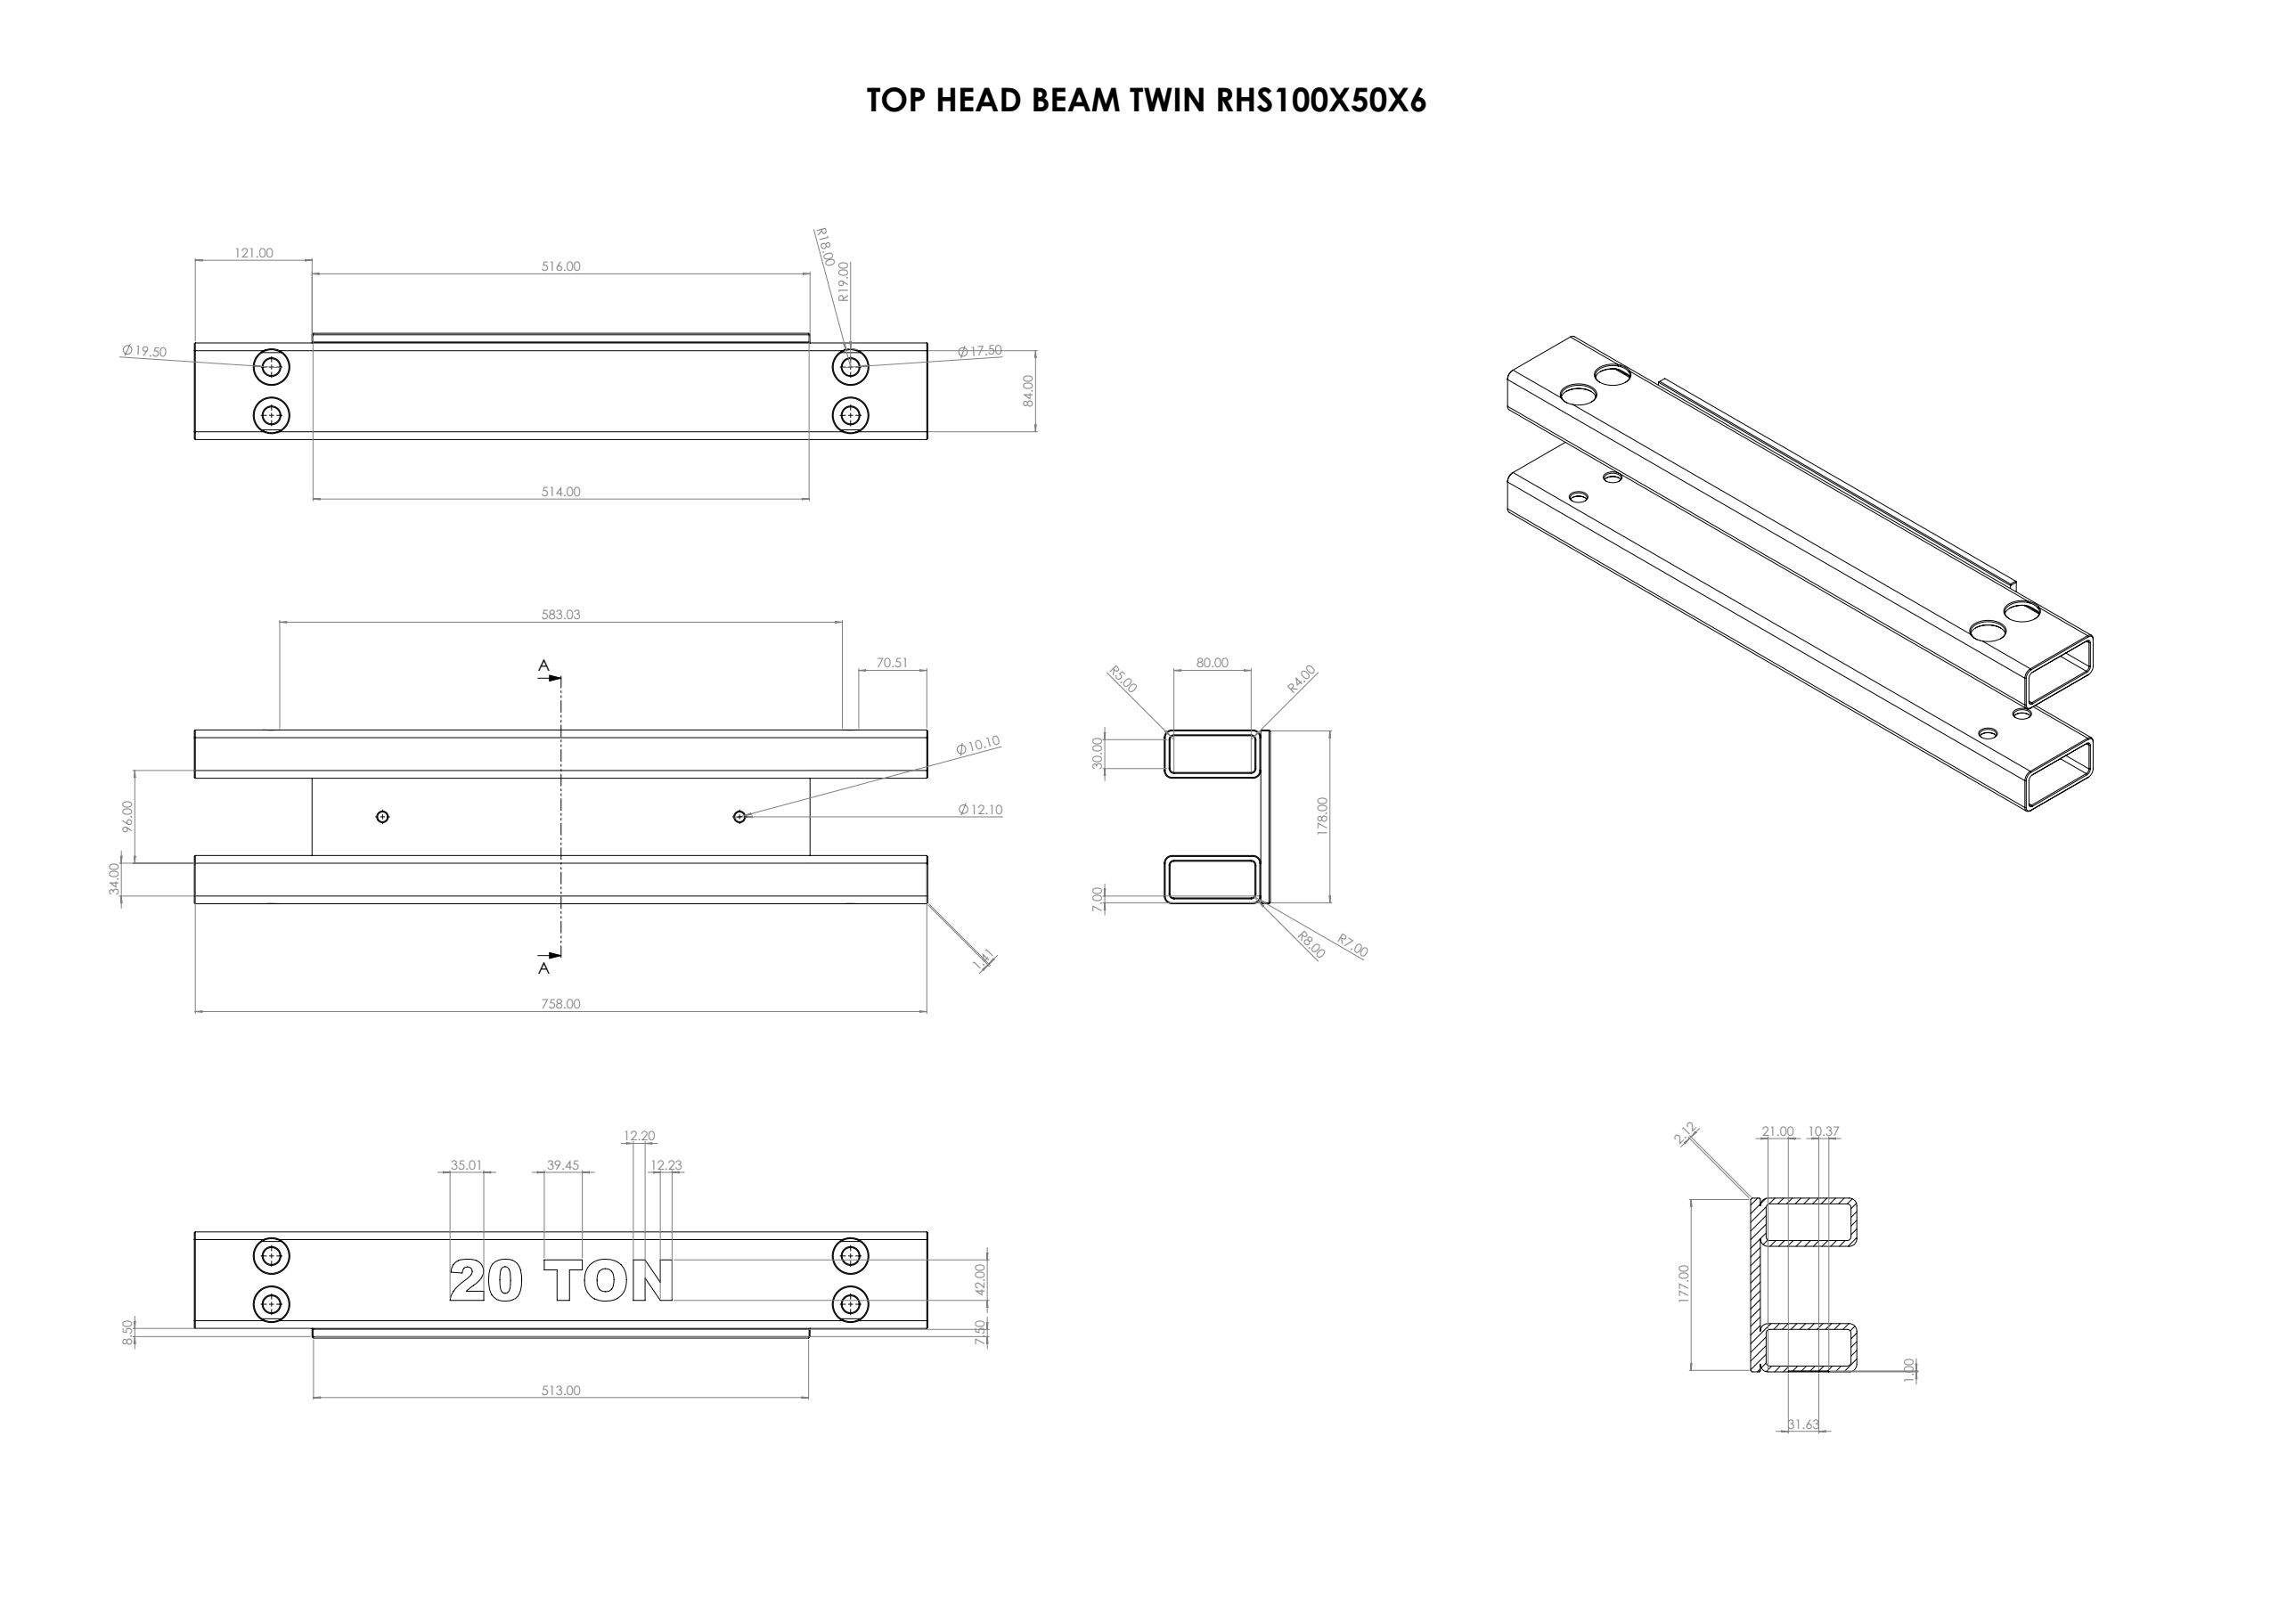
ISO-10303-21;
HEADER;
/* Generated by software containing ST-Developer
 * from STEP Tools, Inc. (www.steptools.com) 
 */

FILE_DESCRIPTION(
/* description */ (''),
/* implementation_level */ '2;1');

FILE_NAME(
/* name */ '02_Top_Head_Beam_Twin_RHS100x50x6.step',
/* time_stamp */ '2026-10-20T10:03:03-07:00',
/* author */ (''),
/* organization */ (''),
/* preprocessor_version */ 'ST-DEVELOPER v20.2',
/* originating_system */ 'Autodesk Translation Framework v15.15.0.0',
/* authorisation */ '');

FILE_SCHEMA (('AUTOMOTIVE_DESIGN { 1 0 10303 214 3 1 1 }'));
ENDSEC;

DATA;
#10=MECHANICAL_DESIGN_GEOMETRIC_PRESENTATION_REPRESENTATION('',(#439,#440,#441,#442,#443,#444,#445,#446,#447,#448,#449,#450,#451,#452,#453,#454,#455,#456,#457,#458,#459,#460,#461,#462,#463,#464,#465,#466,#467,#468,#469,#470,#471,#472,#473,#474,#475,#476,#477,#478,#479,#480,#481,#482,#483,#484,#485,#486,#487,#488,#489,#490,#491,#492,#493,#494,#495,#496,#497,#498,#499,#500,#501,#502,#503,#504,#505,#506,#507,#508,#509,#510,#511,#512,#513,#514,#515,#516,#517,#518,#519,#520,#521,#522,#523,#524),#71492);
#382=SHAPE_REPRESENTATION_RELATIONSHIP('SRR','None',#71603,#401);
#401=ADVANCED_BREP_SHAPE_REPRESENTATION('',(#420),#71473);
#420=MANIFOLD_SOLID_BREP('Top beam',#28459);
#439=STYLED_ITEM('',(#71873),#27095);
#440=STYLED_ITEM('',(#71873),#27096);
#441=STYLED_ITEM('',(#71873),#27097);
#442=STYLED_ITEM('',(#71873),#27098);
#443=STYLED_ITEM('',(#71873),#27099);
#444=STYLED_ITEM('',(#71873),#27100);
#445=STYLED_ITEM('',(#71873),#27101);
#446=STYLED_ITEM('',(#71873),#27102);
#447=STYLED_ITEM('',(#71873),#27103);
#448=STYLED_ITEM('',(#71873),#27104);
#449=STYLED_ITEM('',(#71873),#27105);
#450=STYLED_ITEM('',(#71873),#27106);
#451=STYLED_ITEM('',(#71873),#27107);
#452=STYLED_ITEM('',(#71873),#27108);
#453=STYLED_ITEM('',(#71873),#27109);
#454=STYLED_ITEM('',(#71873),#27110);
#455=STYLED_ITEM('',(#71873),#27111);
#456=STYLED_ITEM('',(#71873),#27112);
#457=STYLED_ITEM('',(#71873),#27113);
#458=STYLED_ITEM('',(#71873),#27114);
#459=STYLED_ITEM('',(#71873),#27115);
#460=STYLED_ITEM('',(#71873),#27116);
#461=STYLED_ITEM('',(#71873),#27117);
#462=STYLED_ITEM('',(#71873),#27118);
#463=STYLED_ITEM('',(#71873),#27119);
#464=STYLED_ITEM('',(#71873),#27120);
#465=STYLED_ITEM('',(#71873),#27121);
#466=STYLED_ITEM('',(#71873),#27122);
#467=STYLED_ITEM('',(#71873),#27123);
#468=STYLED_ITEM('',(#71873),#27124);
#469=STYLED_ITEM('',(#71873),#27125);
#470=STYLED_ITEM('',(#71873),#27126);
#471=STYLED_ITEM('',(#71873),#27127);
#472=STYLED_ITEM('',(#71873),#27128);
#473=STYLED_ITEM('',(#71873),#27129);
#474=STYLED_ITEM('',(#71873),#27130);
#475=STYLED_ITEM('',(#71873),#27131);
#476=STYLED_ITEM('',(#71873),#27132);
#477=STYLED_ITEM('',(#71873),#27133);
#478=STYLED_ITEM('',(#71873),#27134);
#479=STYLED_ITEM('',(#71873),#27135);
#480=STYLED_ITEM('',(#71873),#27136);
#481=STYLED_ITEM('',(#71873),#27137);
#482=STYLED_ITEM('',(#71873),#27138);
#483=STYLED_ITEM('',(#71873),#27139);
#484=STYLED_ITEM('',(#71873),#27140);
#485=STYLED_ITEM('',(#71873),#27141);
#486=STYLED_ITEM('',(#71873),#27142);
#487=STYLED_ITEM('',(#71873),#27143);
#488=STYLED_ITEM('',(#71873),#27144);
#489=STYLED_ITEM('',(#71873),#27145);
#490=STYLED_ITEM('',(#71873),#27146);
#491=STYLED_ITEM('',(#71873),#27147);
#492=STYLED_ITEM('',(#71873),#27148);
#493=STYLED_ITEM('',(#71873),#27149);
#494=STYLED_ITEM('',(#71873),#27150);
#495=STYLED_ITEM('',(#71873),#27151);
#496=STYLED_ITEM('',(#71873),#27152);
#497=STYLED_ITEM('',(#71873),#27153);
#498=STYLED_ITEM('',(#71873),#27154);
#499=STYLED_ITEM('',(#71873),#27155);
#500=STYLED_ITEM('',(#71873),#27156);
#501=STYLED_ITEM('',(#71873),#27157);
#502=STYLED_ITEM('',(#71873),#27158);
#503=STYLED_ITEM('',(#71873),#27159);
#504=STYLED_ITEM('',(#71873),#27160);
#505=STYLED_ITEM('',(#71873),#27161);
#506=STYLED_ITEM('',(#71873),#27162);
#507=STYLED_ITEM('',(#71873),#27163);
#508=STYLED_ITEM('',(#71873),#27164);
#509=STYLED_ITEM('',(#71873),#27165);
#510=STYLED_ITEM('',(#71873),#27166);
#511=STYLED_ITEM('',(#71873),#27167);
#512=STYLED_ITEM('',(#71873),#27168);
#513=STYLED_ITEM('',(#71873),#27169);
#514=STYLED_ITEM('',(#71873),#27170);
#515=STYLED_ITEM('',(#71873),#27171);
#516=STYLED_ITEM('',(#71873),#27172);
#517=STYLED_ITEM('',(#71873),#27173);
#518=STYLED_ITEM('',(#71873),#27174);
#519=STYLED_ITEM('',(#71873),#27175);
#520=STYLED_ITEM('',(#71873),#27176);
#521=STYLED_ITEM('',(#71873),#27177);
#522=STYLED_ITEM('',(#71873),#27178);
#523=STYLED_ITEM('',(#71873),#27179);
#524=STYLED_ITEM('',(#71873),#420);
#551=B_SPLINE_CURVE_WITH_KNOTS('',3,(#37939,#37940,#37941,#37942,#37943,
#37944,#37945,#37946,#37947),.UNSPECIFIED.,.F.,.F.,(4,2,1,1,1,4),(-2.76222327472562,
-2.70245118401238,-2.26839934091757,-2.05137341937016,-1.83434749782276,
-1.61732157627536),.UNSPECIFIED.);
#552=B_SPLINE_CURVE_WITH_KNOTS('',3,(#37950,#37951,#37952,#37953,#37954,
#37955,#37956,#37957,#37958),.UNSPECIFIED.,.F.,.F.,(4,1,1,1,2,4),(1.61732157627536,
1.83434749782276,2.05137341937016,2.26839934091757,2.70245118401238,2.76222327472562),
 .UNSPECIFIED.);
#553=B_SPLINE_CURVE_WITH_KNOTS('',3,(#37975,#37976,#37977,#37978),
 .UNSPECIFIED.,.F.,.F.,(4,4),(1.90569248523429,2.03375105473527),
 .UNSPECIFIED.);
#554=B_SPLINE_CURVE_WITH_KNOTS('',3,(#37979,#37980,#37981,#37982),
 .UNSPECIFIED.,.F.,.F.,(4,4),(-2.03375105473527,-1.90569248523429),
 .UNSPECIFIED.);
#555=B_SPLINE_CURVE_WITH_KNOTS('',3,(#37999,#38000,#38001,#38002),
 .UNSPECIFIED.,.F.,.F.,(4,4),(1.10784159885376,1.2359001683555),
 .UNSPECIFIED.);
#556=B_SPLINE_CURVE_WITH_KNOTS('',3,(#38003,#38004,#38005,#38006),
 .UNSPECIFIED.,.F.,.F.,(4,4),(-1.2359001683555,-1.10784159885376),
 .UNSPECIFIED.);
#557=B_SPLINE_CURVE_WITH_KNOTS('',3,(#38019,#38020,#38021,#38022),
 .UNSPECIFIED.,.F.,.F.,(4,4),(1.90569248523429,2.03375105473527),
 .UNSPECIFIED.);
#558=B_SPLINE_CURVE_WITH_KNOTS('',3,(#38024,#38025,#38026,#38027,#38028,
#38029,#38030,#38031,#38032,#38033),.UNSPECIFIED.,.F.,.F.,(4,2,1,1,1,1,
4),(-2.76222327472564,-2.70245118401238,-2.48542526246498,-2.26839934091757,
-2.05137341937017,-1.83434749782276,-1.61732157627536),.UNSPECIFIED.);
#559=B_SPLINE_CURVE_WITH_KNOTS('',3,(#38035,#38036,#38037,#38038),
 .UNSPECIFIED.,.F.,.F.,(4,4),(1.10784159885378,1.2359001683555),
 .UNSPECIFIED.);
#560=B_SPLINE_CURVE_WITH_KNOTS('',3,(#38046,#38047,#38048,#38049),
 .UNSPECIFIED.,.F.,.F.,(4,4),(2.15648187025205,2.23164162261786),
 .UNSPECIFIED.);
#561=B_SPLINE_CURVE_WITH_KNOTS('',3,(#38051,#38052,#38053,#38054,#38055,
#38056,#38057,#38058,#38059,#38060,#38061,#38062,#38063,#38064,#38065,#38066,
#38067,#38068,#38069,#38070,#38071,#38072,#38073,#38074,#38075,#38076,#38077,
#38078,#38079,#38080,#38081,#38082,#38083,#38084,#38085,#38086,#38087),
 .UNSPECIFIED.,.F.,.F.,(4,3,3,3,3,3,3,3,3,3,3,3,4),(0.754355313185428,0.781440569694549,
0.818270933113804,1.2600819055102,1.70189287790659,1.71022064144053,1.73520393204235,
1.80478675064372,1.8743695692451,1.92549026456033,1.97661095987556,2.5752615771494,
2.77481178290734),.UNSPECIFIED.);
#562=B_SPLINE_CURVE_WITH_KNOTS('',3,(#38089,#38090,#38091,#38092),
 .UNSPECIFIED.,.F.,.F.,(4,4),(0.90995103097194,0.98511078333776),
 .UNSPECIFIED.);
#563=B_SPLINE_CURVE_WITH_KNOTS('',3,(#38174,#38175,#38176,#38177),
 .UNSPECIFIED.,.F.,.F.,(4,4),(-1.2359001683555,-1.10784159885453),
 .UNSPECIFIED.);
#564=B_SPLINE_CURVE_WITH_KNOTS('',3,(#38179,#38180,#38181,#38182,#38183,
#38184,#38185,#38186,#38187,#38188),.UNSPECIFIED.,.F.,.F.,(4,2,1,1,2,4),
(-2.76222327472564,-2.70245118401238,-2.29230817720287,-2.08723667379812,
-1.67709366698862,-1.61732157627537),.UNSPECIFIED.);
#565=B_SPLINE_CURVE_WITH_KNOTS('',3,(#38190,#38191,#38192,#38193),
 .UNSPECIFIED.,.F.,.F.,(4,4),(-2.03375105473602,-1.9056924852343),
 .UNSPECIFIED.);
#566=B_SPLINE_CURVE_WITH_KNOTS('',3,(#38197,#38198,#38199,#38200),
 .UNSPECIFIED.,.F.,.F.,(4,4),(-1.2359001683555,-1.10784159885453),
 .UNSPECIFIED.);
#567=B_SPLINE_CURVE_WITH_KNOTS('',3,(#38202,#38203,#38204,#38205,#38206,
#38207,#38208,#38209,#38210,#38211,#38212),.UNSPECIFIED.,.F.,.F.,(4,2,1,
1,1,2,4),(-2.76222327472563,-2.70245118401238,-2.49737968060763,-2.39484392890525,
-2.08723667379813,-1.67709366698862,-1.61732157627537),.UNSPECIFIED.);
#568=B_SPLINE_CURVE_WITH_KNOTS('',3,(#38214,#38215,#38216,#38217),
 .UNSPECIFIED.,.F.,.F.,(4,4),(-2.03375105473601,-1.9056924852343),
 .UNSPECIFIED.);
#569=B_SPLINE_CURVE_WITH_KNOTS('',2,(#38285,#38286,#38287),
 .UNSPECIFIED.,.F.,.F.,(3,3),(0.,1.),.UNSPECIFIED.);
#570=B_SPLINE_CURVE_WITH_KNOTS('',2,(#38289,#38290,#38291),
 .UNSPECIFIED.,.F.,.F.,(3,3),(0.,1.),.UNSPECIFIED.);
#571=B_SPLINE_CURVE_WITH_KNOTS('',2,(#38293,#38294,#38295),
 .UNSPECIFIED.,.F.,.F.,(3,3),(0.,1.),.UNSPECIFIED.);
#572=B_SPLINE_CURVE_WITH_KNOTS('',2,(#38297,#38298,#38299),
 .UNSPECIFIED.,.F.,.F.,(3,3),(0.,1.),.UNSPECIFIED.);
#573=B_SPLINE_CURVE_WITH_KNOTS('',2,(#38301,#38302,#38303),
 .UNSPECIFIED.,.F.,.F.,(3,3),(0.,1.),.UNSPECIFIED.);
#574=B_SPLINE_CURVE_WITH_KNOTS('',2,(#38305,#38306,#38307),
 .UNSPECIFIED.,.F.,.F.,(3,3),(0.,1.),.UNSPECIFIED.);
#575=B_SPLINE_CURVE_WITH_KNOTS('',2,(#38309,#38310,#38311),
 .UNSPECIFIED.,.F.,.F.,(3,3),(0.,1.),.UNSPECIFIED.);
#576=B_SPLINE_CURVE_WITH_KNOTS('',2,(#38313,#38314,#38315),
 .UNSPECIFIED.,.F.,.F.,(3,3),(0.,1.),.UNSPECIFIED.);
#577=B_SPLINE_CURVE_WITH_KNOTS('',2,(#38317,#38318,#38319),
 .UNSPECIFIED.,.F.,.F.,(3,3),(0.,1.),.UNSPECIFIED.);
#578=B_SPLINE_CURVE_WITH_KNOTS('',2,(#38320,#38321,#38322),
 .UNSPECIFIED.,.F.,.F.,(3,3),(0.,1.),.UNSPECIFIED.);
#579=B_SPLINE_CURVE_WITH_KNOTS('',2,(#38341,#38342,#38343),
 .UNSPECIFIED.,.F.,.F.,(3,3),(0.,1.),.UNSPECIFIED.);
#580=B_SPLINE_CURVE_WITH_KNOTS('',2,(#38345,#38346,#38347),
 .UNSPECIFIED.,.F.,.F.,(3,3),(0.,1.),.UNSPECIFIED.);
#581=B_SPLINE_CURVE_WITH_KNOTS('',2,(#38349,#38350,#38351),
 .UNSPECIFIED.,.F.,.F.,(3,3),(0.,1.),.UNSPECIFIED.);
#582=B_SPLINE_CURVE_WITH_KNOTS('',2,(#38353,#38354,#38355),
 .UNSPECIFIED.,.F.,.F.,(3,3),(0.,1.),.UNSPECIFIED.);
#583=B_SPLINE_CURVE_WITH_KNOTS('',2,(#38357,#38358,#38359),
 .UNSPECIFIED.,.F.,.F.,(3,3),(0.,1.),.UNSPECIFIED.);
#584=B_SPLINE_CURVE_WITH_KNOTS('',2,(#38361,#38362,#38363),
 .UNSPECIFIED.,.F.,.F.,(3,3),(0.,1.),.UNSPECIFIED.);
#585=B_SPLINE_CURVE_WITH_KNOTS('',2,(#38365,#38366,#38367),
 .UNSPECIFIED.,.F.,.F.,(3,3),(0.,1.),.UNSPECIFIED.);
#586=B_SPLINE_CURVE_WITH_KNOTS('',2,(#38369,#38370,#38371),
 .UNSPECIFIED.,.F.,.F.,(3,3),(0.,1.),.UNSPECIFIED.);
#587=B_SPLINE_CURVE_WITH_KNOTS('',2,(#38373,#38374,#38375),
 .UNSPECIFIED.,.F.,.F.,(3,3),(0.,1.),.UNSPECIFIED.);
#588=B_SPLINE_CURVE_WITH_KNOTS('',2,(#38377,#38378,#38379),
 .UNSPECIFIED.,.F.,.F.,(3,3),(0.,1.),.UNSPECIFIED.);
#589=B_SPLINE_CURVE_WITH_KNOTS('',2,(#38381,#38382,#38383),
 .UNSPECIFIED.,.F.,.F.,(3,3),(0.,1.),.UNSPECIFIED.);
#590=B_SPLINE_CURVE_WITH_KNOTS('',2,(#38385,#38386,#38387),
 .UNSPECIFIED.,.F.,.F.,(3,3),(0.,1.),.UNSPECIFIED.);
#591=B_SPLINE_CURVE_WITH_KNOTS('',2,(#38388,#38389,#38390),
 .UNSPECIFIED.,.F.,.F.,(3,3),(0.,1.),.UNSPECIFIED.);
#592=B_SPLINE_CURVE_WITH_KNOTS('',2,(#38399,#38400,#38401),
 .UNSPECIFIED.,.F.,.F.,(3,3),(0.,1.),.UNSPECIFIED.);
#593=B_SPLINE_CURVE_WITH_KNOTS('',2,(#38403,#38404,#38405),
 .UNSPECIFIED.,.F.,.F.,(3,3),(0.,1.),.UNSPECIFIED.);
#594=B_SPLINE_CURVE_WITH_KNOTS('',2,(#38407,#38408,#38409),
 .UNSPECIFIED.,.F.,.F.,(3,3),(0.,1.),.UNSPECIFIED.);
#595=B_SPLINE_CURVE_WITH_KNOTS('',2,(#38411,#38412,#38413),
 .UNSPECIFIED.,.F.,.F.,(3,3),(0.,1.),.UNSPECIFIED.);
#596=B_SPLINE_CURVE_WITH_KNOTS('',2,(#38415,#38416,#38417),
 .UNSPECIFIED.,.F.,.F.,(3,3),(0.,1.),.UNSPECIFIED.);
#597=B_SPLINE_CURVE_WITH_KNOTS('',2,(#38419,#38420,#38421),
 .UNSPECIFIED.,.F.,.F.,(3,3),(0.,1.),.UNSPECIFIED.);
#598=B_SPLINE_CURVE_WITH_KNOTS('',2,(#38423,#38424,#38425),
 .UNSPECIFIED.,.F.,.F.,(3,3),(0.,1.),.UNSPECIFIED.);
#599=B_SPLINE_CURVE_WITH_KNOTS('',2,(#38427,#38428,#38429),
 .UNSPECIFIED.,.F.,.F.,(3,3),(0.,1.),.UNSPECIFIED.);
#600=B_SPLINE_CURVE_WITH_KNOTS('',2,(#38433,#38434,#38435),
 .UNSPECIFIED.,.F.,.F.,(3,3),(0.,1.),.UNSPECIFIED.);
#601=B_SPLINE_CURVE_WITH_KNOTS('',2,(#38437,#38438,#38439),
 .UNSPECIFIED.,.F.,.F.,(3,3),(0.,1.),.UNSPECIFIED.);
#602=B_SPLINE_CURVE_WITH_KNOTS('',2,(#38441,#38442,#38443),
 .UNSPECIFIED.,.F.,.F.,(3,3),(0.,1.),.UNSPECIFIED.);
#603=B_SPLINE_CURVE_WITH_KNOTS('',2,(#38445,#38446,#38447),
 .UNSPECIFIED.,.F.,.F.,(3,3),(0.,1.),.UNSPECIFIED.);
#604=B_SPLINE_CURVE_WITH_KNOTS('',2,(#38449,#38450,#38451),
 .UNSPECIFIED.,.F.,.F.,(3,3),(0.,1.),.UNSPECIFIED.);
#605=B_SPLINE_CURVE_WITH_KNOTS('',2,(#38453,#38454,#38455),
 .UNSPECIFIED.,.F.,.F.,(3,3),(0.,1.),.UNSPECIFIED.);
#606=B_SPLINE_CURVE_WITH_KNOTS('',2,(#38457,#38458,#38459),
 .UNSPECIFIED.,.F.,.F.,(3,3),(0.,1.),.UNSPECIFIED.);
#607=B_SPLINE_CURVE_WITH_KNOTS('',2,(#38461,#38462,#38463),
 .UNSPECIFIED.,.F.,.F.,(3,3),(0.,1.),.UNSPECIFIED.);
#608=B_SPLINE_CURVE_WITH_KNOTS('',2,(#38465,#38466,#38467),
 .UNSPECIFIED.,.F.,.F.,(3,3),(0.,1.),.UNSPECIFIED.);
#609=B_SPLINE_CURVE_WITH_KNOTS('',2,(#38468,#38469,#38470),
 .UNSPECIFIED.,.F.,.F.,(3,3),(0.,1.),.UNSPECIFIED.);
#610=B_SPLINE_CURVE_WITH_KNOTS('',3,(#38564,#38565,#38566,#38567,#38568,
#38569,#38570,#38571,#38572,#38573,#38574),.UNSPECIFIED.,.F.,.F.,(4,2,1,
1,1,2,4),(1.61732157627537,1.67709366698862,2.08723667379813,2.39484392890525,
2.49737968060763,2.70245118401238,2.76222327472563),.UNSPECIFIED.);
#611=B_SPLINE_CURVE_WITH_KNOTS('',3,(#38591,#38592,#38593,#38594),
 .UNSPECIFIED.,.F.,.F.,(4,4),(1.10784159885453,1.2359001683555),
 .UNSPECIFIED.);
#612=B_SPLINE_CURVE_WITH_KNOTS('',3,(#38611,#38612,#38613,#38614),
 .UNSPECIFIED.,.F.,.F.,(4,4),(1.9056924852343,2.03375105473601),
 .UNSPECIFIED.);
#613=B_SPLINE_CURVE_WITH_KNOTS('',3,(#38621,#38622,#38623,#38624),
 .UNSPECIFIED.,.F.,.F.,(4,4),(-0.985110783337743,-0.909951030971934),
 .UNSPECIFIED.);
#614=B_SPLINE_CURVE_WITH_KNOTS('',3,(#38626,#38627,#38628,#38629,#38630,
#38631,#38632,#38633,#38634,#38635,#38636,#38637,#38638,#38639,#38640,#38641,
#38642,#38643,#38644,#38645,#38646,#38647,#38648,#38649,#38650,#38651,#38652,
#38653,#38654,#38655,#38656),.UNSPECIFIED.,.F.,.F.,(4,3,3,3,3,3,3,3,3,3,
4),(0.754355313185451,0.781440569694569,0.818270933113807,1.42914691644436,
1.63277224422121,1.70189287790658,1.73520393204232,1.87436956924877,1.97661095987549,
2.57526157714938,2.77481178290734),.UNSPECIFIED.);
#615=B_SPLINE_CURVE_WITH_KNOTS('',3,(#38658,#38659,#38660,#38661),
 .UNSPECIFIED.,.F.,.F.,(4,4),(-2.23164162261785,-2.15648187025204),
 .UNSPECIFIED.);
#616=B_SPLINE_CURVE_WITH_KNOTS('',3,(#38715,#38716,#38717,#38718,#38719,
#38720,#38721,#38722,#38723,#38724),.UNSPECIFIED.,.F.,.F.,(4,1,1,1,1,2,
4),(1.61732157627536,1.83434749782276,2.05137341937017,2.26839934091757,
2.48542526246498,2.70245118401238,2.76222327472564),.UNSPECIFIED.);
#617=B_SPLINE_CURVE_WITH_KNOTS('',3,(#38741,#38742,#38743,#38744),
 .UNSPECIFIED.,.F.,.F.,(4,4),(-2.03375105473527,-1.90569248523429),
 .UNSPECIFIED.);
#618=B_SPLINE_CURVE_WITH_KNOTS('',3,(#38761,#38762,#38763,#38764),
 .UNSPECIFIED.,.F.,.F.,(4,4),(-1.2359001683555,-1.10784159885378),
 .UNSPECIFIED.);
#619=B_SPLINE_CURVE_WITH_KNOTS('',3,(#38771,#38772,#38773,#38774),
 .UNSPECIFIED.,.F.,.F.,(4,4),(2.15648187025205,2.23164162261786),
 .UNSPECIFIED.);
#620=B_SPLINE_CURVE_WITH_KNOTS('',3,(#38776,#38777,#38778,#38779,#38780,
#38781,#38782,#38783,#38784,#38785,#38786,#38787,#38788,#38789,#38790,#38791,
#38792,#38793,#38794,#38795,#38796,#38797,#38798,#38799,#38800,#38801,#38802,
#38803,#38804,#38805,#38806,#38807,#38808,#38809,#38810,#38811,#38812),
 .UNSPECIFIED.,.F.,.F.,(4,3,3,3,3,3,3,3,3,3,3,3,4),(0.75435531318544,0.781440569694525,
0.818270933113715,1.47797557423085,1.63277224422101,1.70189287790658,1.73520393204241,
1.87436956924587,1.97661095987572,2.10085602838433,2.43783390564597,2.60632284427679,
2.77481178290761),.UNSPECIFIED.);
#621=B_SPLINE_CURVE_WITH_KNOTS('',3,(#38814,#38815,#38816,#38817),
 .UNSPECIFIED.,.F.,.F.,(4,4),(0.90995103097194,0.985110783337756),
 .UNSPECIFIED.);
#622=B_SPLINE_CURVE_WITH_KNOTS('',3,(#38860,#38861,#38862,#38863),
 .UNSPECIFIED.,.F.,.F.,(4,4),(2.15648187025204,2.23164162261785),
 .UNSPECIFIED.);
#623=B_SPLINE_CURVE_WITH_KNOTS('',3,(#38865,#38866,#38867,#38868,#38869,
#38870,#38871,#38872,#38873,#38874),.UNSPECIFIED.,.F.,.F.,(4,3,3,4),(-1.16153810946438,
-0.819783369909235,-0.782081488746963,-0.754355313185429),.UNSPECIFIED.);
#624=B_SPLINE_CURVE_WITH_KNOTS('',3,(#38876,#38877,#38878,#38879,#38880,
#38881,#38882,#38883,#38884,#38885,#38886,#38887,#38888,#38889,#38890),
 .UNSPECIFIED.,.F.,.F.,(4,2,2,2,2,2,1,4),(-2.39250890756734,-2.0015894299973,
-1.89936032175267,-1.76021140268278,-1.72690435024433,-1.6577920201044,
-1.45419115408482,-1.17754443036118),.UNSPECIFIED.);
#625=B_SPLINE_CURVE_WITH_KNOTS('',3,(#38892,#38893,#38894,#38895,#38896),
 .UNSPECIFIED.,.F.,.F.,(4,1,4),(-2.79969436419745,-2.60016813064741,-2.39250890756734),
 .UNSPECIFIED.);
#626=B_SPLINE_CURVE_WITH_KNOTS('',3,(#38898,#38899,#38900,#38901),
 .UNSPECIFIED.,.F.,.F.,(4,4),(0.969091106047996,0.985110783337743),
 .UNSPECIFIED.);
#627=B_SPLINE_CURVE_WITH_KNOTS('',3,(#38903,#38904,#38905,#38906),
 .UNSPECIFIED.,.F.,.F.,(4,4),(0.909951030971922,0.969091106047996),
 .UNSPECIFIED.);
#628=B_SPLINE_CURVE_WITH_KNOTS('',3,(#38910,#38911,#38912,#38913),
 .UNSPECIFIED.,.F.,.F.,(4,4),(2.15648187025204,2.23164162261785),
 .UNSPECIFIED.);
#629=B_SPLINE_CURVE_WITH_KNOTS('',3,(#38915,#38916,#38917,#38918,#38919,
#38920,#38921,#38922,#38923,#38924),.UNSPECIFIED.,.F.,.F.,(4,3,3,4),(-1.16153810946442,
-0.8197833699093,-0.782081488746932,-0.754355313185416),.UNSPECIFIED.);
#630=B_SPLINE_CURVE_WITH_KNOTS('',3,(#38926,#38927,#38928,#38929,#38930,
#38931,#38932,#38933,#38934,#38935,#38936,#38937),.UNSPECIFIED.,.F.,.F.,
(4,2,2,2,1,1,4),(-2.39249743427155,-1.89936032175298,-1.76021140268327,
-1.72690435024575,-1.50602540169085,-1.28514645313595,-1.17750891267616),
 .UNSPECIFIED.);
#631=B_SPLINE_CURVE_WITH_KNOTS('',3,(#38939,#38940,#38941,#38942,#38943,
#38944),.UNSPECIFIED.,.F.,.F.,(4,1,1,4),(-2.79969436419745,-2.68715260889189,
-2.57461085358633,-2.39249743427155),.UNSPECIFIED.);
#632=B_SPLINE_CURVE_WITH_KNOTS('',3,(#38946,#38947,#38948,#38949),
 .UNSPECIFIED.,.F.,.F.,(4,4),(0.969091106053859,0.985110783337744),
 .UNSPECIFIED.);
#633=B_SPLINE_CURVE_WITH_KNOTS('',3,(#38951,#38952,#38953,#38954),
 .UNSPECIFIED.,.F.,.F.,(4,4),(0.909951030971929,0.969091106053859),
 .UNSPECIFIED.);
#634=B_SPLINE_CURVE_WITH_KNOTS('',3,(#39116,#39117,#39118,#39119),
 .UNSPECIFIED.,.F.,.F.,(4,4),(-0.98511078333776,-0.90995103097194),
 .UNSPECIFIED.);
#635=B_SPLINE_CURVE_WITH_KNOTS('',3,(#39121,#39122,#39123,#39124,#39125,
#39126,#39127,#39128,#39129,#39130),.UNSPECIFIED.,.F.,.F.,(4,3,3,4),(-1.16153810946441,
-0.819783369909218,-0.782081488746928,-0.754355313185416),.UNSPECIFIED.);
#636=B_SPLINE_CURVE_WITH_KNOTS('',3,(#39132,#39133,#39134,#39135,#39136,
#39137,#39138,#39139,#39140,#39141,#39142,#39143,#39144,#39145,#39146,#39147),
 .UNSPECIFIED.,.F.,.F.,(4,2,1,2,1,2,1,2,1,4),(-2.39254555505919,-2.00158942999727,
-1.95047487587308,-1.89936032174889,-1.82978586221579,-1.76021140268269,
-1.73523111335382,-1.7269043502442,-1.28514645313502,-1.17757064087985),
 .UNSPECIFIED.);
#637=B_SPLINE_CURVE_WITH_KNOTS('',3,(#39149,#39150,#39151,#39152,#39153),
 .UNSPECIFIED.,.F.,.F.,(4,1,4),(-2.79969436419745,-2.60016813064741,-2.39254555505919),
 .UNSPECIFIED.);
#638=B_SPLINE_CURVE_WITH_KNOTS('',3,(#39155,#39156,#39157,#39158),
 .UNSPECIFIED.,.F.,.F.,(4,4),(-2.17250154754389,-2.15648187025205),
 .UNSPECIFIED.);
#639=B_SPLINE_CURVE_WITH_KNOTS('',3,(#39159,#39160,#39161,#39162),
 .UNSPECIFIED.,.F.,.F.,(4,4),(-2.23164162261787,-2.17250154754389),
 .UNSPECIFIED.);
#640=B_SPLINE_CURVE_WITH_KNOTS('',3,(#39164,#39165,#39166,#39167),
 .UNSPECIFIED.,.F.,.F.,(4,4),(-0.985110783337756,-0.90995103097194),
 .UNSPECIFIED.);
#641=B_SPLINE_CURVE_WITH_KNOTS('',3,(#39169,#39170,#39171,#39172,#39173,
#39174,#39175,#39176,#39177,#39178),.UNSPECIFIED.,.F.,.F.,(4,3,3,4),(-1.16153810946433,
-0.819783369909133,-0.782081488746918,-0.754355313185436),.UNSPECIFIED.);
#642=B_SPLINE_CURVE_WITH_KNOTS('',3,(#39180,#39181,#39182,#39183,#39184,
#39185,#39186,#39187,#39188,#39189,#39190,#39191,#39192,#39193,#39194,#39195,
#39196,#39197),.UNSPECIFIED.,.F.,.F.,(4,2,2,2,2,2,2,2,4),(-2.39280165059179,
-2.12581957279538,-2.00158942999736,-1.89936032174962,-1.76021140268274,
-1.72690435024419,-1.65779202010408,-1.50301394602541,-1.17741711999687),
 .UNSPECIFIED.);
#643=B_SPLINE_CURVE_WITH_KNOTS('',3,(#39199,#39200,#39201,#39202,#39203,
#39204),.UNSPECIFIED.,.F.,.F.,(4,1,1,4),(-2.79969436419745,-2.63122566634693,
-2.46275696849641,-2.39280165059179),.UNSPECIFIED.);
#644=B_SPLINE_CURVE_WITH_KNOTS('',3,(#39206,#39207,#39208,#39209),
 .UNSPECIFIED.,.F.,.F.,(4,4),(-2.17250154754018,-2.15648187025205),
 .UNSPECIFIED.);
#645=B_SPLINE_CURVE_WITH_KNOTS('',3,(#39210,#39211,#39212,#39213),
 .UNSPECIFIED.,.F.,.F.,(4,4),(-2.23164162261787,-2.17250154754018),
 .UNSPECIFIED.);
#646=B_SPLINE_CURVE_WITH_KNOTS('',3,(#39520,#39521,#39522,#39523,#39524,
#39525,#39526,#39527,#39528,#39529),.UNSPECIFIED.,.F.,.F.,(4,2,1,1,2,4),
(1.61732157627537,1.67709366698862,2.08723667379812,2.29230817720287,2.70245118401238,
2.76222327472564),.UNSPECIFIED.);
#647=B_SPLINE_CURVE_WITH_KNOTS('',3,(#39546,#39547,#39548,#39549),
 .UNSPECIFIED.,.F.,.F.,(4,4),(1.10784159885453,1.2359001683555),
 .UNSPECIFIED.);
#648=B_SPLINE_CURVE_WITH_KNOTS('',3,(#39566,#39567,#39568,#39569),
 .UNSPECIFIED.,.F.,.F.,(4,4),(1.9056924852343,2.03375105473602),
 .UNSPECIFIED.);
#649=B_SPLINE_CURVE_WITH_KNOTS('',3,(#39576,#39577,#39578,#39579),
 .UNSPECIFIED.,.F.,.F.,(4,4),(-0.985110783337744,-0.909951030971936),
 .UNSPECIFIED.);
#650=B_SPLINE_CURVE_WITH_KNOTS('',3,(#39581,#39582,#39583,#39584,#39585,
#39586,#39587,#39588,#39589,#39590,#39591,#39592,#39593,#39594,#39595,#39596,
#39597,#39598,#39599,#39600,#39601,#39602,#39603,#39604,#39605,#39606,#39607,
#39608,#39609,#39610,#39611),.UNSPECIFIED.,.F.,.F.,(4,3,3,3,3,3,3,3,3,3,
4),(0.754355313185423,0.781440569694544,0.818270933113877,1.26008190551097,
1.48098739170952,1.70189287790806,1.73520393204287,1.87436956924915,2.5497012294929,
2.66225650620019,2.77481178290748),.UNSPECIFIED.);
#651=B_SPLINE_CURVE_WITH_KNOTS('',3,(#39613,#39614,#39615,#39616),
 .UNSPECIFIED.,.F.,.F.,(4,4),(-2.23164162261785,-2.15648187025204),
 .UNSPECIFIED.);
#652=B_SPLINE_CURVE_WITH_KNOTS('',3,(#39787,#39788,#39789,#39790),
 .UNSPECIFIED.,.F.,.F.,(4,4),(1.90569248523429,2.03375105473527),
 .UNSPECIFIED.);
#653=B_SPLINE_CURVE_WITH_KNOTS('',3,(#39792,#39793,#39794,#39795,#39796,
#39797,#39798,#39799,#39800,#39801),.UNSPECIFIED.,.F.,.F.,(4,2,1,1,2,4),
(-2.76222327472563,-2.70245118401238,-2.29230817720288,-2.08723667379812,
-1.67709366698862,-1.61732157627537),.UNSPECIFIED.);
#654=B_SPLINE_CURVE_WITH_KNOTS('',3,(#39803,#39804,#39805,#39806),
 .UNSPECIFIED.,.F.,.F.,(4,4),(1.10784159885378,1.2359001683555),
 .UNSPECIFIED.);
#655=B_SPLINE_CURVE_WITH_KNOTS('',3,(#39810,#39811,#39812,#39813),
 .UNSPECIFIED.,.F.,.F.,(4,4),(1.90569248523429,2.03375105473527),
 .UNSPECIFIED.);
#656=B_SPLINE_CURVE_WITH_KNOTS('',3,(#39815,#39816,#39817,#39818,#39819,
#39820,#39821,#39822,#39823,#39824),.UNSPECIFIED.,.F.,.F.,(4,2,1,1,2,4),
(-2.76222327472562,-2.70245118401238,-2.29230817720287,-2.08723667379812,
-1.67709366698862,-1.61732157627537),.UNSPECIFIED.);
#657=B_SPLINE_CURVE_WITH_KNOTS('',3,(#39826,#39827,#39828,#39829),
 .UNSPECIFIED.,.F.,.F.,(4,4),(1.10784159885377,1.23590016835549),
 .UNSPECIFIED.);
#658=B_SPLINE_CURVE_WITH_KNOTS('',3,(#39900,#39901,#39902,#39903),
 .UNSPECIFIED.,.F.,.F.,(4,4),(-1.23590016835551,-1.10784159885453),
 .UNSPECIFIED.);
#659=B_SPLINE_CURVE_WITH_KNOTS('',3,(#39905,#39906,#39907,#39908,#39909,
#39910,#39911,#39912,#39913,#39914),.UNSPECIFIED.,.F.,.F.,(4,2,1,1,2,4),
(-2.76222327472564,-2.70245118401238,-2.29230817720287,-2.08723667379812,
-1.67709366698862,-1.61732157627537),.UNSPECIFIED.);
#660=B_SPLINE_CURVE_WITH_KNOTS('',3,(#39916,#39917,#39918,#39919),
 .UNSPECIFIED.,.F.,.F.,(4,4),(-2.03375105473599,-1.9056924852343),
 .UNSPECIFIED.);
#661=B_SPLINE_CURVE_WITH_KNOTS('',3,(#39923,#39924,#39925,#39926),
 .UNSPECIFIED.,.F.,.F.,(4,4),(-1.2359001683555,-1.10784159885453),
 .UNSPECIFIED.);
#662=B_SPLINE_CURVE_WITH_KNOTS('',3,(#39928,#39929,#39930,#39931,#39932,
#39933,#39934,#39935,#39936,#39937,#39938),.UNSPECIFIED.,.F.,.F.,(4,2,1,
1,1,2,4),(-2.76222327472563,-2.70245118401238,-2.49737968060763,-2.39484392890525,
-2.08723667379813,-1.67709366698862,-1.61732157627537),.UNSPECIFIED.);
#663=B_SPLINE_CURVE_WITH_KNOTS('',3,(#39940,#39941,#39942,#39943),
 .UNSPECIFIED.,.F.,.F.,(4,4),(-2.03375105473601,-1.9056924852343),
 .UNSPECIFIED.);
#664=B_SPLINE_CURVE_WITH_KNOTS('',3,(#40011,#40012,#40013,#40014,#40015,
#40016,#40017,#40018,#40019,#40020),.UNSPECIFIED.,.F.,.F.,(4,2,1,1,2,4),
(1.61732157627537,1.67709366698862,2.08723667379812,2.29230817720287,2.70245118401238,
2.76222327472564),.UNSPECIFIED.);
#665=B_SPLINE_CURVE_WITH_KNOTS('',3,(#40045,#40046,#40047,#40048),
 .UNSPECIFIED.,.F.,.F.,(4,4),(1.9056924852343,2.03375105473599),
 .UNSPECIFIED.);
#666=B_SPLINE_CURVE_WITH_KNOTS('',3,(#40065,#40066,#40067,#40068),
 .UNSPECIFIED.,.F.,.F.,(4,4),(1.10784159885453,1.23590016835551),
 .UNSPECIFIED.);
#667=B_SPLINE_CURVE_WITH_KNOTS('',3,(#40075,#40076,#40077,#40078),
 .UNSPECIFIED.,.F.,.F.,(4,4),(-0.985110783337744,-0.909951030971936),
 .UNSPECIFIED.);
#668=B_SPLINE_CURVE_WITH_KNOTS('',3,(#40080,#40081,#40082,#40083,#40084,
#40085,#40086,#40087,#40088,#40089,#40090,#40091,#40092,#40093,#40094,#40095,
#40096,#40097,#40098,#40099,#40100,#40101,#40102,#40103,#40104,#40105,#40106,
#40107,#40108,#40109,#40110,#40111,#40112,#40113),.UNSPECIFIED.,.F.,.F.,
(4,3,3,3,3,3,3,3,3,3,3,4),(0.754355313185457,0.781440569694525,0.818270933113784,
1.26008190551044,1.48098739170876,1.70189287790709,1.73520393204254,1.80044174678674,
1.87436956924505,2.54970122949192,2.66225650619973,2.77481178290754),
 .UNSPECIFIED.);
#669=B_SPLINE_CURVE_WITH_KNOTS('',3,(#40115,#40116,#40117,#40118),
 .UNSPECIFIED.,.F.,.F.,(4,4),(-2.23164162261785,-2.15648187025204),
 .UNSPECIFIED.);
#670=B_SPLINE_CURVE_WITH_KNOTS('',3,(#40161,#40162,#40163,#40164),
 .UNSPECIFIED.,.F.,.F.,(4,4),(-0.985110783337753,-0.90995103097194),
 .UNSPECIFIED.);
#671=B_SPLINE_CURVE_WITH_KNOTS('',3,(#40166,#40167,#40168,#40169,#40170,
#40171,#40172,#40173,#40174,#40175),.UNSPECIFIED.,.F.,.F.,(4,3,3,4),(-1.16153810946444,
-0.819783369909333,-0.782081488746978,-0.754355313185483),.UNSPECIFIED.);
#672=B_SPLINE_CURVE_WITH_KNOTS('',3,(#40177,#40178,#40179,#40180,#40181,
#40182,#40183,#40184,#40185,#40186,#40187,#40188,#40189,#40190),
 .UNSPECIFIED.,.F.,.F.,(4,2,2,2,2,2,4),(-2.39249786125564,-1.89936032174935,
-1.8254413803293,-1.76021140268281,-1.72690435024458,-1.65779202010542,
-1.17747397511189),.UNSPECIFIED.);
#673=B_SPLINE_CURVE_WITH_KNOTS('',3,(#40192,#40193,#40194,#40195,#40196,
#40197),.UNSPECIFIED.,.F.,.F.,(4,1,1,4),(-2.79969436419745,-2.68715260889144,
-2.57461085358543,-2.39249786125564),.UNSPECIFIED.);
#674=B_SPLINE_CURVE_WITH_KNOTS('',3,(#40199,#40200,#40201,#40202),
 .UNSPECIFIED.,.F.,.F.,(4,4),(-2.23164162261786,-2.15648187025205),
 .UNSPECIFIED.);
#675=B_SPLINE_CURVE_WITH_KNOTS('',3,(#40206,#40207,#40208,#40209),
 .UNSPECIFIED.,.F.,.F.,(4,4),(-0.985110783337756,-0.90995103097194),
 .UNSPECIFIED.);
#676=B_SPLINE_CURVE_WITH_KNOTS('',3,(#40211,#40212,#40213,#40214,#40215,
#40216,#40217,#40218,#40219,#40220),.UNSPECIFIED.,.F.,.F.,(4,3,3,4),(-1.16153810946435,
-0.819783369909053,-0.782081488746808,-0.754355313185456),.UNSPECIFIED.);
#677=B_SPLINE_CURVE_WITH_KNOTS('',3,(#40222,#40223,#40224,#40225,#40226,
#40227,#40228,#40229,#40230,#40231,#40232,#40233,#40234,#40235,#40236),
 .UNSPECIFIED.,.F.,.F.,(4,2,2,2,2,2,1,4),(-2.39250890756776,-2.00158942999731,
-1.89936032174878,-1.76021140268269,-1.72690435024413,-1.65779202010392,
-1.45419115408438,-1.17754443036329),.UNSPECIFIED.);
#678=B_SPLINE_CURVE_WITH_KNOTS('',3,(#40238,#40239,#40240,#40241,#40242),
 .UNSPECIFIED.,.F.,.F.,(4,1,4),(-2.79969436419747,-2.60016813064743,-2.39250890756776),
 .UNSPECIFIED.);
#679=B_SPLINE_CURVE_WITH_KNOTS('',3,(#40244,#40245,#40246,#40247),
 .UNSPECIFIED.,.F.,.F.,(4,4),(-2.17250154753575,-2.15648187025205),
 .UNSPECIFIED.);
#680=B_SPLINE_CURVE_WITH_KNOTS('',3,(#40249,#40250,#40251,#40252),
 .UNSPECIFIED.,.F.,.F.,(4,4),(-2.23164162261787,-2.17250154753575),
 .UNSPECIFIED.);
#681=B_SPLINE_CURVE_WITH_KNOTS('',3,(#40297,#40298,#40299,#40300),
 .UNSPECIFIED.,.F.,.F.,(4,4),(2.15648187025204,2.23164162261785),
 .UNSPECIFIED.);
#682=B_SPLINE_CURVE_WITH_KNOTS('',3,(#40302,#40303,#40304,#40305,#40306,
#40307,#40308,#40309,#40310,#40311),.UNSPECIFIED.,.F.,.F.,(4,3,3,4),(-1.1615381094643,
-0.819783369909086,-0.782081488746884,-0.754355313185452),.UNSPECIFIED.);
#683=B_SPLINE_CURVE_WITH_KNOTS('',3,(#40313,#40314,#40315,#40316,#40317,
#40318,#40319,#40320,#40321,#40322,#40323,#40324,#40325,#40326,#40327,#40328),
 .UNSPECIFIED.,.F.,.F.,(4,2,2,2,2,2,2,4),(-2.39249643071187,-2.00158942999732,
-1.89936032174887,-1.82544138032896,-1.76021140268264,-1.72690435024399,
-1.65779202010374,-1.1774981323703),.UNSPECIFIED.);
#684=B_SPLINE_CURVE_WITH_KNOTS('',3,(#40330,#40331,#40332,#40333,#40334),
 .UNSPECIFIED.,.F.,.F.,(4,1,4),(-2.79969436419746,-2.60016813064742,-2.39249643071187),
 .UNSPECIFIED.);
#685=B_SPLINE_CURVE_WITH_KNOTS('',3,(#40335,#40336,#40337,#40338),
 .UNSPECIFIED.,.F.,.F.,(4,4),(0.90995103097193,0.985110783337743),
 .UNSPECIFIED.);
#686=B_SPLINE_CURVE_WITH_KNOTS('',3,(#40340,#40341,#40342,#40343),
 .UNSPECIFIED.,.F.,.F.,(4,4),(2.15648187025204,2.23164162261785),
 .UNSPECIFIED.);
#687=B_SPLINE_CURVE_WITH_KNOTS('',3,(#40345,#40346,#40347,#40348,#40349,
#40350,#40351,#40352,#40353,#40354),.UNSPECIFIED.,.F.,.F.,(4,3,3,4),(-1.16153810946437,
-0.819783369909201,-0.782081488746912,-0.754355313185438),.UNSPECIFIED.);
#688=B_SPLINE_CURVE_WITH_KNOTS('',3,(#40356,#40357,#40358,#40359,#40360,
#40361,#40362,#40363,#40364,#40365,#40366,#40367,#40368,#40369),
 .UNSPECIFIED.,.F.,.F.,(4,2,2,2,2,1,1,4),(-2.39247844687041,-1.89936032174889,
-1.82544138032945,-1.76021140268296,-1.7269043502448,-1.50602540169013,
-1.28514645313547,-1.17750545093659),.UNSPECIFIED.);
#689=B_SPLINE_CURVE_WITH_KNOTS('',3,(#40371,#40372,#40373,#40374,#40375,
#40376),.UNSPECIFIED.,.F.,.F.,(4,1,1,4),(-2.79969436419745,-2.68715260889138,
-2.57461085358531,-2.39247844687041),.UNSPECIFIED.);
#690=B_SPLINE_CURVE_WITH_KNOTS('',3,(#40378,#40379,#40380,#40381),
 .UNSPECIFIED.,.F.,.F.,(4,4),(0.969091106047469,0.985110783337744),
 .UNSPECIFIED.);
#691=B_SPLINE_CURVE_WITH_KNOTS('',3,(#40382,#40383,#40384,#40385),
 .UNSPECIFIED.,.F.,.F.,(4,4),(0.909951030971929,0.969091106047469),
 .UNSPECIFIED.);
#692=B_SPLINE_CURVE_WITH_KNOTS('',3,(#40555,#40556,#40557,#40558,#40559,
#40560,#40561,#40562,#40563,#40564),.UNSPECIFIED.,.F.,.F.,(4,2,1,1,2,4),
(1.61732157627537,1.67709366698862,2.08723667379812,2.29230817720288,2.70245118401238,
2.76222327472563),.UNSPECIFIED.);
#693=B_SPLINE_CURVE_WITH_KNOTS('',3,(#40581,#40582,#40583,#40584),
 .UNSPECIFIED.,.F.,.F.,(4,4),(-2.03375105473527,-1.90569248523429),
 .UNSPECIFIED.);
#694=B_SPLINE_CURVE_WITH_KNOTS('',3,(#40601,#40602,#40603,#40604),
 .UNSPECIFIED.,.F.,.F.,(4,4),(-1.2359001683555,-1.10784159885378),
 .UNSPECIFIED.);
#695=B_SPLINE_CURVE_WITH_KNOTS('',3,(#40611,#40612,#40613,#40614),
 .UNSPECIFIED.,.F.,.F.,(4,4),(2.15648187025205,2.23164162261786),
 .UNSPECIFIED.);
#696=B_SPLINE_CURVE_WITH_KNOTS('',3,(#40616,#40617,#40618,#40619,#40620,
#40621,#40622,#40623,#40624,#40625,#40626,#40627,#40628,#40629,#40630,#40631,
#40632,#40633,#40634,#40635,#40636,#40637,#40638,#40639,#40640,#40641,#40642,
#40643,#40644,#40645,#40646),.UNSPECIFIED.,.F.,.F.,(4,3,3,3,3,3,3,3,3,3,
4),(0.754355313185418,0.781440569694357,0.818270933113567,1.4291469164439,
1.63277224422068,1.70189287790631,1.73520393204215,1.87436956924478,1.97661095987539,
2.57526157714918,2.77481178290704),.UNSPECIFIED.);
#697=B_SPLINE_CURVE_WITH_KNOTS('',3,(#40648,#40649,#40650,#40651),
 .UNSPECIFIED.,.F.,.F.,(4,4),(0.90995103097194,0.985110783337756),
 .UNSPECIFIED.);
#698=B_SPLINE_CURVE_WITH_KNOTS('',3,(#40818,#40819,#40820,#40821,#40822,
#40823,#40824,#40825,#40826,#40827,#40828),.UNSPECIFIED.,.F.,.F.,(4,2,1,
1,1,2,4),(1.61732157627537,1.67709366698862,2.08723667379813,2.39484392890525,
2.49737968060763,2.70245118401238,2.76222327472563),.UNSPECIFIED.);
#699=B_SPLINE_CURVE_WITH_KNOTS('',3,(#40853,#40854,#40855,#40856),
 .UNSPECIFIED.,.F.,.F.,(4,4),(1.9056924852343,2.03375105473601),
 .UNSPECIFIED.);
#700=B_SPLINE_CURVE_WITH_KNOTS('',3,(#40873,#40874,#40875,#40876),
 .UNSPECIFIED.,.F.,.F.,(4,4),(1.10784159885453,1.2359001683555),
 .UNSPECIFIED.);
#701=B_SPLINE_CURVE_WITH_KNOTS('',3,(#40883,#40884,#40885,#40886),
 .UNSPECIFIED.,.F.,.F.,(4,4),(-0.985110783337743,-0.909951030971934),
 .UNSPECIFIED.);
#702=B_SPLINE_CURVE_WITH_KNOTS('',3,(#40888,#40889,#40890,#40891,#40892,
#40893,#40894,#40895,#40896,#40897,#40898,#40899,#40900,#40901,#40902,#40903,
#40904,#40905,#40906,#40907,#40908,#40909,#40910,#40911,#40912,#40913,#40914,
#40915,#40916,#40917,#40918),.UNSPECIFIED.,.F.,.F.,(4,3,3,3,3,3,3,3,3,3,
4),(0.754355313185433,0.781440569694449,0.818270933113629,1.63277224422067,
1.70189287790637,1.7352039320423,1.80044174678633,1.87436956924509,1.97661095987564,
2.57526157714951,2.77481178290747),.UNSPECIFIED.);
#703=B_SPLINE_CURVE_WITH_KNOTS('',3,(#40920,#40921,#40922,#40923),
 .UNSPECIFIED.,.F.,.F.,(4,4),(-2.23164162261785,-2.15648187025204),
 .UNSPECIFIED.);
#704=B_SPLINE_CURVE_WITH_KNOTS('',3,(#41098,#41099,#41100,#41101,#41102,
#41103,#41104,#41105,#41106,#41107),.UNSPECIFIED.,.F.,.F.,(4,2,1,1,2,4),
(1.61732157627537,1.67709366698862,2.08723667379812,2.29230817720287,2.70245118401238,
2.76222327472562),.UNSPECIFIED.);
#705=B_SPLINE_CURVE_WITH_KNOTS('',3,(#41124,#41125,#41126,#41127),
 .UNSPECIFIED.,.F.,.F.,(4,4),(-2.03375105473527,-1.90569248523429),
 .UNSPECIFIED.);
#706=B_SPLINE_CURVE_WITH_KNOTS('',3,(#41144,#41145,#41146,#41147),
 .UNSPECIFIED.,.F.,.F.,(4,4),(-1.23590016835549,-1.10784159885377),
 .UNSPECIFIED.);
#707=B_SPLINE_CURVE_WITH_KNOTS('',3,(#41154,#41155,#41156,#41157),
 .UNSPECIFIED.,.F.,.F.,(4,4),(2.15648187025205,2.23164162261786),
 .UNSPECIFIED.);
#708=B_SPLINE_CURVE_WITH_KNOTS('',3,(#41159,#41160,#41161,#41162,#41163,
#41164,#41165,#41166,#41167,#41168,#41169,#41170,#41171,#41172,#41173,#41174,
#41175,#41176,#41177,#41178,#41179,#41180,#41181,#41182,#41183,#41184,#41185,
#41186,#41187,#41188,#41189),.UNSPECIFIED.,.F.,.F.,(4,3,3,3,3,3,3,3,3,3,
4),(0.754355313185446,0.781440569694518,0.818270933113847,1.6327722442224,
1.701892877907,1.73520393204251,1.8004417467867,1.87436956924561,2.54970122949198,
2.6622565061997,2.77481178290743),.UNSPECIFIED.);
#709=B_SPLINE_CURVE_WITH_KNOTS('',3,(#41191,#41192,#41193,#41194),
 .UNSPECIFIED.,.F.,.F.,(4,4),(0.90995103097194,0.985110783337753),
 .UNSPECIFIED.);
#710=B_SPLINE_CURVE_WITH_KNOTS('',2,(#41352,#41353,#41354),
 .UNSPECIFIED.,.F.,.F.,(3,3),(0.,1.),.UNSPECIFIED.);
#711=B_SPLINE_CURVE_WITH_KNOTS('',2,(#41358,#41359,#41360),
 .UNSPECIFIED.,.F.,.F.,(3,3),(0.,1.),.UNSPECIFIED.);
#712=B_SPLINE_CURVE_WITH_KNOTS('',2,(#41369,#41370,#41371),
 .UNSPECIFIED.,.F.,.F.,(3,3),(0.,1.),.UNSPECIFIED.);
#713=B_SPLINE_CURVE_WITH_KNOTS('',2,(#41374,#41375,#41376),
 .UNSPECIFIED.,.F.,.F.,(3,3),(0.,1.),.UNSPECIFIED.);
#714=B_SPLINE_CURVE_WITH_KNOTS('',2,(#41384,#41385,#41386),
 .UNSPECIFIED.,.F.,.F.,(3,3),(0.,1.),.UNSPECIFIED.);
#715=B_SPLINE_CURVE_WITH_KNOTS('',2,(#41389,#41390,#41391),
 .UNSPECIFIED.,.F.,.F.,(3,3),(0.,1.),.UNSPECIFIED.);
#716=B_SPLINE_CURVE_WITH_KNOTS('',2,(#41399,#41400,#41401),
 .UNSPECIFIED.,.F.,.F.,(3,3),(0.,1.),.UNSPECIFIED.);
#717=B_SPLINE_CURVE_WITH_KNOTS('',2,(#41404,#41405,#41406),
 .UNSPECIFIED.,.F.,.F.,(3,3),(0.,1.),.UNSPECIFIED.);
#718=B_SPLINE_CURVE_WITH_KNOTS('',2,(#41414,#41415,#41416),
 .UNSPECIFIED.,.F.,.F.,(3,3),(0.,1.),.UNSPECIFIED.);
#719=B_SPLINE_CURVE_WITH_KNOTS('',2,(#41419,#41420,#41421),
 .UNSPECIFIED.,.F.,.F.,(3,3),(0.,1.),.UNSPECIFIED.);
#720=B_SPLINE_CURVE_WITH_KNOTS('',2,(#41429,#41430,#41431),
 .UNSPECIFIED.,.F.,.F.,(3,3),(0.,1.),.UNSPECIFIED.);
#721=B_SPLINE_CURVE_WITH_KNOTS('',2,(#41434,#41435,#41436),
 .UNSPECIFIED.,.F.,.F.,(3,3),(0.,1.),.UNSPECIFIED.);
#722=B_SPLINE_CURVE_WITH_KNOTS('',2,(#41444,#41445,#41446),
 .UNSPECIFIED.,.F.,.F.,(3,3),(0.,1.),.UNSPECIFIED.);
#723=B_SPLINE_CURVE_WITH_KNOTS('',2,(#41449,#41450,#41451),
 .UNSPECIFIED.,.F.,.F.,(3,3),(0.,1.),.UNSPECIFIED.);
#724=B_SPLINE_CURVE_WITH_KNOTS('',2,(#41458,#41459,#41460),
 .UNSPECIFIED.,.F.,.F.,(3,3),(0.,1.),.UNSPECIFIED.);
#725=B_SPLINE_CURVE_WITH_KNOTS('',2,(#41461,#41462,#41463),
 .UNSPECIFIED.,.F.,.F.,(3,3),(0.,1.),.UNSPECIFIED.);
#726=B_SPLINE_CURVE_WITH_KNOTS('',2,(#41473,#41474,#41475),
 .UNSPECIFIED.,.F.,.F.,(3,3),(0.,1.),.UNSPECIFIED.);
#727=B_SPLINE_CURVE_WITH_KNOTS('',2,(#41485,#41486,#41487),
 .UNSPECIFIED.,.F.,.F.,(3,3),(0.,1.),.UNSPECIFIED.);
#728=B_SPLINE_CURVE_WITH_KNOTS('',2,(#41496,#41497,#41498),
 .UNSPECIFIED.,.F.,.F.,(3,3),(0.,1.),.UNSPECIFIED.);
#729=B_SPLINE_CURVE_WITH_KNOTS('',2,(#41507,#41508,#41509),
 .UNSPECIFIED.,.F.,.F.,(3,3),(0.,1.),.UNSPECIFIED.);
#730=B_SPLINE_CURVE_WITH_KNOTS('',2,(#41518,#41519,#41520),
 .UNSPECIFIED.,.F.,.F.,(3,3),(0.,1.),.UNSPECIFIED.);
#731=B_SPLINE_CURVE_WITH_KNOTS('',2,(#41529,#41530,#41531),
 .UNSPECIFIED.,.F.,.F.,(3,3),(0.,1.),.UNSPECIFIED.);
#732=B_SPLINE_CURVE_WITH_KNOTS('',2,(#41540,#41541,#41542),
 .UNSPECIFIED.,.F.,.F.,(3,3),(0.,1.),.UNSPECIFIED.);
#733=B_SPLINE_CURVE_WITH_KNOTS('',2,(#41551,#41552,#41553),
 .UNSPECIFIED.,.F.,.F.,(3,3),(0.,1.),.UNSPECIFIED.);
#734=B_SPLINE_CURVE_WITH_KNOTS('',2,(#41562,#41563,#41564),
 .UNSPECIFIED.,.F.,.F.,(3,3),(0.,1.),.UNSPECIFIED.);
#735=B_SPLINE_CURVE_WITH_KNOTS('',2,(#41571,#41572,#41573),
 .UNSPECIFIED.,.F.,.F.,(3,3),(0.,1.),.UNSPECIFIED.);
#736=B_SPLINE_CURVE_WITH_KNOTS('',2,(#41616,#41617,#41618),
 .UNSPECIFIED.,.F.,.F.,(3,3),(0.,1.),.UNSPECIFIED.);
#737=B_SPLINE_CURVE_WITH_KNOTS('',2,(#41622,#41623,#41624),
 .UNSPECIFIED.,.F.,.F.,(3,3),(0.,1.),.UNSPECIFIED.);
#738=B_SPLINE_CURVE_WITH_KNOTS('',2,(#41633,#41634,#41635),
 .UNSPECIFIED.,.F.,.F.,(3,3),(0.,1.),.UNSPECIFIED.);
#739=B_SPLINE_CURVE_WITH_KNOTS('',2,(#41638,#41639,#41640),
 .UNSPECIFIED.,.F.,.F.,(3,3),(0.,1.),.UNSPECIFIED.);
#740=B_SPLINE_CURVE_WITH_KNOTS('',2,(#41648,#41649,#41650),
 .UNSPECIFIED.,.F.,.F.,(3,3),(0.,1.),.UNSPECIFIED.);
#741=B_SPLINE_CURVE_WITH_KNOTS('',2,(#41653,#41654,#41655),
 .UNSPECIFIED.,.F.,.F.,(3,3),(0.,1.),.UNSPECIFIED.);
#742=B_SPLINE_CURVE_WITH_KNOTS('',2,(#41663,#41664,#41665),
 .UNSPECIFIED.,.F.,.F.,(3,3),(0.,1.),.UNSPECIFIED.);
#743=B_SPLINE_CURVE_WITH_KNOTS('',2,(#41668,#41669,#41670),
 .UNSPECIFIED.,.F.,.F.,(3,3),(0.,1.),.UNSPECIFIED.);
#744=B_SPLINE_CURVE_WITH_KNOTS('',2,(#41678,#41679,#41680),
 .UNSPECIFIED.,.F.,.F.,(3,3),(0.,1.),.UNSPECIFIED.);
#745=B_SPLINE_CURVE_WITH_KNOTS('',2,(#41683,#41684,#41685),
 .UNSPECIFIED.,.F.,.F.,(3,3),(0.,1.),.UNSPECIFIED.);
#746=B_SPLINE_CURVE_WITH_KNOTS('',2,(#41693,#41694,#41695),
 .UNSPECIFIED.,.F.,.F.,(3,3),(0.,1.),.UNSPECIFIED.);
#747=B_SPLINE_CURVE_WITH_KNOTS('',2,(#41698,#41699,#41700),
 .UNSPECIFIED.,.F.,.F.,(3,3),(0.,1.),.UNSPECIFIED.);
#748=B_SPLINE_CURVE_WITH_KNOTS('',2,(#41708,#41709,#41710),
 .UNSPECIFIED.,.F.,.F.,(3,3),(0.,1.),.UNSPECIFIED.);
#749=B_SPLINE_CURVE_WITH_KNOTS('',2,(#41713,#41714,#41715),
 .UNSPECIFIED.,.F.,.F.,(3,3),(0.,1.),.UNSPECIFIED.);
#750=B_SPLINE_CURVE_WITH_KNOTS('',2,(#41723,#41724,#41725),
 .UNSPECIFIED.,.F.,.F.,(3,3),(0.,1.),.UNSPECIFIED.);
#751=B_SPLINE_CURVE_WITH_KNOTS('',2,(#41728,#41729,#41730),
 .UNSPECIFIED.,.F.,.F.,(3,3),(0.,1.),.UNSPECIFIED.);
#752=B_SPLINE_CURVE_WITH_KNOTS('',2,(#41737,#41738,#41739),
 .UNSPECIFIED.,.F.,.F.,(3,3),(0.,1.),.UNSPECIFIED.);
#753=B_SPLINE_CURVE_WITH_KNOTS('',2,(#41740,#41741,#41742),
 .UNSPECIFIED.,.F.,.F.,(3,3),(0.,1.),.UNSPECIFIED.);
#754=B_SPLINE_CURVE_WITH_KNOTS('',2,(#41752,#41753,#41754),
 .UNSPECIFIED.,.F.,.F.,(3,3),(0.,1.),.UNSPECIFIED.);
#755=B_SPLINE_CURVE_WITH_KNOTS('',2,(#41764,#41765,#41766),
 .UNSPECIFIED.,.F.,.F.,(3,3),(0.,1.),.UNSPECIFIED.);
#756=B_SPLINE_CURVE_WITH_KNOTS('',2,(#41775,#41776,#41777),
 .UNSPECIFIED.,.F.,.F.,(3,3),(0.,1.),.UNSPECIFIED.);
#757=B_SPLINE_CURVE_WITH_KNOTS('',2,(#41786,#41787,#41788),
 .UNSPECIFIED.,.F.,.F.,(3,3),(0.,1.),.UNSPECIFIED.);
#758=B_SPLINE_CURVE_WITH_KNOTS('',2,(#41797,#41798,#41799),
 .UNSPECIFIED.,.F.,.F.,(3,3),(0.,1.),.UNSPECIFIED.);
#759=B_SPLINE_CURVE_WITH_KNOTS('',2,(#41808,#41809,#41810),
 .UNSPECIFIED.,.F.,.F.,(3,3),(0.,1.),.UNSPECIFIED.);
#760=B_SPLINE_CURVE_WITH_KNOTS('',2,(#41819,#41820,#41821),
 .UNSPECIFIED.,.F.,.F.,(3,3),(0.,1.),.UNSPECIFIED.);
#761=B_SPLINE_CURVE_WITH_KNOTS('',2,(#41830,#41831,#41832),
 .UNSPECIFIED.,.F.,.F.,(3,3),(0.,1.),.UNSPECIFIED.);
#762=B_SPLINE_CURVE_WITH_KNOTS('',2,(#41841,#41842,#41843),
 .UNSPECIFIED.,.F.,.F.,(3,3),(0.,1.),.UNSPECIFIED.);
#763=B_SPLINE_CURVE_WITH_KNOTS('',2,(#41852,#41853,#41854),
 .UNSPECIFIED.,.F.,.F.,(3,3),(0.,1.),.UNSPECIFIED.);
#764=B_SPLINE_CURVE_WITH_KNOTS('',2,(#41863,#41864,#41865),
 .UNSPECIFIED.,.F.,.F.,(3,3),(0.,1.),.UNSPECIFIED.);
#765=B_SPLINE_CURVE_WITH_KNOTS('',2,(#41874,#41875,#41876),
 .UNSPECIFIED.,.F.,.F.,(3,3),(0.,1.),.UNSPECIFIED.);
#766=B_SPLINE_CURVE_WITH_KNOTS('',2,(#41883,#41884,#41885),
 .UNSPECIFIED.,.F.,.F.,(3,3),(0.,1.),.UNSPECIFIED.);
#767=B_SPLINE_CURVE_WITH_KNOTS('',2,(#41901,#41902,#41903),
 .UNSPECIFIED.,.F.,.F.,(3,3),(0.,1.),.UNSPECIFIED.);
#768=B_SPLINE_CURVE_WITH_KNOTS('',2,(#41912,#41913,#41914),
 .UNSPECIFIED.,.F.,.F.,(3,3),(0.,1.),.UNSPECIFIED.);
#769=B_SPLINE_CURVE_WITH_KNOTS('',2,(#41923,#41924,#41925),
 .UNSPECIFIED.,.F.,.F.,(3,3),(0.,1.),.UNSPECIFIED.);
#770=B_SPLINE_CURVE_WITH_KNOTS('',2,(#41934,#41935,#41936),
 .UNSPECIFIED.,.F.,.F.,(3,3),(0.,1.),.UNSPECIFIED.);
#771=B_SPLINE_CURVE_WITH_KNOTS('',2,(#41945,#41946,#41947),
 .UNSPECIFIED.,.F.,.F.,(3,3),(0.,1.),.UNSPECIFIED.);
#772=B_SPLINE_CURVE_WITH_KNOTS('',2,(#41956,#41957,#41958),
 .UNSPECIFIED.,.F.,.F.,(3,3),(0.,1.),.UNSPECIFIED.);
#773=B_SPLINE_CURVE_WITH_KNOTS('',2,(#41967,#41968,#41969),
 .UNSPECIFIED.,.F.,.F.,(3,3),(0.,1.),.UNSPECIFIED.);
#774=B_SPLINE_CURVE_WITH_KNOTS('',2,(#41978,#41979,#41980),
 .UNSPECIFIED.,.F.,.F.,(3,3),(0.,1.),.UNSPECIFIED.);
#775=B_SPLINE_CURVE_WITH_KNOTS('',2,(#41989,#41990,#41991),
 .UNSPECIFIED.,.F.,.F.,(3,3),(0.,1.),.UNSPECIFIED.);
#776=B_SPLINE_CURVE_WITH_KNOTS('',2,(#42000,#42001,#42002),
 .UNSPECIFIED.,.F.,.F.,(3,3),(0.,1.),.UNSPECIFIED.);
#777=B_SPLINE_CURVE_WITH_KNOTS('',2,(#42015,#42016,#42017),
 .UNSPECIFIED.,.F.,.F.,(3,3),(0.,1.),.UNSPECIFIED.);
#778=B_SPLINE_CURVE_WITH_KNOTS('',2,(#42026,#42027,#42028),
 .UNSPECIFIED.,.F.,.F.,(3,3),(0.,1.),.UNSPECIFIED.);
#779=B_SPLINE_CURVE_WITH_KNOTS('',2,(#42037,#42038,#42039),
 .UNSPECIFIED.,.F.,.F.,(3,3),(0.,1.),.UNSPECIFIED.);
#780=B_SPLINE_CURVE_WITH_KNOTS('',2,(#42048,#42049,#42050),
 .UNSPECIFIED.,.F.,.F.,(3,3),(0.,1.),.UNSPECIFIED.);
#781=B_SPLINE_CURVE_WITH_KNOTS('',2,(#42059,#42060,#42061),
 .UNSPECIFIED.,.F.,.F.,(3,3),(0.,1.),.UNSPECIFIED.);
#782=B_SPLINE_CURVE_WITH_KNOTS('',2,(#42070,#42071,#42072),
 .UNSPECIFIED.,.F.,.F.,(3,3),(0.,1.),.UNSPECIFIED.);
#783=B_SPLINE_CURVE_WITH_KNOTS('',2,(#42081,#42082,#42083),
 .UNSPECIFIED.,.F.,.F.,(3,3),(0.,1.),.UNSPECIFIED.);
#784=B_SPLINE_CURVE_WITH_KNOTS('',2,(#42092,#42093,#42094),
 .UNSPECIFIED.,.F.,.F.,(3,3),(0.,1.),.UNSPECIFIED.);
#1348=B_SPLINE_SURFACE_WITH_KNOTS('',3,3,((#37899,#37900,#37901,#37902,
#37903,#37904,#37905,#37906,#37907),(#37908,#37909,#37910,#37911,#37912,
#37913,#37914,#37915,#37916),(#37917,#37918,#37919,#37920,#37921,#37922,
#37923,#37924,#37925),(#37926,#37927,#37928,#37929,#37930,#37931,#37932,
#37933,#37934)),.UNSPECIFIED.,.F.,.F.,.F.,(4,4),(4,1,1,1,2,4),(0.,1.),(1.61732157627536,
1.83434749782276,2.05137341937016,2.26839934091757,2.70245118401238,2.76222327472562),
 .UNSPECIFIED.);
#1349=B_SPLINE_SURFACE_WITH_KNOTS('',3,3,((#37959,#37960,#37961,#37962),
(#37963,#37964,#37965,#37966),(#37967,#37968,#37969,#37970),(#37971,#37972,
#37973,#37974)),.UNSPECIFIED.,.F.,.F.,.F.,(4,4),(4,4),(0.,1.),(-2.03375105473527,
-1.90569248523429),.UNSPECIFIED.);
#1350=B_SPLINE_SURFACE_WITH_KNOTS('',3,3,((#37983,#37984,#37985,#37986),
(#37987,#37988,#37989,#37990),(#37991,#37992,#37993,#37994),(#37995,#37996,
#37997,#37998)),.UNSPECIFIED.,.F.,.F.,.F.,(4,4),(4,4),(0.,1.),(-1.2359001683555,
-1.10784159885376),.UNSPECIFIED.);
#1351=B_SPLINE_SURFACE_WITH_KNOTS('',3,3,((#38516,#38517,#38518,#38519,
#38520,#38521,#38522,#38523,#38524,#38525,#38526),(#38527,#38528,#38529,
#38530,#38531,#38532,#38533,#38534,#38535,#38536,#38537),(#38538,#38539,
#38540,#38541,#38542,#38543,#38544,#38545,#38546,#38547,#38548),(#38549,
#38550,#38551,#38552,#38553,#38554,#38555,#38556,#38557,#38558,#38559)),
 .UNSPECIFIED.,.F.,.F.,.F.,(4,4),(4,2,1,1,1,2,4),(0.,1.),(1.61732157627537,
1.67709366698862,2.08723667379813,2.39484392890525,2.49737968060763,2.70245118401238,
2.76222327472563),.UNSPECIFIED.);
#1352=B_SPLINE_SURFACE_WITH_KNOTS('',3,3,((#38575,#38576,#38577,#38578),
(#38579,#38580,#38581,#38582),(#38583,#38584,#38585,#38586),(#38587,#38588,
#38589,#38590)),.UNSPECIFIED.,.F.,.F.,.F.,(4,4),(4,4),(0.,1.),(1.10784159885453,
1.2359001683555),.UNSPECIFIED.);
#1353=B_SPLINE_SURFACE_WITH_KNOTS('',3,3,((#38595,#38596,#38597,#38598),
(#38599,#38600,#38601,#38602),(#38603,#38604,#38605,#38606),(#38607,#38608,
#38609,#38610)),.UNSPECIFIED.,.F.,.F.,.F.,(4,4),(4,4),(0.,1.),(1.9056924852343,
2.03375105473601),.UNSPECIFIED.);
#1354=B_SPLINE_SURFACE_WITH_KNOTS('',3,3,((#38671,#38672,#38673,#38674,
#38675,#38676,#38677,#38678,#38679,#38680),(#38681,#38682,#38683,#38684,
#38685,#38686,#38687,#38688,#38689,#38690),(#38691,#38692,#38693,#38694,
#38695,#38696,#38697,#38698,#38699,#38700),(#38701,#38702,#38703,#38704,
#38705,#38706,#38707,#38708,#38709,#38710)),.UNSPECIFIED.,.F.,.F.,.F.,(4,
4),(4,1,1,1,1,2,4),(0.,1.),(1.61732157627536,1.83434749782276,2.05137341937017,
2.26839934091757,2.48542526246498,2.70245118401238,2.76222327472564),
 .UNSPECIFIED.);
#1355=B_SPLINE_SURFACE_WITH_KNOTS('',3,3,((#38725,#38726,#38727,#38728),
(#38729,#38730,#38731,#38732),(#38733,#38734,#38735,#38736),(#38737,#38738,
#38739,#38740)),.UNSPECIFIED.,.F.,.F.,.F.,(4,4),(4,4),(0.,1.),(-2.03375105473527,
-1.90569248523429),.UNSPECIFIED.);
#1356=B_SPLINE_SURFACE_WITH_KNOTS('',3,3,((#38745,#38746,#38747,#38748),
(#38749,#38750,#38751,#38752),(#38753,#38754,#38755,#38756),(#38757,#38758,
#38759,#38760)),.UNSPECIFIED.,.F.,.F.,.F.,(4,4),(4,4),(0.,1.),(-1.2359001683555,
-1.10784159885378),.UNSPECIFIED.);
#1357=B_SPLINE_SURFACE_WITH_KNOTS('',3,3,((#38972,#38973,#38974,#38975,
#38976,#38977,#38978,#38979,#38980,#38981,#38982,#38983,#38984,#38985,#38986,
#38987,#38988,#38989,#38990,#38991),(#38992,#38993,#38994,#38995,#38996,
#38997,#38998,#38999,#39000,#39001,#39002,#39003,#39004,#39005,#39006,#39007,
#39008,#39009,#39010,#39011),(#39012,#39013,#39014,#39015,#39016,#39017,
#39018,#39019,#39020,#39021,#39022,#39023,#39024,#39025,#39026,#39027,#39028,
#39029,#39030,#39031),(#39032,#39033,#39034,#39035,#39036,#39037,#39038,
#39039,#39040,#39041,#39042,#39043,#39044,#39045,#39046,#39047,#39048,#39049,
#39050,#39051)),.UNSPECIFIED.,.F.,.F.,.F.,(4,4),(4,2,2,1,2,2,2,2,2,1,4),
(0.,1.),(0.779480614358526,0.806562617083009,0.843388556026078,1.45419115408482,
1.6577920201044,1.72690435024433,1.76021140268278,1.89936032175267,2.0015894299973,
2.60016813064741,2.79969436419745),.UNSPECIFIED.);
#1358=B_SPLINE_SURFACE_WITH_KNOTS('',3,3,((#39057,#39058,#39059,#39060),
(#39061,#39062,#39063,#39064),(#39065,#39066,#39067,#39068),(#39069,#39070,
#39071,#39072)),.UNSPECIFIED.,.F.,.F.,.F.,(4,4),(4,4),(0.,1.),(-0.985110783337743,
-0.90995102981447),.UNSPECIFIED.);
#1359=B_SPLINE_SURFACE_WITH_KNOTS('',3,3,((#39073,#39074,#39075,#39076),
(#39077,#39078,#39079,#39080),(#39081,#39082,#39083,#39084),(#39085,#39086,
#39087,#39088)),.UNSPECIFIED.,.F.,.F.,.F.,(4,4),(4,4),(0.,1.),(-2.23164162261785,
-2.15648187025204),.UNSPECIFIED.);
#1360=B_SPLINE_SURFACE_WITH_KNOTS('',3,3,((#39214,#39215,#39216,#39217,
#39218,#39219,#39220,#39221,#39222,#39223,#39224,#39225,#39226,#39227,#39228,
#39229,#39230,#39231,#39232,#39233,#39234),(#39235,#39236,#39237,#39238,
#39239,#39240,#39241,#39242,#39243,#39244,#39245,#39246,#39247,#39248,#39249,
#39250,#39251,#39252,#39253,#39254,#39255),(#39256,#39257,#39258,#39259,
#39260,#39261,#39262,#39263,#39264,#39265,#39266,#39267,#39268,#39269,#39270,
#39271,#39272,#39273,#39274,#39275,#39276),(#39277,#39278,#39279,#39280,
#39281,#39282,#39283,#39284,#39285,#39286,#39287,#39288,#39289,#39290,#39291,
#39292,#39293,#39294,#39295,#39296,#39297)),.UNSPECIFIED.,.F.,.F.,.F.,(4,
4),(4,2,2,1,2,1,2,1,2,1,2,1,4),(0.,1.),(0.779480614358288,0.806562617082741,
0.843388556025833,1.28514645313502,1.7269043502442,1.73523111335382,1.76021140268269,
1.82978586221579,1.89936032174889,1.95047487587308,2.00158942999727,2.60016813064741,
2.79969436419745),.UNSPECIFIED.);
#1361=B_SPLINE_SURFACE_WITH_KNOTS('',3,3,((#39303,#39304,#39305,#39306),
(#39307,#39308,#39309,#39310),(#39311,#39312,#39313,#39314),(#39315,#39316,
#39317,#39318)),.UNSPECIFIED.,.F.,.F.,.F.,(4,4),(4,4),(0.,1.),(2.15648187025205,
2.23164162377532),.UNSPECIFIED.);
#1362=B_SPLINE_SURFACE_WITH_KNOTS('',3,3,((#39319,#39320,#39321,#39322),
(#39323,#39324,#39325,#39326),(#39327,#39328,#39329,#39330),(#39331,#39332,
#39333,#39334)),.UNSPECIFIED.,.F.,.F.,.F.,(4,4),(4,4),(0.,1.),(0.90995103097194,
0.98511078333776),.UNSPECIFIED.);
#1363=B_SPLINE_SURFACE_WITH_KNOTS('',3,3,((#39335,#39336,#39337,#39338,
#39339,#39340,#39341,#39342,#39343,#39344,#39345,#39346,#39347,#39348,#39349,
#39350,#39351,#39352,#39353,#39354,#39355,#39356,#39357,#39358),(#39359,
#39360,#39361,#39362,#39363,#39364,#39365,#39366,#39367,#39368,#39369,#39370,
#39371,#39372,#39373,#39374,#39375,#39376,#39377,#39378,#39379,#39380,#39381,
#39382),(#39383,#39384,#39385,#39386,#39387,#39388,#39389,#39390,#39391,
#39392,#39393,#39394,#39395,#39396,#39397,#39398,#39399,#39400,#39401,#39402,
#39403,#39404,#39405,#39406),(#39407,#39408,#39409,#39410,#39411,#39412,
#39413,#39414,#39415,#39416,#39417,#39418,#39419,#39420,#39421,#39422,#39423,
#39424,#39425,#39426,#39427,#39428,#39429,#39430)),.UNSPECIFIED.,.F.,.F.,
 .F.,(4,4),(4,2,2,2,2,2,2,2,2,2,1,1,4),(0.,1.),(0.77948061435851,0.806562617082946,
0.843388556025962,1.50301394602541,1.65779202010408,1.72690435024419,1.76021140268274,
1.89936032174962,2.00158942999736,2.12581957279538,2.46275696849641,2.63122566634693,
2.79969436419745),.UNSPECIFIED.);
#1364=B_SPLINE_SURFACE_WITH_KNOTS('',3,3,((#39436,#39437,#39438,#39439),
(#39440,#39441,#39442,#39443),(#39444,#39445,#39446,#39447),(#39448,#39449,
#39450,#39451)),.UNSPECIFIED.,.F.,.F.,.F.,(4,4),(4,4),(0.,1.),(2.15648187025205,
2.23164162377532),.UNSPECIFIED.);
#1365=B_SPLINE_SURFACE_WITH_KNOTS('',3,3,((#39452,#39453,#39454,#39455),
(#39456,#39457,#39458,#39459),(#39460,#39461,#39462,#39463),(#39464,#39465,
#39466,#39467)),.UNSPECIFIED.,.F.,.F.,.F.,(4,4),(4,4),(0.,1.),(0.90995103097194,
0.985110783337756),.UNSPECIFIED.);
#1366=B_SPLINE_SURFACE_WITH_KNOTS('',3,3,((#39476,#39477,#39478,#39479,
#39480,#39481,#39482,#39483,#39484,#39485),(#39486,#39487,#39488,#39489,
#39490,#39491,#39492,#39493,#39494,#39495),(#39496,#39497,#39498,#39499,
#39500,#39501,#39502,#39503,#39504,#39505),(#39506,#39507,#39508,#39509,
#39510,#39511,#39512,#39513,#39514,#39515)),.UNSPECIFIED.,.F.,.F.,.F.,(4,
4),(4,2,1,1,2,4),(0.,1.),(1.61732157627537,1.67709366698862,2.08723667379812,
2.29230817720287,2.70245118401238,2.76222327472564),.UNSPECIFIED.);
#1367=B_SPLINE_SURFACE_WITH_KNOTS('',3,3,((#39530,#39531,#39532,#39533),
(#39534,#39535,#39536,#39537),(#39538,#39539,#39540,#39541),(#39542,#39543,
#39544,#39545)),.UNSPECIFIED.,.F.,.F.,.F.,(4,4),(4,4),(0.,1.),(1.10784159885453,
1.2359001683555),.UNSPECIFIED.);
#1368=B_SPLINE_SURFACE_WITH_KNOTS('',3,3,((#39550,#39551,#39552,#39553),
(#39554,#39555,#39556,#39557),(#39558,#39559,#39560,#39561),(#39562,#39563,
#39564,#39565)),.UNSPECIFIED.,.F.,.F.,.F.,(4,4),(4,4),(0.,1.),(1.9056924852343,
2.03375105473602),.UNSPECIFIED.);
#1369=B_SPLINE_SURFACE_WITH_KNOTS('',3,3,((#39618,#39619,#39620,#39621,
#39622,#39623,#39624,#39625,#39626,#39627,#39628,#39629,#39630,#39631,#39632,
#39633,#39634,#39635),(#39636,#39637,#39638,#39639,#39640,#39641,#39642,
#39643,#39644,#39645,#39646,#39647,#39648,#39649,#39650,#39651,#39652,#39653),
(#39654,#39655,#39656,#39657,#39658,#39659,#39660,#39661,#39662,#39663,
#39664,#39665,#39666,#39667,#39668,#39669,#39670,#39671),(#39672,#39673,
#39674,#39675,#39676,#39677,#39678,#39679,#39680,#39681,#39682,#39683,#39684,
#39685,#39686,#39687,#39688,#39689)),.UNSPECIFIED.,.F.,.F.,.F.,(4,4),(4,
2,2,1,1,2,2,2,1,1,4),(0.,1.),(0.779480614358544,0.806562617082991,0.843388556026153,
1.28514645313595,1.50602540169085,1.72690435024575,1.76021140268327,1.89936032175298,
2.57461085358633,2.68715260889189,2.79969436419745),.UNSPECIFIED.);
#1370=B_SPLINE_SURFACE_WITH_KNOTS('',3,3,((#39695,#39696,#39697,#39698),
(#39699,#39700,#39701,#39702),(#39703,#39704,#39705,#39706),(#39707,#39708,
#39709,#39710)),.UNSPECIFIED.,.F.,.F.,.F.,(4,4),(4,4),(0.,1.),(-0.985110783337744,
-0.909951029814477),.UNSPECIFIED.);
#1371=B_SPLINE_SURFACE_WITH_KNOTS('',3,3,((#39711,#39712,#39713,#39714),
(#39715,#39716,#39717,#39718),(#39719,#39720,#39721,#39722),(#39723,#39724,
#39725,#39726)),.UNSPECIFIED.,.F.,.F.,.F.,(4,4),(4,4),(0.,1.),(-2.23164162261785,
-2.15648187025204),.UNSPECIFIED.);
#1372=B_SPLINE_SURFACE_WITH_KNOTS('',3,3,((#39967,#39968,#39969,#39970,
#39971,#39972,#39973,#39974,#39975,#39976),(#39977,#39978,#39979,#39980,
#39981,#39982,#39983,#39984,#39985,#39986),(#39987,#39988,#39989,#39990,
#39991,#39992,#39993,#39994,#39995,#39996),(#39997,#39998,#39999,#40000,
#40001,#40002,#40003,#40004,#40005,#40006)),.UNSPECIFIED.,.F.,.F.,.F.,(4,
4),(4,2,1,1,2,4),(0.,1.),(1.61732157627537,1.67709366698862,2.08723667379812,
2.29230817720287,2.70245118401238,2.76222327472564),.UNSPECIFIED.);
#1373=B_SPLINE_SURFACE_WITH_KNOTS('',3,3,((#40029,#40030,#40031,#40032),
(#40033,#40034,#40035,#40036),(#40037,#40038,#40039,#40040),(#40041,#40042,
#40043,#40044)),.UNSPECIFIED.,.F.,.F.,.F.,(4,4),(4,4),(0.,1.),(1.9056924852343,
2.03375105473599),.UNSPECIFIED.);
#1374=B_SPLINE_SURFACE_WITH_KNOTS('',3,3,((#40049,#40050,#40051,#40052),
(#40053,#40054,#40055,#40056),(#40057,#40058,#40059,#40060),(#40061,#40062,
#40063,#40064)),.UNSPECIFIED.,.F.,.F.,.F.,(4,4),(4,4),(0.,1.),(1.10784159885453,
1.23590016835551),.UNSPECIFIED.);
#1375=B_SPLINE_SURFACE_WITH_KNOTS('',3,3,((#40386,#40387,#40388,#40389,
#40390,#40391,#40392,#40393,#40394,#40395,#40396,#40397,#40398,#40399,#40400,
#40401,#40402,#40403,#40404,#40405),(#40406,#40407,#40408,#40409,#40410,
#40411,#40412,#40413,#40414,#40415,#40416,#40417,#40418,#40419,#40420,#40421,
#40422,#40423,#40424,#40425),(#40426,#40427,#40428,#40429,#40430,#40431,
#40432,#40433,#40434,#40435,#40436,#40437,#40438,#40439,#40440,#40441,#40442,
#40443,#40444,#40445),(#40446,#40447,#40448,#40449,#40450,#40451,#40452,
#40453,#40454,#40455,#40456,#40457,#40458,#40459,#40460,#40461,#40462,#40463,
#40464,#40465)),.UNSPECIFIED.,.F.,.F.,.F.,(4,4),(4,2,2,1,1,2,2,2,2,1,1,
4),(0.,1.),(0.779480614358656,0.806562617083063,0.843388556026148,1.28514645313547,
1.50602540169013,1.7269043502448,1.76021140268296,1.82544138032945,1.89936032174889,
2.57461085358531,2.68715260889138,2.79969436419745),.UNSPECIFIED.);
#1376=B_SPLINE_SURFACE_WITH_KNOTS('',3,3,((#40471,#40472,#40473,#40474),
(#40475,#40476,#40477,#40478),(#40479,#40480,#40481,#40482),(#40483,#40484,
#40485,#40486)),.UNSPECIFIED.,.F.,.F.,.F.,(4,4),(4,4),(0.,1.),(-0.985110783337744,
-0.909951029814477),.UNSPECIFIED.);
#1377=B_SPLINE_SURFACE_WITH_KNOTS('',3,3,((#40487,#40488,#40489,#40490),
(#40491,#40492,#40493,#40494),(#40495,#40496,#40497,#40498),(#40499,#40500,
#40501,#40502)),.UNSPECIFIED.,.F.,.F.,.F.,(4,4),(4,4),(0.,1.),(-2.23164162261785,
-2.15648187025204),.UNSPECIFIED.);
#1378=B_SPLINE_SURFACE_WITH_KNOTS('',3,3,((#40511,#40512,#40513,#40514,
#40515,#40516,#40517,#40518,#40519,#40520),(#40521,#40522,#40523,#40524,
#40525,#40526,#40527,#40528,#40529,#40530),(#40531,#40532,#40533,#40534,
#40535,#40536,#40537,#40538,#40539,#40540),(#40541,#40542,#40543,#40544,
#40545,#40546,#40547,#40548,#40549,#40550)),.UNSPECIFIED.,.F.,.F.,.F.,(4,
4),(4,2,1,1,2,4),(0.,1.),(1.61732157627537,1.67709366698862,2.08723667379812,
2.29230817720288,2.70245118401238,2.76222327472563),.UNSPECIFIED.);
#1379=B_SPLINE_SURFACE_WITH_KNOTS('',3,3,((#40565,#40566,#40567,#40568),
(#40569,#40570,#40571,#40572),(#40573,#40574,#40575,#40576),(#40577,#40578,
#40579,#40580)),.UNSPECIFIED.,.F.,.F.,.F.,(4,4),(4,4),(0.,1.),(-2.03375105473527,
-1.90569248523429),.UNSPECIFIED.);
#1380=B_SPLINE_SURFACE_WITH_KNOTS('',3,3,((#40585,#40586,#40587,#40588),
(#40589,#40590,#40591,#40592),(#40593,#40594,#40595,#40596),(#40597,#40598,
#40599,#40600)),.UNSPECIFIED.,.F.,.F.,.F.,(4,4),(4,4),(0.,1.),(-1.2359001683555,
-1.10784159885378),.UNSPECIFIED.);
#1381=B_SPLINE_SURFACE_WITH_KNOTS('',3,3,((#40653,#40654,#40655,#40656,
#40657,#40658,#40659,#40660,#40661,#40662,#40663,#40664,#40665,#40666,#40667,
#40668,#40669,#40670,#40671,#40672),(#40673,#40674,#40675,#40676,#40677,
#40678,#40679,#40680,#40681,#40682,#40683,#40684,#40685,#40686,#40687,#40688,
#40689,#40690,#40691,#40692),(#40693,#40694,#40695,#40696,#40697,#40698,
#40699,#40700,#40701,#40702,#40703,#40704,#40705,#40706,#40707,#40708,#40709,
#40710,#40711,#40712),(#40713,#40714,#40715,#40716,#40717,#40718,#40719,
#40720,#40721,#40722,#40723,#40724,#40725,#40726,#40727,#40728,#40729,#40730,
#40731,#40732)),.UNSPECIFIED.,.F.,.F.,.F.,(4,4),(4,2,2,1,2,2,2,2,2,1,4),
(0.,1.),(0.77948061435839,0.806562617082694,0.843388556025742,1.45419115408438,
1.65779202010392,1.72690435024413,1.76021140268269,1.89936032174878,2.00158942999731,
2.60016813064743,2.79969436419747),.UNSPECIFIED.);
#1382=B_SPLINE_SURFACE_WITH_KNOTS('',3,3,((#40738,#40739,#40740,#40741),
(#40742,#40743,#40744,#40745),(#40746,#40747,#40748,#40749),(#40750,#40751,
#40752,#40753)),.UNSPECIFIED.,.F.,.F.,.F.,(4,4),(4,4),(0.,1.),(2.15648187025205,
2.23164162377532),.UNSPECIFIED.);
#1383=B_SPLINE_SURFACE_WITH_KNOTS('',3,3,((#40754,#40755,#40756,#40757),
(#40758,#40759,#40760,#40761),(#40762,#40763,#40764,#40765),(#40766,#40767,
#40768,#40769)),.UNSPECIFIED.,.F.,.F.,.F.,(4,4),(4,4),(0.,1.),(0.90995103097194,
0.985110783337756),.UNSPECIFIED.);
#1384=B_SPLINE_SURFACE_WITH_KNOTS('',3,3,((#40770,#40771,#40772,#40773,
#40774,#40775,#40776,#40777,#40778,#40779,#40780),(#40781,#40782,#40783,
#40784,#40785,#40786,#40787,#40788,#40789,#40790,#40791),(#40792,#40793,
#40794,#40795,#40796,#40797,#40798,#40799,#40800,#40801,#40802),(#40803,
#40804,#40805,#40806,#40807,#40808,#40809,#40810,#40811,#40812,#40813)),
 .UNSPECIFIED.,.F.,.F.,.F.,(4,4),(4,2,1,1,1,2,4),(0.,1.),(1.61732157627537,
1.67709366698862,2.08723667379813,2.39484392890525,2.49737968060763,2.70245118401238,
2.76222327472563),.UNSPECIFIED.);
#1385=B_SPLINE_SURFACE_WITH_KNOTS('',3,3,((#40837,#40838,#40839,#40840),
(#40841,#40842,#40843,#40844),(#40845,#40846,#40847,#40848),(#40849,#40850,
#40851,#40852)),.UNSPECIFIED.,.F.,.F.,.F.,(4,4),(4,4),(0.,1.),(1.9056924852343,
2.03375105473601),.UNSPECIFIED.);
#1386=B_SPLINE_SURFACE_WITH_KNOTS('',3,3,((#40857,#40858,#40859,#40860),
(#40861,#40862,#40863,#40864),(#40865,#40866,#40867,#40868),(#40869,#40870,
#40871,#40872)),.UNSPECIFIED.,.F.,.F.,.F.,(4,4),(4,4),(0.,1.),(1.10784159885453,
1.2359001683555),.UNSPECIFIED.);
#1387=B_SPLINE_SURFACE_WITH_KNOTS('',3,3,((#40925,#40926,#40927,#40928,
#40929,#40930,#40931,#40932,#40933,#40934,#40935,#40936,#40937,#40938,#40939,
#40940,#40941,#40942,#40943,#40944,#40945),(#40946,#40947,#40948,#40949,
#40950,#40951,#40952,#40953,#40954,#40955,#40956,#40957,#40958,#40959,#40960,
#40961,#40962,#40963,#40964,#40965,#40966),(#40967,#40968,#40969,#40970,
#40971,#40972,#40973,#40974,#40975,#40976,#40977,#40978,#40979,#40980,#40981,
#40982,#40983,#40984,#40985,#40986,#40987),(#40988,#40989,#40990,#40991,
#40992,#40993,#40994,#40995,#40996,#40997,#40998,#40999,#41000,#41001,#41002,
#41003,#41004,#41005,#41006,#41007,#41008)),.UNSPECIFIED.,.F.,.F.,.F.,(4,
4),(4,2,2,2,2,2,2,2,2,1,4),(0.,1.),(0.779480614358366,0.806562617082747,
0.84338855602576,1.65779202010374,1.72690435024399,1.76021140268264,1.82544138032896,
1.89936032174887,2.00158942999732,2.60016813064742,2.79969436419746),
 .UNSPECIFIED.);
#1388=B_SPLINE_SURFACE_WITH_KNOTS('',3,3,((#41014,#41015,#41016,#41017),
(#41018,#41019,#41020,#41021),(#41022,#41023,#41024,#41025),(#41026,#41027,
#41028,#41029)),.UNSPECIFIED.,.F.,.F.,.F.,(4,4),(4,4),(0.,1.),(-0.985110783337743,
-0.90995102981447),.UNSPECIFIED.);
#1389=B_SPLINE_SURFACE_WITH_KNOTS('',3,3,((#41030,#41031,#41032,#41033),
(#41034,#41035,#41036,#41037),(#41038,#41039,#41040,#41041),(#41042,#41043,
#41044,#41045)),.UNSPECIFIED.,.F.,.F.,.F.,(4,4),(4,4),(0.,1.),(-2.23164162261785,
-2.15648187025204),.UNSPECIFIED.);
#1390=B_SPLINE_SURFACE_WITH_KNOTS('',3,3,((#41054,#41055,#41056,#41057,
#41058,#41059,#41060,#41061,#41062,#41063),(#41064,#41065,#41066,#41067,
#41068,#41069,#41070,#41071,#41072,#41073),(#41074,#41075,#41076,#41077,
#41078,#41079,#41080,#41081,#41082,#41083),(#41084,#41085,#41086,#41087,
#41088,#41089,#41090,#41091,#41092,#41093)),.UNSPECIFIED.,.F.,.F.,.F.,(4,
4),(4,2,1,1,2,4),(0.,1.),(1.61732157627537,1.67709366698862,2.08723667379812,
2.29230817720287,2.70245118401238,2.76222327472562),.UNSPECIFIED.);
#1391=B_SPLINE_SURFACE_WITH_KNOTS('',3,3,((#41108,#41109,#41110,#41111),
(#41112,#41113,#41114,#41115),(#41116,#41117,#41118,#41119),(#41120,#41121,
#41122,#41123)),.UNSPECIFIED.,.F.,.F.,.F.,(4,4),(4,4),(0.,1.),(-2.03375105473527,
-1.90569248523429),.UNSPECIFIED.);
#1392=B_SPLINE_SURFACE_WITH_KNOTS('',3,3,((#41128,#41129,#41130,#41131),
(#41132,#41133,#41134,#41135),(#41136,#41137,#41138,#41139),(#41140,#41141,
#41142,#41143)),.UNSPECIFIED.,.F.,.F.,.F.,(4,4),(4,4),(0.,1.),(-1.23590016835549,
-1.10784159885377),.UNSPECIFIED.);
#1393=B_SPLINE_SURFACE_WITH_KNOTS('',3,3,((#41196,#41197,#41198,#41199,
#41200,#41201,#41202,#41203,#41204,#41205,#41206,#41207,#41208,#41209,#41210,
#41211,#41212,#41213,#41214,#41215),(#41216,#41217,#41218,#41219,#41220,
#41221,#41222,#41223,#41224,#41225,#41226,#41227,#41228,#41229,#41230,#41231,
#41232,#41233,#41234,#41235),(#41236,#41237,#41238,#41239,#41240,#41241,
#41242,#41243,#41244,#41245,#41246,#41247,#41248,#41249,#41250,#41251,#41252,
#41253,#41254,#41255),(#41256,#41257,#41258,#41259,#41260,#41261,#41262,
#41263,#41264,#41265,#41266,#41267,#41268,#41269,#41270,#41271,#41272,#41273,
#41274,#41275)),.UNSPECIFIED.,.F.,.F.,.F.,(4,4),(4,2,2,2,2,2,2,2,1,1,4),
(0.,1.),(0.779480614358288,0.806562617082717,0.843388556025879,1.65779202010542,
1.72690435024458,1.76021140268281,1.8254413803293,1.89936032174935,2.57461085358543,
2.68715260889144,2.79969436419745),.UNSPECIFIED.);
#1394=B_SPLINE_SURFACE_WITH_KNOTS('',3,3,((#41281,#41282,#41283,#41284),
(#41285,#41286,#41287,#41288),(#41289,#41290,#41291,#41292),(#41293,#41294,
#41295,#41296)),.UNSPECIFIED.,.F.,.F.,.F.,(4,4),(4,4),(0.,1.),(2.15648187025205,
2.23164162377533),.UNSPECIFIED.);
#1395=B_SPLINE_SURFACE_WITH_KNOTS('',3,3,((#41297,#41298,#41299,#41300),
(#41301,#41302,#41303,#41304),(#41305,#41306,#41307,#41308),(#41309,#41310,
#41311,#41312)),.UNSPECIFIED.,.F.,.F.,.F.,(4,4),(4,4),(0.,1.),(0.90995103097194,
0.985110783337753),.UNSPECIFIED.);
#1396=B_SPLINE_SURFACE_WITH_KNOTS('',2,1,((#41344,#41345),(#41346,#41347),
(#41348,#41349)),.UNSPECIFIED.,.F.,.F.,.F.,(3,3),(2,2),(0.,1.),(0.,0.0999999999999996),
 .UNSPECIFIED.);
#1397=B_SPLINE_SURFACE_WITH_KNOTS('',2,1,((#41362,#41363),(#41364,#41365),
(#41366,#41367)),.UNSPECIFIED.,.F.,.F.,.F.,(3,3),(2,2),(0.,1.),(0.,0.0999999999999996),
 .UNSPECIFIED.);
#1398=B_SPLINE_SURFACE_WITH_KNOTS('',2,1,((#41377,#41378),(#41379,#41380),
(#41381,#41382)),.UNSPECIFIED.,.F.,.F.,.F.,(3,3),(2,2),(0.,1.),(0.,0.0999999999999996),
 .UNSPECIFIED.);
#1399=B_SPLINE_SURFACE_WITH_KNOTS('',2,1,((#41392,#41393),(#41394,#41395),
(#41396,#41397)),.UNSPECIFIED.,.F.,.F.,.F.,(3,3),(2,2),(0.,1.),(0.,0.0999999999999996),
 .UNSPECIFIED.);
#1400=B_SPLINE_SURFACE_WITH_KNOTS('',2,1,((#41407,#41408),(#41409,#41410),
(#41411,#41412)),.UNSPECIFIED.,.F.,.F.,.F.,(3,3),(2,2),(0.,1.),(0.,0.0999999999999996),
 .UNSPECIFIED.);
#1401=B_SPLINE_SURFACE_WITH_KNOTS('',2,1,((#41422,#41423),(#41424,#41425),
(#41426,#41427)),.UNSPECIFIED.,.F.,.F.,.F.,(3,3),(2,2),(0.,1.),(0.,0.0999999999999996),
 .UNSPECIFIED.);
#1402=B_SPLINE_SURFACE_WITH_KNOTS('',2,1,((#41437,#41438),(#41439,#41440),
(#41441,#41442)),.UNSPECIFIED.,.F.,.F.,.F.,(3,3),(2,2),(0.,1.),(0.,0.0999999999999996),
 .UNSPECIFIED.);
#1403=B_SPLINE_SURFACE_WITH_KNOTS('',2,1,((#41452,#41453),(#41454,#41455),
(#41456,#41457)),.UNSPECIFIED.,.F.,.F.,.F.,(3,3),(2,2),(0.,1.),(0.,0.0999999999999996),
 .UNSPECIFIED.);
#1404=B_SPLINE_SURFACE_WITH_KNOTS('',2,1,((#41464,#41465),(#41466,#41467),
(#41468,#41469)),.UNSPECIFIED.,.F.,.F.,.F.,(3,3),(2,2),(0.,1.),(0.,0.0999999999999996),
 .UNSPECIFIED.);
#1405=B_SPLINE_SURFACE_WITH_KNOTS('',2,1,((#41477,#41478),(#41479,#41480),
(#41481,#41482)),.UNSPECIFIED.,.F.,.F.,.F.,(3,3),(2,2),(0.,1.),(0.,0.0999999999999996),
 .UNSPECIFIED.);
#1406=B_SPLINE_SURFACE_WITH_KNOTS('',2,1,((#41488,#41489),(#41490,#41491),
(#41492,#41493)),.UNSPECIFIED.,.F.,.F.,.F.,(3,3),(2,2),(0.,1.),(0.,0.0999999999999996),
 .UNSPECIFIED.);
#1407=B_SPLINE_SURFACE_WITH_KNOTS('',2,1,((#41499,#41500),(#41501,#41502),
(#41503,#41504)),.UNSPECIFIED.,.F.,.F.,.F.,(3,3),(2,2),(0.,1.),(0.,0.0999999999999996),
 .UNSPECIFIED.);
#1408=B_SPLINE_SURFACE_WITH_KNOTS('',2,1,((#41510,#41511),(#41512,#41513),
(#41514,#41515)),.UNSPECIFIED.,.F.,.F.,.F.,(3,3),(2,2),(0.,1.),(0.,0.0999999999999996),
 .UNSPECIFIED.);
#1409=B_SPLINE_SURFACE_WITH_KNOTS('',2,1,((#41521,#41522),(#41523,#41524),
(#41525,#41526)),.UNSPECIFIED.,.F.,.F.,.F.,(3,3),(2,2),(0.,1.),(0.,0.0999999999999996),
 .UNSPECIFIED.);
#1410=B_SPLINE_SURFACE_WITH_KNOTS('',2,1,((#41532,#41533),(#41534,#41535),
(#41536,#41537)),.UNSPECIFIED.,.F.,.F.,.F.,(3,3),(2,2),(0.,1.),(0.,0.0999999999999996),
 .UNSPECIFIED.);
#1411=B_SPLINE_SURFACE_WITH_KNOTS('',2,1,((#41543,#41544),(#41545,#41546),
(#41547,#41548)),.UNSPECIFIED.,.F.,.F.,.F.,(3,3),(2,2),(0.,1.),(0.,0.0999999999999996),
 .UNSPECIFIED.);
#1412=B_SPLINE_SURFACE_WITH_KNOTS('',2,1,((#41554,#41555),(#41556,#41557),
(#41558,#41559)),.UNSPECIFIED.,.F.,.F.,.F.,(3,3),(2,2),(0.,1.),(0.,0.0999999999999996),
 .UNSPECIFIED.);
#1413=B_SPLINE_SURFACE_WITH_KNOTS('',2,1,((#41565,#41566),(#41567,#41568),
(#41569,#41570)),.UNSPECIFIED.,.F.,.F.,.F.,(3,3),(2,2),(0.,1.),(0.,0.0999999999999996),
 .UNSPECIFIED.);
#1414=B_SPLINE_SURFACE_WITH_KNOTS('',2,1,((#41608,#41609),(#41610,#41611),
(#41612,#41613)),.UNSPECIFIED.,.F.,.F.,.F.,(3,3),(2,2),(0.,1.),(0.,0.0999999999999996),
 .UNSPECIFIED.);
#1415=B_SPLINE_SURFACE_WITH_KNOTS('',2,1,((#41626,#41627),(#41628,#41629),
(#41630,#41631)),.UNSPECIFIED.,.F.,.F.,.F.,(3,3),(2,2),(0.,1.),(0.,0.0999999999999996),
 .UNSPECIFIED.);
#1416=B_SPLINE_SURFACE_WITH_KNOTS('',2,1,((#41641,#41642),(#41643,#41644),
(#41645,#41646)),.UNSPECIFIED.,.F.,.F.,.F.,(3,3),(2,2),(0.,1.),(0.,0.0999999999999996),
 .UNSPECIFIED.);
#1417=B_SPLINE_SURFACE_WITH_KNOTS('',2,1,((#41656,#41657),(#41658,#41659),
(#41660,#41661)),.UNSPECIFIED.,.F.,.F.,.F.,(3,3),(2,2),(0.,1.),(0.,0.0999999999999996),
 .UNSPECIFIED.);
#1418=B_SPLINE_SURFACE_WITH_KNOTS('',2,1,((#41671,#41672),(#41673,#41674),
(#41675,#41676)),.UNSPECIFIED.,.F.,.F.,.F.,(3,3),(2,2),(0.,1.),(0.,0.0999999999999996),
 .UNSPECIFIED.);
#1419=B_SPLINE_SURFACE_WITH_KNOTS('',2,1,((#41686,#41687),(#41688,#41689),
(#41690,#41691)),.UNSPECIFIED.,.F.,.F.,.F.,(3,3),(2,2),(0.,1.),(0.,0.0999999999999996),
 .UNSPECIFIED.);
#1420=B_SPLINE_SURFACE_WITH_KNOTS('',2,1,((#41701,#41702),(#41703,#41704),
(#41705,#41706)),.UNSPECIFIED.,.F.,.F.,.F.,(3,3),(2,2),(0.,1.),(0.,0.0999999999999996),
 .UNSPECIFIED.);
#1421=B_SPLINE_SURFACE_WITH_KNOTS('',2,1,((#41716,#41717),(#41718,#41719),
(#41720,#41721)),.UNSPECIFIED.,.F.,.F.,.F.,(3,3),(2,2),(0.,1.),(0.,0.0999999999999996),
 .UNSPECIFIED.);
#1422=B_SPLINE_SURFACE_WITH_KNOTS('',2,1,((#41731,#41732),(#41733,#41734),
(#41735,#41736)),.UNSPECIFIED.,.F.,.F.,.F.,(3,3),(2,2),(0.,1.),(0.,0.0999999999999996),
 .UNSPECIFIED.);
#1423=B_SPLINE_SURFACE_WITH_KNOTS('',2,1,((#41743,#41744),(#41745,#41746),
(#41747,#41748)),.UNSPECIFIED.,.F.,.F.,.F.,(3,3),(2,2),(0.,1.),(0.,0.0999999999999996),
 .UNSPECIFIED.);
#1424=B_SPLINE_SURFACE_WITH_KNOTS('',2,1,((#41756,#41757),(#41758,#41759),
(#41760,#41761)),.UNSPECIFIED.,.F.,.F.,.F.,(3,3),(2,2),(0.,1.),(0.,0.0999999999999996),
 .UNSPECIFIED.);
#1425=B_SPLINE_SURFACE_WITH_KNOTS('',2,1,((#41767,#41768),(#41769,#41770),
(#41771,#41772)),.UNSPECIFIED.,.F.,.F.,.F.,(3,3),(2,2),(0.,1.),(0.,0.0999999999999996),
 .UNSPECIFIED.);
#1426=B_SPLINE_SURFACE_WITH_KNOTS('',2,1,((#41778,#41779),(#41780,#41781),
(#41782,#41783)),.UNSPECIFIED.,.F.,.F.,.F.,(3,3),(2,2),(0.,1.),(0.,0.0999999999999996),
 .UNSPECIFIED.);
#1427=B_SPLINE_SURFACE_WITH_KNOTS('',2,1,((#41789,#41790),(#41791,#41792),
(#41793,#41794)),.UNSPECIFIED.,.F.,.F.,.F.,(3,3),(2,2),(0.,1.),(0.,0.0999999999999996),
 .UNSPECIFIED.);
#1428=B_SPLINE_SURFACE_WITH_KNOTS('',2,1,((#41800,#41801),(#41802,#41803),
(#41804,#41805)),.UNSPECIFIED.,.F.,.F.,.F.,(3,3),(2,2),(0.,1.),(0.,0.0999999999999996),
 .UNSPECIFIED.);
#1429=B_SPLINE_SURFACE_WITH_KNOTS('',2,1,((#41811,#41812),(#41813,#41814),
(#41815,#41816)),.UNSPECIFIED.,.F.,.F.,.F.,(3,3),(2,2),(0.,1.),(0.,0.0999999999999996),
 .UNSPECIFIED.);
#1430=B_SPLINE_SURFACE_WITH_KNOTS('',2,1,((#41822,#41823),(#41824,#41825),
(#41826,#41827)),.UNSPECIFIED.,.F.,.F.,.F.,(3,3),(2,2),(0.,1.),(0.,0.0999999999999996),
 .UNSPECIFIED.);
#1431=B_SPLINE_SURFACE_WITH_KNOTS('',2,1,((#41833,#41834),(#41835,#41836),
(#41837,#41838)),.UNSPECIFIED.,.F.,.F.,.F.,(3,3),(2,2),(0.,1.),(0.,0.0999999999999996),
 .UNSPECIFIED.);
#1432=B_SPLINE_SURFACE_WITH_KNOTS('',2,1,((#41844,#41845),(#41846,#41847),
(#41848,#41849)),.UNSPECIFIED.,.F.,.F.,.F.,(3,3),(2,2),(0.,1.),(0.,0.0999999999999996),
 .UNSPECIFIED.);
#1433=B_SPLINE_SURFACE_WITH_KNOTS('',2,1,((#41855,#41856),(#41857,#41858),
(#41859,#41860)),.UNSPECIFIED.,.F.,.F.,.F.,(3,3),(2,2),(0.,1.),(0.,0.0999999999999996),
 .UNSPECIFIED.);
#1434=B_SPLINE_SURFACE_WITH_KNOTS('',2,1,((#41866,#41867),(#41868,#41869),
(#41870,#41871)),.UNSPECIFIED.,.F.,.F.,.F.,(3,3),(2,2),(0.,1.),(0.,0.0999999999999996),
 .UNSPECIFIED.);
#1435=B_SPLINE_SURFACE_WITH_KNOTS('',2,1,((#41877,#41878),(#41879,#41880),
(#41881,#41882)),.UNSPECIFIED.,.F.,.F.,.F.,(3,3),(2,2),(0.,1.),(0.,0.0999999999999996),
 .UNSPECIFIED.);
#1436=B_SPLINE_SURFACE_WITH_KNOTS('',2,1,((#41893,#41894),(#41895,#41896),
(#41897,#41898)),.UNSPECIFIED.,.F.,.F.,.F.,(3,3),(2,2),(0.,1.),(0.,0.0999999999999996),
 .UNSPECIFIED.);
#1437=B_SPLINE_SURFACE_WITH_KNOTS('',2,1,((#41904,#41905),(#41906,#41907),
(#41908,#41909)),.UNSPECIFIED.,.F.,.F.,.F.,(3,3),(2,2),(0.,1.),(0.,0.0999999999999996),
 .UNSPECIFIED.);
#1438=B_SPLINE_SURFACE_WITH_KNOTS('',2,1,((#41915,#41916),(#41917,#41918),
(#41919,#41920)),.UNSPECIFIED.,.F.,.F.,.F.,(3,3),(2,2),(0.,1.),(0.,0.0999999999999996),
 .UNSPECIFIED.);
#1439=B_SPLINE_SURFACE_WITH_KNOTS('',2,1,((#41926,#41927),(#41928,#41929),
(#41930,#41931)),.UNSPECIFIED.,.F.,.F.,.F.,(3,3),(2,2),(0.,1.),(0.,0.0999999999999996),
 .UNSPECIFIED.);
#1440=B_SPLINE_SURFACE_WITH_KNOTS('',2,1,((#41937,#41938),(#41939,#41940),
(#41941,#41942)),.UNSPECIFIED.,.F.,.F.,.F.,(3,3),(2,2),(0.,1.),(0.,0.0999999999999996),
 .UNSPECIFIED.);
#1441=B_SPLINE_SURFACE_WITH_KNOTS('',2,1,((#41948,#41949),(#41950,#41951),
(#41952,#41953)),.UNSPECIFIED.,.F.,.F.,.F.,(3,3),(2,2),(0.,1.),(0.,0.0999999999999996),
 .UNSPECIFIED.);
#1442=B_SPLINE_SURFACE_WITH_KNOTS('',2,1,((#41959,#41960),(#41961,#41962),
(#41963,#41964)),.UNSPECIFIED.,.F.,.F.,.F.,(3,3),(2,2),(0.,1.),(0.,0.0999999999999996),
 .UNSPECIFIED.);
#1443=B_SPLINE_SURFACE_WITH_KNOTS('',2,1,((#41970,#41971),(#41972,#41973),
(#41974,#41975)),.UNSPECIFIED.,.F.,.F.,.F.,(3,3),(2,2),(0.,1.),(0.,0.0999999999999996),
 .UNSPECIFIED.);
#1444=B_SPLINE_SURFACE_WITH_KNOTS('',2,1,((#41981,#41982),(#41983,#41984),
(#41985,#41986)),.UNSPECIFIED.,.F.,.F.,.F.,(3,3),(2,2),(0.,1.),(0.,0.0999999999999996),
 .UNSPECIFIED.);
#1445=B_SPLINE_SURFACE_WITH_KNOTS('',2,1,((#41992,#41993),(#41994,#41995),
(#41996,#41997)),.UNSPECIFIED.,.F.,.F.,.F.,(3,3),(2,2),(0.,1.),(0.,0.0999999999999996),
 .UNSPECIFIED.);
#1446=B_SPLINE_SURFACE_WITH_KNOTS('',2,1,((#42007,#42008),(#42009,#42010),
(#42011,#42012)),.UNSPECIFIED.,.F.,.F.,.F.,(3,3),(2,2),(0.,1.),(0.,0.0999999999999996),
 .UNSPECIFIED.);
#1447=B_SPLINE_SURFACE_WITH_KNOTS('',2,1,((#42018,#42019),(#42020,#42021),
(#42022,#42023)),.UNSPECIFIED.,.F.,.F.,.F.,(3,3),(2,2),(0.,1.),(0.,0.0999999999999996),
 .UNSPECIFIED.);
#1448=B_SPLINE_SURFACE_WITH_KNOTS('',2,1,((#42029,#42030),(#42031,#42032),
(#42033,#42034)),.UNSPECIFIED.,.F.,.F.,.F.,(3,3),(2,2),(0.,1.),(0.,0.0999999999999996),
 .UNSPECIFIED.);
#1449=B_SPLINE_SURFACE_WITH_KNOTS('',2,1,((#42040,#42041),(#42042,#42043),
(#42044,#42045)),.UNSPECIFIED.,.F.,.F.,.F.,(3,3),(2,2),(0.,1.),(0.,0.0999999999999996),
 .UNSPECIFIED.);
#1450=B_SPLINE_SURFACE_WITH_KNOTS('',2,1,((#42051,#42052),(#42053,#42054),
(#42055,#42056)),.UNSPECIFIED.,.F.,.F.,.F.,(3,3),(2,2),(0.,1.),(0.,0.0999999999999996),
 .UNSPECIFIED.);
#1451=B_SPLINE_SURFACE_WITH_KNOTS('',2,1,((#42062,#42063),(#42064,#42065),
(#42066,#42067)),.UNSPECIFIED.,.F.,.F.,.F.,(3,3),(2,2),(0.,1.),(0.,0.0999999999999996),
 .UNSPECIFIED.);
#1452=B_SPLINE_SURFACE_WITH_KNOTS('',2,1,((#42073,#42074),(#42075,#42076),
(#42077,#42078)),.UNSPECIFIED.,.F.,.F.,.F.,(3,3),(2,2),(0.,1.),(0.,0.0999999999999996),
 .UNSPECIFIED.);
#1453=B_SPLINE_SURFACE_WITH_KNOTS('',2,1,((#42084,#42085),(#42086,#42087),
(#42088,#42089)),.UNSPECIFIED.,.F.,.F.,.F.,(3,3),(2,2),(0.,1.),(0.,0.0999999999999996),
 .UNSPECIFIED.);
#1532=CYLINDRICAL_SURFACE('',#28711,0.875);
#1533=CYLINDRICAL_SURFACE('',#28715,0.875);
#1534=CYLINDRICAL_SURFACE('',#28719,0.875);
#1535=CYLINDRICAL_SURFACE('',#28723,0.875);
#1536=CYLINDRICAL_SURFACE('',#28741,0.875);
#1537=CYLINDRICAL_SURFACE('',#28745,0.875);
#1538=CYLINDRICAL_SURFACE('',#28749,0.875);
#1539=CYLINDRICAL_SURFACE('',#28753,0.875);
#1540=CYLINDRICAL_SURFACE('',#28759,0.8);
#1541=CYLINDRICAL_SURFACE('',#28762,1.8);
#1542=CYLINDRICAL_SURFACE('',#28789,0.8);
#1543=CYLINDRICAL_SURFACE('',#28792,0.8);
#1544=CYLINDRICAL_SURFACE('',#28825,1.8);
#1545=CYLINDRICAL_SURFACE('',#28831,1.8);
#1546=CYLINDRICAL_SURFACE('',#28846,0.4);
#1547=CYLINDRICAL_SURFACE('',#28849,0.4);
#1548=CYLINDRICAL_SURFACE('',#28867,0.4);
#1549=CYLINDRICAL_SURFACE('',#28869,0.4);
#1550=CYLINDRICAL_SURFACE('',#28875,1.8);
#1551=CYLINDRICAL_SURFACE('',#28895,0.8);
#1552=CYLINDRICAL_SURFACE('',#28898,0.8);
#1553=CYLINDRICAL_SURFACE('',#28920,0.8);
#1554=CYLINDRICAL_SURFACE('',#28934,1.8);
#1555=CYLINDRICAL_SURFACE('',#28949,0.4);
#1556=CYLINDRICAL_SURFACE('',#28952,0.4);
#1557=CYLINDRICAL_SURFACE('',#28969,0.4);
#1558=CYLINDRICAL_SURFACE('',#28971,0.4);
#1559=CYLINDRICAL_SURFACE('',#28976,1.8);
#1560=CYLINDRICAL_SURFACE('',#28983,1.8);
#1561=CYLINDRICAL_SURFACE('',#28990,1.8);
#1562=CYLINDRICAL_SURFACE('',#28997,0.504999999999999);
#1563=CYLINDRICAL_SURFACE('',#29007,0.504999999999999);
#1564=CYLINDRICAL_SURFACE('',#29042,0.8);
#1565=CYLINDRICAL_SURFACE('',#29044,0.8);
#1874=FACE_BOUND('',#4567,.T.);
#1875=FACE_BOUND('',#4568,.T.);
#1876=FACE_BOUND('',#4569,.T.);
#1877=FACE_BOUND('',#4570,.T.);
#1878=FACE_BOUND('',#4580,.T.);
#1879=FACE_BOUND('',#4581,.T.);
#1880=FACE_BOUND('',#4582,.T.);
#1881=FACE_BOUND('',#4583,.T.);
#1882=FACE_BOUND('',#4589,.T.);
#1883=FACE_BOUND('',#4590,.T.);
#1884=FACE_BOUND('',#4591,.T.);
#1885=FACE_BOUND('',#4592,.T.);
#1886=FACE_BOUND('',#4608,.T.);
#1887=FACE_BOUND('',#4609,.T.);
#1888=FACE_BOUND('',#4610,.T.);
#1889=FACE_BOUND('',#4611,.T.);
#1890=FACE_BOUND('',#4627,.T.);
#1891=FACE_BOUND('',#4638,.T.);
#1892=FACE_BOUND('',#4639,.T.);
#1893=FACE_BOUND('',#4640,.T.);
#1894=FACE_BOUND('',#4641,.T.);
#1895=FACE_BOUND('',#4642,.T.);
#1896=FACE_BOUND('',#4644,.T.);
#1897=FACE_BOUND('',#4711,.T.);
#1898=FACE_BOUND('',#4724,.T.);
#1899=FACE_BOUND('',#4787,.T.);
#1900=FACE_BOUND('',#4788,.T.);
#1901=FACE_BOUND('',#4791,.T.);
#1902=FACE_BOUND('',#4792,.T.);
#1903=FACE_BOUND('',#4815,.T.);
#1904=FACE_BOUND('',#4848,.T.);
#2045=CIRCLE('',#28705,0.975000000000001);
#2046=CIRCLE('',#28706,0.875);
#2047=CIRCLE('',#28708,0.975000000000001);
#2048=CIRCLE('',#28709,0.975000000000001);
#2049=CIRCLE('',#28710,0.975000000000001);
#2050=CIRCLE('',#28712,0.875);
#2051=CIRCLE('',#28714,0.875);
#2052=CIRCLE('',#28716,0.875);
#2053=CIRCLE('',#28718,0.875);
#2054=CIRCLE('',#28720,0.875);
#2055=CIRCLE('',#28722,0.875);
#2056=CIRCLE('',#28724,0.875);
#2057=CIRCLE('',#28726,0.975000000000001);
#2058=CIRCLE('',#28728,0.975000000000001);
#2059=CIRCLE('',#28729,0.975000000000001);
#2060=CIRCLE('',#28730,0.975000000000001);
#2061=CIRCLE('',#28735,0.975000000000001);
#2062=CIRCLE('',#28736,0.875);
#2063=CIRCLE('',#28738,0.975000000000001);
#2064=CIRCLE('',#28739,0.975000000000001);
#2065=CIRCLE('',#28740,0.975000000000001);
#2066=CIRCLE('',#28742,0.875);
#2067=CIRCLE('',#28744,0.875);
#2068=CIRCLE('',#28746,0.875);
#2069=CIRCLE('',#28748,0.875);
#2070=CIRCLE('',#28750,0.875);
#2071=CIRCLE('',#28752,0.875);
#2072=CIRCLE('',#28754,0.875);
#2073=CIRCLE('',#28756,1.8);
#2074=CIRCLE('',#28757,1.8);
#2075=CIRCLE('',#28758,1.9);
#2076=CIRCLE('',#28760,0.8);
#2077=CIRCLE('',#28761,0.8);
#2078=CIRCLE('',#28763,1.8);
#2079=CIRCLE('',#28764,1.8);
#2080=CIRCLE('',#28766,0.975000000000001);
#2081=CIRCLE('',#28768,0.975000000000001);
#2082=CIRCLE('',#28769,0.975000000000001);
#2083=CIRCLE('',#28770,0.975000000000001);
#2084=CIRCLE('',#28775,0.8);
#2085=CIRCLE('',#28776,0.700000000000011);
#2086=CIRCLE('',#28779,0.700000000000011);
#2087=CIRCLE('',#28782,0.8);
#2088=CIRCLE('',#28783,0.700000000000011);
#2089=CIRCLE('',#28786,0.8);
#2090=CIRCLE('',#28787,0.700000000000011);
#2091=CIRCLE('',#28790,0.8);
#2092=CIRCLE('',#28793,0.8);
#2093=CIRCLE('',#28795,0.499999999999985);
#2094=CIRCLE('',#28796,0.499999999999985);
#2095=CIRCLE('',#28797,0.499999999999985);
#2096=CIRCLE('',#28798,0.499999999999986);
#2097=CIRCLE('',#28800,0.700000000000011);
#2098=CIRCLE('',#28803,0.700000000000011);
#2099=CIRCLE('',#28806,0.8);
#2100=CIRCLE('',#28807,0.700000000000011);
#2101=CIRCLE('',#28810,0.700000000000011);
#2102=CIRCLE('',#28814,1.9);
#2103=CIRCLE('',#28815,1.9);
#2104=CIRCLE('',#28816,1.9);
#2105=CIRCLE('',#28818,0.499999999999986);
#2106=CIRCLE('',#28819,0.499999999999985);
#2107=CIRCLE('',#28820,0.499999999999985);
#2108=CIRCLE('',#28821,0.499999999999985);
#2109=CIRCLE('',#28823,1.8);
#2110=CIRCLE('',#28824,1.8);
#2111=CIRCLE('',#28826,1.8);
#2112=CIRCLE('',#28827,1.8);
#2113=CIRCLE('',#28829,1.8);
#2114=CIRCLE('',#28830,1.8);
#2115=CIRCLE('',#28832,1.8);
#2116=CIRCLE('',#28833,1.8);
#2117=CIRCLE('',#28836,0.4);
#2118=CIRCLE('',#28839,0.4);
#2119=CIRCLE('',#28842,0.4);
#2120=CIRCLE('',#28845,0.4);
#2121=CIRCLE('',#28847,0.4);
#2122=CIRCLE('',#28850,0.4);
#2123=CIRCLE('',#28852,1.9);
#2124=CIRCLE('',#28853,1.9);
#2125=CIRCLE('',#28854,1.9);
#2126=CIRCLE('',#28855,1.9);
#2127=CIRCLE('',#28859,0.4);
#2128=CIRCLE('',#28862,0.4);
#2129=CIRCLE('',#28873,1.8);
#2130=CIRCLE('',#28874,1.8);
#2131=CIRCLE('',#28876,1.8);
#2132=CIRCLE('',#28877,1.8);
#2133=CIRCLE('',#28880,0.8);
#2134=CIRCLE('',#28881,0.700000000000011);
#2135=CIRCLE('',#28884,0.8);
#2136=CIRCLE('',#28885,0.700000000000011);
#2137=CIRCLE('',#28888,0.8);
#2138=CIRCLE('',#28889,0.700000000000011);
#2139=CIRCLE('',#28892,0.8);
#2140=CIRCLE('',#28893,0.700000000000011);
#2141=CIRCLE('',#28896,0.8);
#2142=CIRCLE('',#28899,0.8);
#2143=CIRCLE('',#28901,0.499999999999986);
#2144=CIRCLE('',#28902,0.499999999999985);
#2145=CIRCLE('',#28903,0.499999999999985);
#2146=CIRCLE('',#28904,0.499999999999985);
#2147=CIRCLE('',#28906,0.700000000000011);
#2148=CIRCLE('',#28909,0.700000000000011);
#2149=CIRCLE('',#28912,0.8);
#2150=CIRCLE('',#28913,0.700000000000011);
#2151=CIRCLE('',#28916,0.8);
#2152=CIRCLE('',#28917,0.700000000000011);
#2153=CIRCLE('',#28922,1.9);
#2154=CIRCLE('',#28923,1.9);
#2155=CIRCLE('',#28924,1.9);
#2156=CIRCLE('',#28925,1.9);
#2157=CIRCLE('',#28927,0.499999999999985);
#2158=CIRCLE('',#28928,0.499999999999985);
#2159=CIRCLE('',#28929,0.499999999999985);
#2160=CIRCLE('',#28930,0.499999999999986);
#2161=CIRCLE('',#28932,1.8);
#2162=CIRCLE('',#28933,1.8);
#2163=CIRCLE('',#28935,1.8);
#2164=CIRCLE('',#28936,1.8);
#2165=CIRCLE('',#28939,0.4);
#2166=CIRCLE('',#28942,0.4);
#2167=CIRCLE('',#28945,0.4);
#2168=CIRCLE('',#28948,0.4);
#2169=CIRCLE('',#28950,0.4);
#2170=CIRCLE('',#28953,0.4);
#2171=CIRCLE('',#28955,1.9);
#2172=CIRCLE('',#28956,1.9);
#2173=CIRCLE('',#28957,1.9);
#2174=CIRCLE('',#28958,1.9);
#2175=CIRCLE('',#28965,0.4);
#2176=CIRCLE('',#28968,0.4);
#2177=CIRCLE('',#28974,1.8);
#2178=CIRCLE('',#28975,1.8);
#2179=CIRCLE('',#28977,1.8);
#2180=CIRCLE('',#28978,1.8);
#2181=CIRCLE('',#28981,1.8);
#2182=CIRCLE('',#28982,1.8);
#2183=CIRCLE('',#28984,1.8);
#2184=CIRCLE('',#28985,1.8);
#2185=CIRCLE('',#28988,1.8);
#2186=CIRCLE('',#28989,1.8);
#2187=CIRCLE('',#28991,1.8);
#2188=CIRCLE('',#28992,1.8);
#2189=CIRCLE('',#28995,0.605);
#2190=CIRCLE('',#28996,0.504999999999999);
#2191=CIRCLE('',#28998,0.504999999999999);
#2192=CIRCLE('',#29000,0.605);
#2193=CIRCLE('',#29002,0.605);
#2194=CIRCLE('',#29004,0.605);
#2195=CIRCLE('',#29006,0.504999999999999);
#2196=CIRCLE('',#29008,0.504999999999999);
#2731=CONICAL_SURFACE('',#28704,0.925000000000001,0.785398163397457);
#2732=CONICAL_SURFACE('',#28713,0.925000000000001,0.785398163397457);
#2733=CONICAL_SURFACE('',#28717,0.925000000000001,0.785398163397457);
#2734=CONICAL_SURFACE('',#28721,0.925000000000001,0.785398163397457);
#2735=CONICAL_SURFACE('',#28725,0.925000000000001,0.785398163397457);
#2736=CONICAL_SURFACE('',#28731,0.925000000000001,0.785398163397457);
#2737=CONICAL_SURFACE('',#28732,0.925000000000001,0.785398163397457);
#2738=CONICAL_SURFACE('',#28733,0.925000000000001,0.785398163397457);
#2739=CONICAL_SURFACE('',#28734,0.925000000000001,0.785398163397457);
#2740=CONICAL_SURFACE('',#28743,0.925000000000001,0.785398163397457);
#2741=CONICAL_SURFACE('',#28747,0.925000000000001,0.785398163397457);
#2742=CONICAL_SURFACE('',#28751,0.925000000000001,0.785398163397457);
#2743=CONICAL_SURFACE('',#28755,1.85,0.785398163397422);
#2744=CONICAL_SURFACE('',#28765,0.925000000000001,0.785398163397457);
#2745=CONICAL_SURFACE('',#28771,0.925000000000001,0.785398163397457);
#2746=CONICAL_SURFACE('',#28772,0.925000000000001,0.785398163397457);
#2747=CONICAL_SURFACE('',#28773,0.925000000000001,0.785398163397457);
#2748=CONICAL_SURFACE('',#28774,0.750000000000006,0.78539816339742);
#2749=CONICAL_SURFACE('',#28778,0.750000000000006,0.78539816339742);
#2750=CONICAL_SURFACE('',#28781,0.750000000000006,0.78539816339742);
#2751=CONICAL_SURFACE('',#28785,0.750000000000005,0.785398163397422);
#2752=CONICAL_SURFACE('',#28799,0.750000000000006,0.785398163397384);
#2753=CONICAL_SURFACE('',#28802,0.750000000000005,0.785398163397387);
#2754=CONICAL_SURFACE('',#28805,0.750000000000006,0.785398163397384);
#2755=CONICAL_SURFACE('',#28809,0.750000000000006,0.785398163397384);
#2756=CONICAL_SURFACE('',#28822,1.85,0.785398163397422);
#2757=CONICAL_SURFACE('',#28828,1.85,0.785398163397422);
#2758=CONICAL_SURFACE('',#28835,0.449999999999992,0.785398163397365);
#2759=CONICAL_SURFACE('',#28838,0.449999999999993,0.785398163397367);
#2760=CONICAL_SURFACE('',#28841,0.449999999999993,0.785398163397367);
#2761=CONICAL_SURFACE('',#28844,0.449999999999993,0.785398163397371);
#2762=CONICAL_SURFACE('',#28856,1.85,0.785398163397422);
#2763=CONICAL_SURFACE('',#28858,0.449999999999992,0.785398163397401);
#2764=CONICAL_SURFACE('',#28861,0.449999999999993,0.785398163397403);
#2765=CONICAL_SURFACE('',#28864,0.449999999999993,0.785398163397403);
#2766=CONICAL_SURFACE('',#28866,0.449999999999993,0.785398163397406);
#2767=CONICAL_SURFACE('',#28870,1.85,0.785398163397422);
#2768=CONICAL_SURFACE('',#28871,1.85,0.785398163397422);
#2769=CONICAL_SURFACE('',#28872,1.85,0.785398163397422);
#2770=CONICAL_SURFACE('',#28878,1.85,0.785398163397422);
#2771=CONICAL_SURFACE('',#28879,0.750000000000006,0.785398163397384);
#2772=CONICAL_SURFACE('',#28883,0.750000000000006,0.785398163397384);
#2773=CONICAL_SURFACE('',#28887,0.750000000000005,0.785398163397387);
#2774=CONICAL_SURFACE('',#28891,0.750000000000006,0.785398163397384);
#2775=CONICAL_SURFACE('',#28905,0.750000000000006,0.78539816339742);
#2776=CONICAL_SURFACE('',#28908,0.750000000000006,0.78539816339742);
#2777=CONICAL_SURFACE('',#28911,0.750000000000005,0.785398163397422);
#2778=CONICAL_SURFACE('',#28915,0.750000000000006,0.78539816339742);
#2779=CONICAL_SURFACE('',#28931,1.85,0.785398163397422);
#2780=CONICAL_SURFACE('',#28938,0.449999999999992,0.785398163397401);
#2781=CONICAL_SURFACE('',#28941,0.449999999999993,0.785398163397403);
#2782=CONICAL_SURFACE('',#28944,0.449999999999993,0.785398163397403);
#2783=CONICAL_SURFACE('',#28947,0.449999999999993,0.785398163397406);
#2784=CONICAL_SURFACE('',#28960,0.449999999999992,0.785398163397365);
#2785=CONICAL_SURFACE('',#28962,0.449999999999993,0.785398163397367);
#2786=CONICAL_SURFACE('',#28964,0.449999999999993,0.785398163397367);
#2787=CONICAL_SURFACE('',#28967,0.449999999999993,0.785398163397371);
#2788=CONICAL_SURFACE('',#28972,1.85,0.785398163397422);
#2789=CONICAL_SURFACE('',#28973,1.85,0.785398163397422);
#2790=CONICAL_SURFACE('',#28979,1.85,0.785398163397422);
#2791=CONICAL_SURFACE('',#28980,1.85,0.785398163397422);
#2792=CONICAL_SURFACE('',#28986,1.85,0.785398163397422);
#2793=CONICAL_SURFACE('',#28987,1.85,0.785398163397422);
#2794=CONICAL_SURFACE('',#28993,1.85,0.785398163397422);
#2795=CONICAL_SURFACE('',#28994,0.555,0.785398163397484);
#2796=CONICAL_SURFACE('',#29001,0.555,0.785398163397484);
#2797=CONICAL_SURFACE('',#29005,0.555,0.785398163397484);
#2798=CONICAL_SURFACE('',#29009,0.555,0.785398163397484);
#2971=FACE_OUTER_BOUND('',#4551,.T.);
#2972=FACE_OUTER_BOUND('',#4552,.T.);
#2973=FACE_OUTER_BOUND('',#4553,.T.);
#2974=FACE_OUTER_BOUND('',#4554,.T.);
#2975=FACE_OUTER_BOUND('',#4555,.T.);
#2976=FACE_OUTER_BOUND('',#4556,.T.);
#2977=FACE_OUTER_BOUND('',#4557,.T.);
#2978=FACE_OUTER_BOUND('',#4558,.T.);
#2979=FACE_OUTER_BOUND('',#4559,.T.);
#2980=FACE_OUTER_BOUND('',#4560,.T.);
#2981=FACE_OUTER_BOUND('',#4561,.T.);
#2982=FACE_OUTER_BOUND('',#4562,.T.);
#2983=FACE_OUTER_BOUND('',#4563,.T.);
#2984=FACE_OUTER_BOUND('',#4564,.T.);
#2985=FACE_OUTER_BOUND('',#4565,.T.);
#2986=FACE_OUTER_BOUND('',#4566,.T.);
#2987=FACE_OUTER_BOUND('',#4571,.T.);
#2988=FACE_OUTER_BOUND('',#4572,.T.);
#2989=FACE_OUTER_BOUND('',#4573,.T.);
#2990=FACE_OUTER_BOUND('',#4574,.T.);
#2991=FACE_OUTER_BOUND('',#4575,.T.);
#2992=FACE_OUTER_BOUND('',#4576,.T.);
#2993=FACE_OUTER_BOUND('',#4577,.T.);
#2994=FACE_OUTER_BOUND('',#4578,.T.);
#2995=FACE_OUTER_BOUND('',#4579,.T.);
#2996=FACE_OUTER_BOUND('',#4584,.T.);
#2997=FACE_OUTER_BOUND('',#4585,.T.);
#2998=FACE_OUTER_BOUND('',#4586,.T.);
#2999=FACE_OUTER_BOUND('',#4587,.T.);
#3000=FACE_OUTER_BOUND('',#4588,.T.);
#3001=FACE_OUTER_BOUND('',#4593,.T.);
#3002=FACE_OUTER_BOUND('',#4594,.T.);
#3003=FACE_OUTER_BOUND('',#4595,.T.);
#3004=FACE_OUTER_BOUND('',#4596,.T.);
#3005=FACE_OUTER_BOUND('',#4597,.T.);
#3006=FACE_OUTER_BOUND('',#4598,.T.);
#3007=FACE_OUTER_BOUND('',#4599,.T.);
#3008=FACE_OUTER_BOUND('',#4600,.T.);
#3009=FACE_OUTER_BOUND('',#4601,.T.);
#3010=FACE_OUTER_BOUND('',#4602,.T.);
#3011=FACE_OUTER_BOUND('',#4603,.T.);
#3012=FACE_OUTER_BOUND('',#4604,.T.);
#3013=FACE_OUTER_BOUND('',#4605,.T.);
#3014=FACE_OUTER_BOUND('',#4606,.T.);
#3015=FACE_OUTER_BOUND('',#4607,.T.);
#3016=FACE_OUTER_BOUND('',#4612,.T.);
#3017=FACE_OUTER_BOUND('',#4613,.T.);
#3018=FACE_OUTER_BOUND('',#4614,.T.);
#3019=FACE_OUTER_BOUND('',#4615,.T.);
#3020=FACE_OUTER_BOUND('',#4616,.T.);
#3021=FACE_OUTER_BOUND('',#4617,.T.);
#3022=FACE_OUTER_BOUND('',#4618,.T.);
#3023=FACE_OUTER_BOUND('',#4619,.T.);
#3024=FACE_OUTER_BOUND('',#4620,.T.);
#3025=FACE_OUTER_BOUND('',#4621,.T.);
#3026=FACE_OUTER_BOUND('',#4622,.T.);
#3027=FACE_OUTER_BOUND('',#4623,.T.);
#3028=FACE_OUTER_BOUND('',#4624,.T.);
#3029=FACE_OUTER_BOUND('',#4625,.T.);
#3030=FACE_OUTER_BOUND('',#4626,.T.);
#3031=FACE_OUTER_BOUND('',#4628,.T.);
#3032=FACE_OUTER_BOUND('',#4629,.T.);
#3033=FACE_OUTER_BOUND('',#4630,.T.);
#3034=FACE_OUTER_BOUND('',#4631,.T.);
#3035=FACE_OUTER_BOUND('',#4632,.T.);
#3036=FACE_OUTER_BOUND('',#4633,.T.);
#3037=FACE_OUTER_BOUND('',#4634,.T.);
#3038=FACE_OUTER_BOUND('',#4635,.T.);
#3039=FACE_OUTER_BOUND('',#4636,.T.);
#3040=FACE_OUTER_BOUND('',#4637,.T.);
#3041=FACE_OUTER_BOUND('',#4643,.T.);
#3042=FACE_OUTER_BOUND('',#4645,.T.);
#3043=FACE_OUTER_BOUND('',#4646,.T.);
#3044=FACE_OUTER_BOUND('',#4647,.T.);
#3045=FACE_OUTER_BOUND('',#4648,.T.);
#3046=FACE_OUTER_BOUND('',#4649,.T.);
#3047=FACE_OUTER_BOUND('',#4650,.T.);
#3048=FACE_OUTER_BOUND('',#4651,.T.);
#3049=FACE_OUTER_BOUND('',#4652,.T.);
#3050=FACE_OUTER_BOUND('',#4653,.T.);
#3051=FACE_OUTER_BOUND('',#4654,.T.);
#3052=FACE_OUTER_BOUND('',#4655,.T.);
#3053=FACE_OUTER_BOUND('',#4656,.T.);
#3054=FACE_OUTER_BOUND('',#4657,.T.);
#3055=FACE_OUTER_BOUND('',#4658,.T.);
#3056=FACE_OUTER_BOUND('',#4659,.T.);
#3057=FACE_OUTER_BOUND('',#4660,.T.);
#3058=FACE_OUTER_BOUND('',#4661,.T.);
#3059=FACE_OUTER_BOUND('',#4662,.T.);
#3060=FACE_OUTER_BOUND('',#4663,.T.);
#3061=FACE_OUTER_BOUND('',#4664,.T.);
#3062=FACE_OUTER_BOUND('',#4665,.T.);
#3063=FACE_OUTER_BOUND('',#4666,.T.);
#3064=FACE_OUTER_BOUND('',#4667,.T.);
#3065=FACE_OUTER_BOUND('',#4668,.T.);
#3066=FACE_OUTER_BOUND('',#4669,.T.);
#3067=FACE_OUTER_BOUND('',#4670,.T.);
#3068=FACE_OUTER_BOUND('',#4671,.T.);
#3069=FACE_OUTER_BOUND('',#4672,.T.);
#3070=FACE_OUTER_BOUND('',#4673,.T.);
#3071=FACE_OUTER_BOUND('',#4674,.T.);
#3072=FACE_OUTER_BOUND('',#4675,.T.);
#3073=FACE_OUTER_BOUND('',#4676,.T.);
#3074=FACE_OUTER_BOUND('',#4677,.T.);
#3075=FACE_OUTER_BOUND('',#4678,.T.);
#3076=FACE_OUTER_BOUND('',#4679,.T.);
#3077=FACE_OUTER_BOUND('',#4680,.T.);
#3078=FACE_OUTER_BOUND('',#4681,.T.);
#3079=FACE_OUTER_BOUND('',#4682,.T.);
#3080=FACE_OUTER_BOUND('',#4683,.T.);
#3081=FACE_OUTER_BOUND('',#4684,.T.);
#3082=FACE_OUTER_BOUND('',#4685,.T.);
#3083=FACE_OUTER_BOUND('',#4686,.T.);
#3084=FACE_OUTER_BOUND('',#4687,.T.);
#3085=FACE_OUTER_BOUND('',#4688,.T.);
#3086=FACE_OUTER_BOUND('',#4689,.T.);
#3087=FACE_OUTER_BOUND('',#4690,.T.);
#3088=FACE_OUTER_BOUND('',#4691,.T.);
#3089=FACE_OUTER_BOUND('',#4692,.T.);
#3090=FACE_OUTER_BOUND('',#4693,.T.);
#3091=FACE_OUTER_BOUND('',#4694,.T.);
#3092=FACE_OUTER_BOUND('',#4695,.T.);
#3093=FACE_OUTER_BOUND('',#4696,.T.);
#3094=FACE_OUTER_BOUND('',#4697,.T.);
#3095=FACE_OUTER_BOUND('',#4698,.T.);
#3096=FACE_OUTER_BOUND('',#4699,.T.);
#3097=FACE_OUTER_BOUND('',#4700,.T.);
#3098=FACE_OUTER_BOUND('',#4701,.T.);
#3099=FACE_OUTER_BOUND('',#4702,.T.);
#3100=FACE_OUTER_BOUND('',#4703,.T.);
#3101=FACE_OUTER_BOUND('',#4704,.T.);
#3102=FACE_OUTER_BOUND('',#4705,.T.);
#3103=FACE_OUTER_BOUND('',#4706,.T.);
#3104=FACE_OUTER_BOUND('',#4707,.T.);
#3105=FACE_OUTER_BOUND('',#4708,.T.);
#3106=FACE_OUTER_BOUND('',#4709,.T.);
#3107=FACE_OUTER_BOUND('',#4710,.T.);
#3108=FACE_OUTER_BOUND('',#4712,.T.);
#3109=FACE_OUTER_BOUND('',#4713,.T.);
#3110=FACE_OUTER_BOUND('',#4714,.T.);
#3111=FACE_OUTER_BOUND('',#4715,.T.);
#3112=FACE_OUTER_BOUND('',#4716,.T.);
#3113=FACE_OUTER_BOUND('',#4717,.T.);
#3114=FACE_OUTER_BOUND('',#4718,.T.);
#3115=FACE_OUTER_BOUND('',#4719,.T.);
#3116=FACE_OUTER_BOUND('',#4720,.T.);
#3117=FACE_OUTER_BOUND('',#4721,.T.);
#3118=FACE_OUTER_BOUND('',#4722,.T.);
#3119=FACE_OUTER_BOUND('',#4723,.T.);
#3120=FACE_OUTER_BOUND('',#4725,.T.);
#3121=FACE_OUTER_BOUND('',#4726,.T.);
#3122=FACE_OUTER_BOUND('',#4727,.T.);
#3123=FACE_OUTER_BOUND('',#4728,.T.);
#3124=FACE_OUTER_BOUND('',#4729,.T.);
#3125=FACE_OUTER_BOUND('',#4730,.T.);
#3126=FACE_OUTER_BOUND('',#4731,.T.);
#3127=FACE_OUTER_BOUND('',#4732,.T.);
#3128=FACE_OUTER_BOUND('',#4733,.T.);
#3129=FACE_OUTER_BOUND('',#4734,.T.);
#3130=FACE_OUTER_BOUND('',#4735,.T.);
#3131=FACE_OUTER_BOUND('',#4736,.T.);
#3132=FACE_OUTER_BOUND('',#4737,.T.);
#3133=FACE_OUTER_BOUND('',#4738,.T.);
#3134=FACE_OUTER_BOUND('',#4739,.T.);
#3135=FACE_OUTER_BOUND('',#4740,.T.);
#3136=FACE_OUTER_BOUND('',#4741,.T.);
#3137=FACE_OUTER_BOUND('',#4742,.T.);
#3138=FACE_OUTER_BOUND('',#4743,.T.);
#3139=FACE_OUTER_BOUND('',#4744,.T.);
#3140=FACE_OUTER_BOUND('',#4745,.T.);
#3141=FACE_OUTER_BOUND('',#4746,.T.);
#3142=FACE_OUTER_BOUND('',#4747,.T.);
#3143=FACE_OUTER_BOUND('',#4748,.T.);
#3144=FACE_OUTER_BOUND('',#4749,.T.);
#3145=FACE_OUTER_BOUND('',#4750,.T.);
#3146=FACE_OUTER_BOUND('',#4751,.T.);
#3147=FACE_OUTER_BOUND('',#4752,.T.);
#3148=FACE_OUTER_BOUND('',#4753,.T.);
#3149=FACE_OUTER_BOUND('',#4754,.T.);
#3150=FACE_OUTER_BOUND('',#4755,.T.);
#3151=FACE_OUTER_BOUND('',#4756,.T.);
#3152=FACE_OUTER_BOUND('',#4757,.T.);
#3153=FACE_OUTER_BOUND('',#4758,.T.);
#3154=FACE_OUTER_BOUND('',#4759,.T.);
#3155=FACE_OUTER_BOUND('',#4760,.T.);
#3156=FACE_OUTER_BOUND('',#4761,.T.);
#3157=FACE_OUTER_BOUND('',#4762,.T.);
#3158=FACE_OUTER_BOUND('',#4763,.T.);
#3159=FACE_OUTER_BOUND('',#4764,.T.);
#3160=FACE_OUTER_BOUND('',#4765,.T.);
#3161=FACE_OUTER_BOUND('',#4766,.T.);
#3162=FACE_OUTER_BOUND('',#4767,.T.);
#3163=FACE_OUTER_BOUND('',#4768,.T.);
#3164=FACE_OUTER_BOUND('',#4769,.T.);
#3165=FACE_OUTER_BOUND('',#4770,.T.);
#3166=FACE_OUTER_BOUND('',#4771,.T.);
#3167=FACE_OUTER_BOUND('',#4772,.T.);
#3168=FACE_OUTER_BOUND('',#4773,.T.);
#3169=FACE_OUTER_BOUND('',#4774,.T.);
#3170=FACE_OUTER_BOUND('',#4775,.T.);
#3171=FACE_OUTER_BOUND('',#4776,.T.);
#3172=FACE_OUTER_BOUND('',#4777,.T.);
#3173=FACE_OUTER_BOUND('',#4778,.T.);
#3174=FACE_OUTER_BOUND('',#4779,.T.);
#3175=FACE_OUTER_BOUND('',#4780,.T.);
#3176=FACE_OUTER_BOUND('',#4781,.T.);
#3177=FACE_OUTER_BOUND('',#4782,.T.);
#3178=FACE_OUTER_BOUND('',#4783,.T.);
#3179=FACE_OUTER_BOUND('',#4784,.T.);
#3180=FACE_OUTER_BOUND('',#4785,.T.);
#3181=FACE_OUTER_BOUND('',#4786,.T.);
#3182=FACE_OUTER_BOUND('',#4789,.T.);
#3183=FACE_OUTER_BOUND('',#4790,.T.);
#3184=FACE_OUTER_BOUND('',#4793,.T.);
#3185=FACE_OUTER_BOUND('',#4794,.T.);
#3186=FACE_OUTER_BOUND('',#4795,.T.);
#3187=FACE_OUTER_BOUND('',#4796,.T.);
#3188=FACE_OUTER_BOUND('',#4797,.T.);
#3189=FACE_OUTER_BOUND('',#4798,.T.);
#3190=FACE_OUTER_BOUND('',#4799,.T.);
#3191=FACE_OUTER_BOUND('',#4800,.T.);
#3192=FACE_OUTER_BOUND('',#4801,.T.);
#3193=FACE_OUTER_BOUND('',#4802,.T.);
#3194=FACE_OUTER_BOUND('',#4803,.T.);
#3195=FACE_OUTER_BOUND('',#4804,.T.);
#3196=FACE_OUTER_BOUND('',#4805,.T.);
#3197=FACE_OUTER_BOUND('',#4806,.T.);
#3198=FACE_OUTER_BOUND('',#4807,.T.);
#3199=FACE_OUTER_BOUND('',#4808,.T.);
#3200=FACE_OUTER_BOUND('',#4809,.T.);
#3201=FACE_OUTER_BOUND('',#4810,.T.);
#3202=FACE_OUTER_BOUND('',#4811,.T.);
#3203=FACE_OUTER_BOUND('',#4812,.T.);
#3204=FACE_OUTER_BOUND('',#4813,.T.);
#3205=FACE_OUTER_BOUND('',#4814,.T.);
#3206=FACE_OUTER_BOUND('',#4816,.T.);
#3207=FACE_OUTER_BOUND('',#4817,.T.);
#3208=FACE_OUTER_BOUND('',#4818,.T.);
#3209=FACE_OUTER_BOUND('',#4819,.T.);
#3210=FACE_OUTER_BOUND('',#4820,.T.);
#3211=FACE_OUTER_BOUND('',#4821,.T.);
#3212=FACE_OUTER_BOUND('',#4822,.T.);
#3213=FACE_OUTER_BOUND('',#4823,.T.);
#3214=FACE_OUTER_BOUND('',#4824,.T.);
#3215=FACE_OUTER_BOUND('',#4825,.T.);
#3216=FACE_OUTER_BOUND('',#4826,.T.);
#3217=FACE_OUTER_BOUND('',#4827,.T.);
#3218=FACE_OUTER_BOUND('',#4828,.T.);
#3219=FACE_OUTER_BOUND('',#4829,.T.);
#3220=FACE_OUTER_BOUND('',#4830,.T.);
#3221=FACE_OUTER_BOUND('',#4831,.T.);
#3222=FACE_OUTER_BOUND('',#4832,.T.);
#3223=FACE_OUTER_BOUND('',#4833,.T.);
#3224=FACE_OUTER_BOUND('',#4834,.T.);
#3225=FACE_OUTER_BOUND('',#4835,.T.);
#3226=FACE_OUTER_BOUND('',#4836,.T.);
#3227=FACE_OUTER_BOUND('',#4837,.T.);
#3228=FACE_OUTER_BOUND('',#4838,.T.);
#3229=FACE_OUTER_BOUND('',#4839,.T.);
#3230=FACE_OUTER_BOUND('',#4840,.T.);
#3231=FACE_OUTER_BOUND('',#4841,.T.);
#3232=FACE_OUTER_BOUND('',#4842,.T.);
#3233=FACE_OUTER_BOUND('',#4843,.T.);
#3234=FACE_OUTER_BOUND('',#4844,.T.);
#3235=FACE_OUTER_BOUND('',#4845,.T.);
#3236=FACE_OUTER_BOUND('',#4846,.T.);
#3237=FACE_OUTER_BOUND('',#4847,.T.);
#3238=FACE_OUTER_BOUND('',#4849,.T.);
#3239=FACE_OUTER_BOUND('',#4850,.T.);
#3240=FACE_OUTER_BOUND('',#4851,.T.);
#3241=FACE_OUTER_BOUND('',#4852,.T.);
#3242=FACE_OUTER_BOUND('',#4853,.T.);
#3243=FACE_OUTER_BOUND('',#4854,.T.);
#3244=FACE_OUTER_BOUND('',#4855,.T.);
#3245=FACE_OUTER_BOUND('',#4856,.T.);
#3246=FACE_OUTER_BOUND('',#4857,.T.);
#3247=FACE_OUTER_BOUND('',#4858,.T.);
#3248=FACE_OUTER_BOUND('',#4859,.T.);
#3249=FACE_OUTER_BOUND('',#4860,.T.);
#3250=FACE_OUTER_BOUND('',#4861,.T.);
#3251=FACE_OUTER_BOUND('',#4862,.T.);
#3252=FACE_OUTER_BOUND('',#4863,.T.);
#3253=FACE_OUTER_BOUND('',#4864,.T.);
#3254=FACE_OUTER_BOUND('',#4865,.T.);
#3255=FACE_OUTER_BOUND('',#4866,.T.);
#3256=FACE_OUTER_BOUND('',#4867,.T.);
#3257=FACE_OUTER_BOUND('',#4868,.T.);
#3258=FACE_OUTER_BOUND('',#4869,.T.);
#3259=FACE_OUTER_BOUND('',#4870,.T.);
#3260=FACE_OUTER_BOUND('',#4871,.T.);
#3261=FACE_OUTER_BOUND('',#4872,.T.);
#3262=FACE_OUTER_BOUND('',#4873,.T.);
#3263=FACE_OUTER_BOUND('',#4874,.T.);
#3264=FACE_OUTER_BOUND('',#4875,.T.);
#3265=FACE_OUTER_BOUND('',#4876,.T.);
#3266=FACE_OUTER_BOUND('',#4877,.T.);
#3267=FACE_OUTER_BOUND('',#4878,.T.);
#3268=FACE_OUTER_BOUND('',#4879,.T.);
#3269=FACE_OUTER_BOUND('',#4880,.T.);
#3270=FACE_OUTER_BOUND('',#4881,.T.);
#3271=FACE_OUTER_BOUND('',#4882,.T.);
#3272=FACE_OUTER_BOUND('',#4883,.T.);
#3273=FACE_OUTER_BOUND('',#4884,.T.);
#3274=FACE_OUTER_BOUND('',#4885,.T.);
#3275=FACE_OUTER_BOUND('',#4886,.T.);
#3276=FACE_OUTER_BOUND('',#4887,.T.);
#3277=FACE_OUTER_BOUND('',#4888,.T.);
#3278=FACE_OUTER_BOUND('',#4889,.T.);
#3279=FACE_OUTER_BOUND('',#4890,.T.);
#4551=EDGE_LOOP('',(#17919,#17920,#17921,#17922,#17923));
#4552=EDGE_LOOP('',(#17924,#17925,#17926,#17927,#17928,#17929));
#4553=EDGE_LOOP('',(#17930,#17931,#17932,#17933));
#4554=EDGE_LOOP('',(#17934,#17935,#17936,#17937));
#4555=EDGE_LOOP('',(#17938,#17939,#17940,#17941,#17942));
#4556=EDGE_LOOP('',(#17943,#17944,#17945,#17946,#17947,#17948));
#4557=EDGE_LOOP('',(#17949,#17950,#17951,#17952,#17953,#17954,#17955,#17956));
#4558=EDGE_LOOP('',(#17957,#17958,#17959,#17960,#17961));
#4559=EDGE_LOOP('',(#17962,#17963,#17964,#17965));
#4560=EDGE_LOOP('',(#17966,#17967,#17968,#17969,#17970,#17971));
#4561=EDGE_LOOP('',(#17972,#17973,#17974,#17975,#17976,#17977));
#4562=EDGE_LOOP('',(#17978,#17979,#17980,#17981));
#4563=EDGE_LOOP('',(#17982,#17983,#17984,#17985));
#4564=EDGE_LOOP('',(#17986,#17987,#17988,#17989,#17990));
#4565=EDGE_LOOP('',(#17991,#17992,#17993,#17994));
#4566=EDGE_LOOP('',(#17995,#17996,#17997,#17998));
#4567=EDGE_LOOP('',(#17999));
#4568=EDGE_LOOP('',(#18000));
#4569=EDGE_LOOP('',(#18001));
#4570=EDGE_LOOP('',(#18002));
#4571=EDGE_LOOP('',(#18003,#18004,#18005,#18006));
#4572=EDGE_LOOP('',(#18007,#18008,#18009,#18010));
#4573=EDGE_LOOP('',(#18011,#18012,#18013,#18014));
#4574=EDGE_LOOP('',(#18015,#18016,#18017,#18018));
#4575=EDGE_LOOP('',(#18019,#18020,#18021,#18022));
#4576=EDGE_LOOP('',(#18023,#18024,#18025,#18026));
#4577=EDGE_LOOP('',(#18027,#18028,#18029,#18030));
#4578=EDGE_LOOP('',(#18031,#18032,#18033,#18034));
#4579=EDGE_LOOP('',(#18035,#18036,#18037,#18038));
#4580=EDGE_LOOP('',(#18039));
#4581=EDGE_LOOP('',(#18040));
#4582=EDGE_LOOP('',(#18041));
#4583=EDGE_LOOP('',(#18042));
#4584=EDGE_LOOP('',(#18043,#18044,#18045,#18046));
#4585=EDGE_LOOP('',(#18047,#18048,#18049,#18050));
#4586=EDGE_LOOP('',(#18051,#18052,#18053,#18054));
#4587=EDGE_LOOP('',(#18055,#18056,#18057,#18058));
#4588=EDGE_LOOP('',(#18059,#18060,#18061,#18062));
#4589=EDGE_LOOP('',(#18063));
#4590=EDGE_LOOP('',(#18064));
#4591=EDGE_LOOP('',(#18065));
#4592=EDGE_LOOP('',(#18066));
#4593=EDGE_LOOP('',(#18067,#18068,#18069,#18070));
#4594=EDGE_LOOP('',(#18071,#18072,#18073,#18074));
#4595=EDGE_LOOP('',(#18075,#18076,#18077,#18078));
#4596=EDGE_LOOP('',(#18079,#18080,#18081,#18082));
#4597=EDGE_LOOP('',(#18083,#18084,#18085,#18086));
#4598=EDGE_LOOP('',(#18087,#18088,#18089,#18090));
#4599=EDGE_LOOP('',(#18091,#18092,#18093,#18094));
#4600=EDGE_LOOP('',(#18095,#18096,#18097,#18098,#18099));
#4601=EDGE_LOOP('',(#18100,#18101,#18102,#18103));
#4602=EDGE_LOOP('',(#18104,#18105,#18106,#18107));
#4603=EDGE_LOOP('',(#18108,#18109,#18110,#18111));
#4604=EDGE_LOOP('',(#18112,#18113,#18114,#18115,#18116,#18117,#18118,#18119,
#18120,#18121,#18122,#18123));
#4605=EDGE_LOOP('',(#18124,#18125,#18126,#18127,#18128,#18129,#18130,#18131,
#18132,#18133,#18134,#18135));
#4606=EDGE_LOOP('',(#18136,#18137,#18138,#18139));
#4607=EDGE_LOOP('',(#18140,#18141,#18142,#18143));
#4608=EDGE_LOOP('',(#18144));
#4609=EDGE_LOOP('',(#18145));
#4610=EDGE_LOOP('',(#18146));
#4611=EDGE_LOOP('',(#18147));
#4612=EDGE_LOOP('',(#18148,#18149,#18150,#18151));
#4613=EDGE_LOOP('',(#18152,#18153,#18154,#18155));
#4614=EDGE_LOOP('',(#18156,#18157,#18158,#18159));
#4615=EDGE_LOOP('',(#18160,#18161,#18162,#18163));
#4616=EDGE_LOOP('',(#18164,#18165,#18166,#18167));
#4617=EDGE_LOOP('',(#18168,#18169,#18170,#18171));
#4618=EDGE_LOOP('',(#18172,#18173,#18174,#18175));
#4619=EDGE_LOOP('',(#18176,#18177,#18178,#18179));
#4620=EDGE_LOOP('',(#18180,#18181,#18182,#18183));
#4621=EDGE_LOOP('',(#18184,#18185,#18186,#18187));
#4622=EDGE_LOOP('',(#18188,#18189,#18190,#18191));
#4623=EDGE_LOOP('',(#18192,#18193,#18194,#18195,#18196,#18197));
#4624=EDGE_LOOP('',(#18198,#18199,#18200,#18201));
#4625=EDGE_LOOP('',(#18202,#18203,#18204,#18205,#18206,#18207,#18208,#18209,
#18210,#18211,#18212,#18213,#18214,#18215));
#4626=EDGE_LOOP('',(#18216,#18217,#18218,#18219,#18220,#18221,#18222,#18223));
#4627=EDGE_LOOP('',(#18224,#18225,#18226,#18227,#18228,#18229,#18230,#18231));
#4628=EDGE_LOOP('',(#18232,#18233,#18234,#18235));
#4629=EDGE_LOOP('',(#18236,#18237,#18238,#18239));
#4630=EDGE_LOOP('',(#18240,#18241,#18242,#18243));
#4631=EDGE_LOOP('',(#18244,#18245,#18246,#18247));
#4632=EDGE_LOOP('',(#18248,#18249,#18250,#18251));
#4633=EDGE_LOOP('',(#18252,#18253,#18254,#18255));
#4634=EDGE_LOOP('',(#18256,#18257,#18258,#18259));
#4635=EDGE_LOOP('',(#18260,#18261,#18262,#18263));
#4636=EDGE_LOOP('',(#18264,#18265,#18266,#18267));
#4637=EDGE_LOOP('',(#18268,#18269,#18270,#18271,#18272,#18273,#18274,#18275,
#18276,#18277,#18278,#18279));
#4638=EDGE_LOOP('',(#18280,#18281,#18282,#18283,#18284,#18285,#18286,#18287,
#18288,#18289));
#4639=EDGE_LOOP('',(#18290,#18291,#18292,#18293,#18294,#18295,#18296,#18297));
#4640=EDGE_LOOP('',(#18298,#18299,#18300,#18301,#18302,#18303,#18304,#18305,
#18306,#18307,#18308,#18309,#18310));
#4641=EDGE_LOOP('',(#18311,#18312,#18313,#18314,#18315,#18316,#18317,#18318,
#18319,#18320,#18321,#18322,#18323,#18324,#18325,#18326,#18327,#18328,#18329,
#18330,#18331,#18332));
#4642=EDGE_LOOP('',(#18333,#18334,#18335,#18336,#18337,#18338,#18339,#18340,
#18341,#18342));
#4643=EDGE_LOOP('',(#18343,#18344,#18345,#18346,#18347,#18348,#18349,#18350));
#4644=EDGE_LOOP('',(#18351,#18352,#18353,#18354,#18355,#18356,#18357,#18358));
#4645=EDGE_LOOP('',(#18359,#18360,#18361,#18362,#18363));
#4646=EDGE_LOOP('',(#18364,#18365,#18366,#18367));
#4647=EDGE_LOOP('',(#18368,#18369,#18370,#18371));
#4648=EDGE_LOOP('',(#18372,#18373,#18374,#18375));
#4649=EDGE_LOOP('',(#18376,#18377,#18378,#18379,#18380,#18381,#18382,#18383,
#18384,#18385,#18386,#18387));
#4650=EDGE_LOOP('',(#18388,#18389,#18390,#18391,#18392));
#4651=EDGE_LOOP('',(#18393,#18394,#18395,#18396));
#4652=EDGE_LOOP('',(#18397,#18398,#18399,#18400));
#4653=EDGE_LOOP('',(#18401,#18402,#18403,#18404));
#4654=EDGE_LOOP('',(#18405,#18406,#18407,#18408,#18409,#18410,#18411,#18412,
#18413,#18414,#18415,#18416));
#4655=EDGE_LOOP('',(#18417,#18418,#18419,#18420));
#4656=EDGE_LOOP('',(#18421,#18422,#18423,#18424));
#4657=EDGE_LOOP('',(#18425,#18426,#18427,#18428));
#4658=EDGE_LOOP('',(#18429,#18430,#18431,#18432));
#4659=EDGE_LOOP('',(#18433,#18434,#18435,#18436));
#4660=EDGE_LOOP('',(#18437,#18438,#18439,#18440));
#4661=EDGE_LOOP('',(#18441,#18442,#18443,#18444));
#4662=EDGE_LOOP('',(#18445,#18446,#18447,#18448));
#4663=EDGE_LOOP('',(#18449,#18450,#18451,#18452));
#4664=EDGE_LOOP('',(#18453,#18454,#18455,#18456));
#4665=EDGE_LOOP('',(#18457,#18458,#18459,#18460,#18461,#18462,#18463,#18464,
#18465,#18466,#18467,#18468,#18469,#18470,#18471,#18472,#18473,#18474));
#4666=EDGE_LOOP('',(#18475,#18476,#18477,#18478,#18479,#18480,#18481,#18482,
#18483,#18484,#18485,#18486));
#4667=EDGE_LOOP('',(#18487,#18488,#18489,#18490,#18491,#18492));
#4668=EDGE_LOOP('',(#18493,#18494,#18495,#18496,#18497));
#4669=EDGE_LOOP('',(#18498,#18499,#18500,#18501,#18502));
#4670=EDGE_LOOP('',(#18503,#18504,#18505,#18506));
#4671=EDGE_LOOP('',(#18507,#18508,#18509,#18510));
#4672=EDGE_LOOP('',(#18511,#18512,#18513,#18514));
#4673=EDGE_LOOP('',(#18515,#18516,#18517,#18518));
#4674=EDGE_LOOP('',(#18519,#18520,#18521,#18522));
#4675=EDGE_LOOP('',(#18523,#18524,#18525,#18526));
#4676=EDGE_LOOP('',(#18527,#18528,#18529,#18530));
#4677=EDGE_LOOP('',(#18531,#18532,#18533,#18534));
#4678=EDGE_LOOP('',(#18535,#18536,#18537,#18538));
#4679=EDGE_LOOP('',(#18539,#18540,#18541,#18542));
#4680=EDGE_LOOP('',(#18543,#18544,#18545,#18546));
#4681=EDGE_LOOP('',(#18547,#18548,#18549,#18550,#18551,#18552,#18553,#18554,
#18555,#18556,#18557,#18558,#18559,#18560,#18561,#18562,#18563,#18564));
#4682=EDGE_LOOP('',(#18565,#18566,#18567,#18568,#18569,#18570));
#4683=EDGE_LOOP('',(#18571,#18572,#18573,#18574,#18575));
#4684=EDGE_LOOP('',(#18576,#18577,#18578,#18579,#18580));
#4685=EDGE_LOOP('',(#18581,#18582,#18583,#18584));
#4686=EDGE_LOOP('',(#18585,#18586,#18587,#18588,#18589,#18590));
#4687=EDGE_LOOP('',(#18591,#18592,#18593,#18594,#18595));
#4688=EDGE_LOOP('',(#18596,#18597,#18598,#18599,#18600));
#4689=EDGE_LOOP('',(#18601,#18602,#18603,#18604));
#4690=EDGE_LOOP('',(#18605,#18606,#18607,#18608,#18609));
#4691=EDGE_LOOP('',(#18610,#18611,#18612,#18613));
#4692=EDGE_LOOP('',(#18614,#18615,#18616,#18617));
#4693=EDGE_LOOP('',(#18618,#18619,#18620,#18621));
#4694=EDGE_LOOP('',(#18622,#18623,#18624,#18625,#18626,#18627,#18628,#18629,
#18630,#18631,#18632,#18633));
#4695=EDGE_LOOP('',(#18634,#18635,#18636,#18637,#18638,#18639));
#4696=EDGE_LOOP('',(#18640,#18641,#18642,#18643,#18644));
#4697=EDGE_LOOP('',(#18645,#18646,#18647,#18648,#18649));
#4698=EDGE_LOOP('',(#18650,#18651,#18652,#18653));
#4699=EDGE_LOOP('',(#18654,#18655,#18656,#18657));
#4700=EDGE_LOOP('',(#18658,#18659,#18660,#18661));
#4701=EDGE_LOOP('',(#18662,#18663,#18664,#18665));
#4702=EDGE_LOOP('',(#18666,#18667,#18668,#18669));
#4703=EDGE_LOOP('',(#18670,#18671,#18672,#18673));
#4704=EDGE_LOOP('',(#18674,#18675,#18676,#18677));
#4705=EDGE_LOOP('',(#18678,#18679,#18680,#18681));
#4706=EDGE_LOOP('',(#18682,#18683,#18684,#18685));
#4707=EDGE_LOOP('',(#18686,#18687,#18688,#18689,#18690,#18691));
#4708=EDGE_LOOP('',(#18692,#18693,#18694,#18695));
#4709=EDGE_LOOP('',(#18696,#18697,#18698,#18699,#18700,#18701,#18702,#18703,
#18704,#18705,#18706,#18707,#18708,#18709));
#4710=EDGE_LOOP('',(#18710,#18711,#18712,#18713,#18714,#18715,#18716,#18717));
#4711=EDGE_LOOP('',(#18718,#18719,#18720,#18721,#18722,#18723,#18724,#18725));
#4712=EDGE_LOOP('',(#18726,#18727,#18728,#18729));
#4713=EDGE_LOOP('',(#18730,#18731,#18732,#18733));
#4714=EDGE_LOOP('',(#18734,#18735,#18736,#18737));
#4715=EDGE_LOOP('',(#18738,#18739,#18740,#18741));
#4716=EDGE_LOOP('',(#18742,#18743,#18744,#18745));
#4717=EDGE_LOOP('',(#18746,#18747,#18748,#18749));
#4718=EDGE_LOOP('',(#18750,#18751,#18752,#18753));
#4719=EDGE_LOOP('',(#18754,#18755,#18756,#18757));
#4720=EDGE_LOOP('',(#18758,#18759,#18760,#18761));
#4721=EDGE_LOOP('',(#18762,#18763,#18764,#18765,#18766,#18767,#18768,#18769,
#18770,#18771,#18772,#18773));
#4722=EDGE_LOOP('',(#18774,#18775,#18776,#18777,#18778,#18779,#18780,#18781,
#18782,#18783,#18784,#18785));
#4723=EDGE_LOOP('',(#18786,#18787,#18788,#18789,#18790,#18791,#18792,#18793));
#4724=EDGE_LOOP('',(#18794,#18795,#18796,#18797,#18798,#18799,#18800,#18801));
#4725=EDGE_LOOP('',(#18802,#18803,#18804,#18805));
#4726=EDGE_LOOP('',(#18806,#18807,#18808,#18809,#18810));
#4727=EDGE_LOOP('',(#18811,#18812,#18813,#18814));
#4728=EDGE_LOOP('',(#18815,#18816,#18817,#18818));
#4729=EDGE_LOOP('',(#18819,#18820,#18821,#18822,#18823,#18824,#18825,#18826,
#18827,#18828,#18829,#18830));
#4730=EDGE_LOOP('',(#18831,#18832,#18833,#18834));
#4731=EDGE_LOOP('',(#18835,#18836,#18837,#18838));
#4732=EDGE_LOOP('',(#18839,#18840,#18841,#18842));
#4733=EDGE_LOOP('',(#18843,#18844,#18845,#18846));
#4734=EDGE_LOOP('',(#18847,#18848,#18849,#18850));
#4735=EDGE_LOOP('',(#18851,#18852,#18853,#18854));
#4736=EDGE_LOOP('',(#18855,#18856,#18857,#18858));
#4737=EDGE_LOOP('',(#18859,#18860,#18861,#18862));
#4738=EDGE_LOOP('',(#18863,#18864,#18865,#18866));
#4739=EDGE_LOOP('',(#18867,#18868,#18869,#18870));
#4740=EDGE_LOOP('',(#18871,#18872,#18873,#18874,#18875,#18876,#18877,#18878,
#18879,#18880,#18881,#18882,#18883,#18884,#18885,#18886,#18887));
#4741=EDGE_LOOP('',(#18888,#18889,#18890,#18891,#18892,#18893,#18894,#18895,
#18896,#18897,#18898,#18899));
#4742=EDGE_LOOP('',(#18900,#18901,#18902,#18903));
#4743=EDGE_LOOP('',(#18904,#18905,#18906,#18907));
#4744=EDGE_LOOP('',(#18908,#18909,#18910,#18911));
#4745=EDGE_LOOP('',(#18912,#18913,#18914,#18915));
#4746=EDGE_LOOP('',(#18916,#18917,#18918,#18919));
#4747=EDGE_LOOP('',(#18920,#18921,#18922,#18923));
#4748=EDGE_LOOP('',(#18924,#18925,#18926,#18927));
#4749=EDGE_LOOP('',(#18928,#18929,#18930,#18931));
#4750=EDGE_LOOP('',(#18932,#18933,#18934,#18935));
#4751=EDGE_LOOP('',(#18936,#18937,#18938,#18939));
#4752=EDGE_LOOP('',(#18940,#18941,#18942,#18943,#18944,#18945,#18946,#18947,
#18948,#18949,#18950,#18951,#18952,#18953,#18954,#18955,#18956));
#4753=EDGE_LOOP('',(#18957,#18958,#18959,#18960,#18961,#18962));
#4754=EDGE_LOOP('',(#18963,#18964,#18965,#18966,#18967));
#4755=EDGE_LOOP('',(#18968,#18969,#18970,#18971,#18972));
#4756=EDGE_LOOP('',(#18973,#18974,#18975,#18976));
#4757=EDGE_LOOP('',(#18977,#18978,#18979,#18980,#18981));
#4758=EDGE_LOOP('',(#18982,#18983,#18984,#18985));
#4759=EDGE_LOOP('',(#18986,#18987,#18988,#18989));
#4760=EDGE_LOOP('',(#18990,#18991,#18992,#18993));
#4761=EDGE_LOOP('',(#18994,#18995,#18996,#18997,#18998,#18999,#19000,#19001,
#19002,#19003,#19004,#19005));
#4762=EDGE_LOOP('',(#19006,#19007,#19008,#19009,#19010,#19011));
#4763=EDGE_LOOP('',(#19012,#19013,#19014,#19015,#19016));
#4764=EDGE_LOOP('',(#19017,#19018,#19019,#19020,#19021));
#4765=EDGE_LOOP('',(#19022,#19023,#19024,#19025));
#4766=EDGE_LOOP('',(#19026,#19027,#19028,#19029));
#4767=EDGE_LOOP('',(#19030,#19031,#19032,#19033,#19034));
#4768=EDGE_LOOP('',(#19035,#19036,#19037,#19038));
#4769=EDGE_LOOP('',(#19039,#19040,#19041,#19042));
#4770=EDGE_LOOP('',(#19043,#19044,#19045,#19046,#19047,#19048,#19049,#19050,
#19051,#19052,#19053,#19054));
#4771=EDGE_LOOP('',(#19055,#19056,#19057,#19058,#19059,#19060));
#4772=EDGE_LOOP('',(#19061,#19062,#19063,#19064,#19065));
#4773=EDGE_LOOP('',(#19066,#19067,#19068,#19069));
#4774=EDGE_LOOP('',(#19070,#19071,#19072,#19073));
#4775=EDGE_LOOP('',(#19074,#19075,#19076,#19077,#19078));
#4776=EDGE_LOOP('',(#19079,#19080,#19081,#19082));
#4777=EDGE_LOOP('',(#19083,#19084,#19085,#19086));
#4778=EDGE_LOOP('',(#19087,#19088,#19089,#19090));
#4779=EDGE_LOOP('',(#19091,#19092,#19093,#19094,#19095,#19096,#19097,#19098,
#19099,#19100,#19101,#19102));
#4780=EDGE_LOOP('',(#19103,#19104,#19105,#19106,#19107,#19108));
#4781=EDGE_LOOP('',(#19109,#19110,#19111,#19112,#19113));
#4782=EDGE_LOOP('',(#19114,#19115,#19116,#19117));
#4783=EDGE_LOOP('',(#19118,#19119,#19120,#19121));
#4784=EDGE_LOOP('',(#19122,#19123,#19124,#19125));
#4785=EDGE_LOOP('',(#19126,#19127,#19128,#19129));
#4786=EDGE_LOOP('',(#19130,#19131,#19132,#19133));
#4787=EDGE_LOOP('',(#19134));
#4788=EDGE_LOOP('',(#19135));
#4789=EDGE_LOOP('',(#19136,#19137,#19138,#19139));
#4790=EDGE_LOOP('',(#19140,#19141,#19142,#19143));
#4791=EDGE_LOOP('',(#19144));
#4792=EDGE_LOOP('',(#19145));
#4793=EDGE_LOOP('',(#19146,#19147,#19148,#19149));
#4794=EDGE_LOOP('',(#19150,#19151,#19152,#19153));
#4795=EDGE_LOOP('',(#19154,#19155,#19156,#19157));
#4796=EDGE_LOOP('',(#19158,#19159,#19160,#19161));
#4797=EDGE_LOOP('',(#19162,#19163,#19164,#19165));
#4798=EDGE_LOOP('',(#19166,#19167,#19168,#19169));
#4799=EDGE_LOOP('',(#19170,#19171,#19172,#19173));
#4800=EDGE_LOOP('',(#19174,#19175,#19176,#19177));
#4801=EDGE_LOOP('',(#19178,#19179,#19180,#19181));
#4802=EDGE_LOOP('',(#19182,#19183,#19184,#19185));
#4803=EDGE_LOOP('',(#19186,#19187,#19188,#19189));
#4804=EDGE_LOOP('',(#19190,#19191,#19192,#19193));
#4805=EDGE_LOOP('',(#19194,#19195,#19196,#19197));
#4806=EDGE_LOOP('',(#19198,#19199,#19200,#19201));
#4807=EDGE_LOOP('',(#19202,#19203,#19204,#19205));
#4808=EDGE_LOOP('',(#19206,#19207,#19208,#19209));
#4809=EDGE_LOOP('',(#19210,#19211,#19212,#19213));
#4810=EDGE_LOOP('',(#19214,#19215,#19216,#19217));
#4811=EDGE_LOOP('',(#19218,#19219,#19220,#19221));
#4812=EDGE_LOOP('',(#19222,#19223,#19224,#19225));
#4813=EDGE_LOOP('',(#19226,#19227,#19228,#19229));
#4814=EDGE_LOOP('',(#19230,#19231,#19232,#19233,#19234,#19235,#19236,#19237,
#19238,#19239));
#4815=EDGE_LOOP('',(#19240,#19241,#19242,#19243,#19244,#19245,#19246,#19247));
#4816=EDGE_LOOP('',(#19248,#19249,#19250,#19251));
#4817=EDGE_LOOP('',(#19252,#19253,#19254,#19255));
#4818=EDGE_LOOP('',(#19256,#19257,#19258,#19259));
#4819=EDGE_LOOP('',(#19260,#19261,#19262,#19263));
#4820=EDGE_LOOP('',(#19264,#19265,#19266,#19267));
#4821=EDGE_LOOP('',(#19268,#19269,#19270,#19271));
#4822=EDGE_LOOP('',(#19272,#19273,#19274,#19275));
#4823=EDGE_LOOP('',(#19276,#19277,#19278,#19279));
#4824=EDGE_LOOP('',(#19280,#19281,#19282,#19283,#19284,#19285,#19286,#19287));
#4825=EDGE_LOOP('',(#19288,#19289,#19290,#19291));
#4826=EDGE_LOOP('',(#19292,#19293,#19294,#19295));
#4827=EDGE_LOOP('',(#19296,#19297,#19298,#19299));
#4828=EDGE_LOOP('',(#19300,#19301,#19302,#19303));
#4829=EDGE_LOOP('',(#19304,#19305,#19306,#19307));
#4830=EDGE_LOOP('',(#19308,#19309,#19310,#19311));
#4831=EDGE_LOOP('',(#19312,#19313,#19314,#19315));
#4832=EDGE_LOOP('',(#19316,#19317,#19318,#19319));
#4833=EDGE_LOOP('',(#19320,#19321,#19322,#19323));
#4834=EDGE_LOOP('',(#19324,#19325,#19326,#19327));
#4835=EDGE_LOOP('',(#19328,#19329,#19330,#19331));
#4836=EDGE_LOOP('',(#19332,#19333,#19334,#19335));
#4837=EDGE_LOOP('',(#19336,#19337,#19338,#19339));
#4838=EDGE_LOOP('',(#19340,#19341,#19342,#19343));
#4839=EDGE_LOOP('',(#19344,#19345,#19346,#19347));
#4840=EDGE_LOOP('',(#19348,#19349,#19350,#19351));
#4841=EDGE_LOOP('',(#19352,#19353,#19354,#19355));
#4842=EDGE_LOOP('',(#19356,#19357,#19358,#19359));
#4843=EDGE_LOOP('',(#19360,#19361,#19362,#19363));
#4844=EDGE_LOOP('',(#19364,#19365,#19366,#19367));
#4845=EDGE_LOOP('',(#19368,#19369,#19370,#19371));
#4846=EDGE_LOOP('',(#19372,#19373,#19374,#19375));
#4847=EDGE_LOOP('',(#19376,#19377,#19378,#19379,#19380,#19381,#19382,#19383,
#19384,#19385,#19386,#19387,#19388));
#4848=EDGE_LOOP('',(#19389,#19390,#19391,#19392,#19393,#19394,#19395,#19396,
#19397));
#4849=EDGE_LOOP('',(#19398,#19399,#19400,#19401));
#4850=EDGE_LOOP('',(#19402,#19403,#19404,#19405));
#4851=EDGE_LOOP('',(#19406,#19407,#19408,#19409));
#4852=EDGE_LOOP('',(#19410,#19411,#19412,#19413));
#4853=EDGE_LOOP('',(#19414,#19415,#19416,#19417));
#4854=EDGE_LOOP('',(#19418,#19419,#19420,#19421));
#4855=EDGE_LOOP('',(#19422,#19423,#19424,#19425));
#4856=EDGE_LOOP('',(#19426,#19427,#19428,#19429));
#4857=EDGE_LOOP('',(#19430,#19431,#19432,#19433));
#4858=EDGE_LOOP('',(#19434,#19435,#19436,#19437));
#4859=EDGE_LOOP('',(#19438,#19439,#19440,#19441));
#4860=EDGE_LOOP('',(#19442,#19443,#19444,#19445));
#4861=EDGE_LOOP('',(#19446,#19447,#19448,#19449));
#4862=EDGE_LOOP('',(#19450,#19451,#19452,#19453));
#4863=EDGE_LOOP('',(#19454,#19455,#19456,#19457));
#4864=EDGE_LOOP('',(#19458,#19459,#19460,#19461));
#4865=EDGE_LOOP('',(#19462,#19463,#19464,#19465));
#4866=EDGE_LOOP('',(#19466,#19467,#19468,#19469));
#4867=EDGE_LOOP('',(#19470,#19471,#19472,#19473));
#4868=EDGE_LOOP('',(#19474,#19475,#19476,#19477));
#4869=EDGE_LOOP('',(#19478,#19479,#19480,#19481));
#4870=EDGE_LOOP('',(#19482,#19483,#19484,#19485));
#4871=EDGE_LOOP('',(#19486,#19487,#19488,#19489,#19490,#19491,#19492,#19493,
#19494,#19495,#19496,#19497,#19498,#19499,#19500,#19501,#19502,#19503,#19504,
#19505,#19506,#19507));
#4872=EDGE_LOOP('',(#19508,#19509,#19510,#19511));
#4873=EDGE_LOOP('',(#19512,#19513,#19514,#19515));
#4874=EDGE_LOOP('',(#19516,#19517,#19518,#19519));
#4875=EDGE_LOOP('',(#19520,#19521,#19522,#19523));
#4876=EDGE_LOOP('',(#19524,#19525,#19526,#19527));
#4877=EDGE_LOOP('',(#19528,#19529,#19530,#19531));
#4878=EDGE_LOOP('',(#19532,#19533,#19534,#19535));
#4879=EDGE_LOOP('',(#19536,#19537,#19538,#19539));
#4880=EDGE_LOOP('',(#19540,#19541,#19542,#19543));
#4881=EDGE_LOOP('',(#19544,#19545,#19546,#19547));
#4882=EDGE_LOOP('',(#19548,#19549,#19550,#19551,#19552,#19553,#19554,#19555,
#19556,#19557));
#4883=EDGE_LOOP('',(#19558,#19559,#19560,#19561,#19562,#19563,#19564,#19565,
#19566));
#4884=EDGE_LOOP('',(#19567,#19568,#19569,#19570,#19571,#19572,#19573,#19574));
#4885=EDGE_LOOP('',(#19575,#19576,#19577,#19578));
#4886=EDGE_LOOP('',(#19579,#19580,#19581,#19582,#19583,#19584,#19585,#19586));
#4887=EDGE_LOOP('',(#19587,#19588,#19589,#19590));
#4888=EDGE_LOOP('',(#19591,#19592,#19593,#19594));
#4889=EDGE_LOOP('',(#19595,#19596,#19597,#19598));
#4890=EDGE_LOOP('',(#19599,#19600,#19601,#19602));
#6302=LINE('',#37682,#8790);
#6303=LINE('',#37684,#8791);
#6304=LINE('',#37686,#8792);
#6305=LINE('',#37688,#8793);
#6306=LINE('',#37689,#8794);
#6307=LINE('',#37692,#8795);
#6308=LINE('',#37694,#8796);
#6309=LINE('',#37696,#8797);
#6310=LINE('',#37698,#8798);
#6311=LINE('',#37699,#8799);
#6312=LINE('',#37702,#8800);
#6313=LINE('',#37703,#8801);
#6314=LINE('',#37706,#8802);
#6315=LINE('',#37707,#8803);
#6316=LINE('',#37710,#8804);
#6317=LINE('',#37711,#8805);
#6318=LINE('',#37714,#8806);
#6319=LINE('',#37716,#8807);
#6320=LINE('',#37718,#8808);
#6321=LINE('',#37719,#8809);
#6322=LINE('',#37722,#8810);
#6323=LINE('',#37724,#8811);
#6324=LINE('',#37726,#8812);
#6325=LINE('',#37728,#8813);
#6326=LINE('',#37730,#8814);
#6327=LINE('',#37731,#8815);
#6328=LINE('',#37735,#8816);
#6329=LINE('',#37737,#8817);
#6330=LINE('',#37739,#8818);
#6331=LINE('',#37741,#8819);
#6332=LINE('',#37742,#8820);
#6333=LINE('',#37745,#8821);
#6334=LINE('',#37747,#8822);
#6335=LINE('',#37748,#8823);
#6336=LINE('',#37751,#8824);
#6337=LINE('',#37752,#8825);
#6338=LINE('',#37753,#8826);
#6339=LINE('',#37755,#8827);
#6340=LINE('',#37756,#8828);
#6341=LINE('',#37758,#8829);
#6342=LINE('',#37759,#8830);
#6343=LINE('',#37762,#8831);
#6344=LINE('',#37763,#8832);
#6345=LINE('',#37769,#8833);
#6346=LINE('',#37774,#8834);
#6347=LINE('',#37776,#8835);
#6348=LINE('',#37778,#8836);
#6349=LINE('',#37779,#8837);
#6350=LINE('',#37788,#8838);
#6351=LINE('',#37792,#8839);
#6352=LINE('',#37796,#8840);
#6353=LINE('',#37800,#8841);
#6354=LINE('',#37804,#8842);
#6355=LINE('',#37808,#8843);
#6356=LINE('',#37812,#8844);
#6357=LINE('',#37817,#8845);
#6358=LINE('',#37821,#8846);
#6359=LINE('',#37823,#8847);
#6360=LINE('',#37825,#8848);
#6361=LINE('',#37826,#8849);
#6362=LINE('',#37834,#8850);
#6363=LINE('',#37836,#8851);
#6364=LINE('',#37838,#8852);
#6365=LINE('',#37843,#8853);
#6366=LINE('',#37848,#8854);
#6367=LINE('',#37850,#8855);
#6368=LINE('',#37852,#8856);
#6369=LINE('',#37853,#8857);
#6370=LINE('',#37863,#8858);
#6371=LINE('',#37866,#8859);
#6372=LINE('',#37871,#8860);
#6373=LINE('',#37874,#8861);
#6374=LINE('',#37879,#8862);
#6375=LINE('',#37882,#8863);
#6376=LINE('',#37887,#8864);
#6377=LINE('',#37891,#8865);
#6378=LINE('',#37897,#8866);
#6379=LINE('',#37937,#8867);
#6380=LINE('',#37949,#8868);
#6381=LINE('',#38009,#8869);
#6382=LINE('',#38013,#8870);
#6383=LINE('',#38017,#8871);
#6384=LINE('',#38039,#8872);
#6385=LINE('',#38042,#8873);
#6386=LINE('',#38097,#8874);
#6387=LINE('',#38101,#8875);
#6388=LINE('',#38103,#8876);
#6389=LINE('',#38105,#8877);
#6390=LINE('',#38106,#8878);
#6391=LINE('',#38114,#8879);
#6392=LINE('',#38116,#8880);
#6393=LINE('',#38118,#8881);
#6394=LINE('',#38122,#8882);
#6395=LINE('',#38126,#8883);
#6396=LINE('',#38130,#8884);
#6397=LINE('',#38131,#8885);
#6398=LINE('',#38132,#8886);
#6399=LINE('',#38135,#8887);
#6400=LINE('',#38139,#8888);
#6401=LINE('',#38141,#8889);
#6402=LINE('',#38142,#8890);
#6403=LINE('',#38145,#8891);
#6404=LINE('',#38150,#8892);
#6405=LINE('',#38151,#8893);
#6406=LINE('',#38155,#8894);
#6407=LINE('',#38159,#8895);
#6408=LINE('',#38160,#8896);
#6409=LINE('',#38162,#8897);
#6410=LINE('',#38164,#8898);
#6411=LINE('',#38166,#8899);
#6412=LINE('',#38169,#8900);
#6413=LINE('',#38172,#8901);
#6414=LINE('',#38195,#8902);
#6415=LINE('',#38219,#8903);
#6416=LINE('',#38222,#8904);
#6417=LINE('',#38226,#8905);
#6418=LINE('',#38230,#8906);
#6419=LINE('',#38234,#8907);
#6420=LINE('',#38238,#8908);
#6421=LINE('',#38242,#8909);
#6422=LINE('',#38244,#8910);
#6423=LINE('',#38248,#8911);
#6424=LINE('',#38249,#8912);
#6425=LINE('',#38250,#8913);
#6426=LINE('',#38253,#8914);
#6427=LINE('',#38257,#8915);
#6428=LINE('',#38258,#8916);
#6429=LINE('',#38262,#8917);
#6430=LINE('',#38267,#8918);
#6431=LINE('',#38268,#8919);
#6432=LINE('',#38269,#8920);
#6433=LINE('',#38272,#8921);
#6434=LINE('',#38275,#8922);
#6435=LINE('',#38276,#8923);
#6436=LINE('',#38278,#8924);
#6437=LINE('',#38325,#8925);
#6438=LINE('',#38327,#8926);
#6439=LINE('',#38329,#8927);
#6440=LINE('',#38331,#8928);
#6441=LINE('',#38333,#8929);
#6442=LINE('',#38335,#8930);
#6443=LINE('',#38337,#8931);
#6444=LINE('',#38338,#8932);
#6445=LINE('',#38393,#8933);
#6446=LINE('',#38395,#8934);
#6447=LINE('',#38397,#8935);
#6448=LINE('',#38431,#8936);
#6449=LINE('',#38473,#8937);
#6450=LINE('',#38475,#8938);
#6451=LINE('',#38477,#8939);
#6452=LINE('',#38479,#8940);
#6453=LINE('',#38481,#8941);
#6454=LINE('',#38483,#8942);
#6455=LINE('',#38485,#8943);
#6456=LINE('',#38487,#8944);
#6457=LINE('',#38489,#8945);
#6458=LINE('',#38490,#8946);
#6459=LINE('',#38494,#8947);
#6460=LINE('',#38498,#8948);
#6461=LINE('',#38502,#8949);
#6462=LINE('',#38506,#8950);
#6463=LINE('',#38510,#8951);
#6464=LINE('',#38515,#8952);
#6465=LINE('',#38561,#8953);
#6466=LINE('',#38563,#8954);
#6467=LINE('',#38617,#8955);
#6468=LINE('',#38665,#8956);
#6469=LINE('',#38670,#8957);
#6470=LINE('',#38712,#8958);
#6471=LINE('',#38714,#8959);
#6472=LINE('',#38767,#8960);
#6473=LINE('',#38821,#8961);
#6474=LINE('',#38823,#8962);
#6475=LINE('',#38824,#8963);
#6476=LINE('',#38827,#8964);
#6477=LINE('',#38831,#8965);
#6478=LINE('',#38832,#8966);
#6479=LINE('',#38834,#8967);
#6480=LINE('',#38837,#8968);
#6481=LINE('',#38840,#8969);
#6482=LINE('',#38844,#8970);
#6483=LINE('',#38845,#8971);
#6484=LINE('',#38850,#8972);
#6485=LINE('',#38854,#8973);
#6486=LINE('',#38855,#8974);
#6487=LINE('',#38858,#8975);
#6488=LINE('',#38908,#8976);
#6489=LINE('',#38956,#8977);
#6490=LINE('',#38960,#8978);
#6491=LINE('',#38964,#8979);
#6492=LINE('',#38968,#8980);
#6493=LINE('',#38969,#8981);
#6494=LINE('',#39052,#8982);
#6495=LINE('',#39053,#8983);
#6496=LINE('',#39055,#8984);
#6497=LINE('',#39056,#8985);
#6498=LINE('',#39090,#8986);
#6499=LINE('',#39091,#8987);
#6500=LINE('',#39095,#8988);
#6501=LINE('',#39098,#8989);
#6502=LINE('',#39099,#8990);
#6503=LINE('',#39102,#8991);
#6504=LINE('',#39104,#8992);
#6505=LINE('',#39106,#8993);
#6506=LINE('',#39108,#8994);
#6507=LINE('',#39111,#8995);
#6508=LINE('',#39113,#8996);
#6509=LINE('',#39298,#8997);
#6510=LINE('',#39299,#8998);
#6511=LINE('',#39301,#8999);
#6512=LINE('',#39302,#9000);
#6513=LINE('',#39431,#9001);
#6514=LINE('',#39432,#9002);
#6515=LINE('',#39434,#9003);
#6516=LINE('',#39435,#9004);
#6517=LINE('',#39470,#9005);
#6518=LINE('',#39475,#9006);
#6519=LINE('',#39517,#9007);
#6520=LINE('',#39519,#9008);
#6521=LINE('',#39572,#9009);
#6522=LINE('',#39690,#9010);
#6523=LINE('',#39691,#9011);
#6524=LINE('',#39693,#9012);
#6525=LINE('',#39694,#9013);
#6526=LINE('',#39730,#9014);
#6527=LINE('',#39734,#9015);
#6528=LINE('',#39739,#9016);
#6529=LINE('',#39740,#9017);
#6530=LINE('',#39741,#9018);
#6531=LINE('',#39745,#9019);
#6532=LINE('',#39751,#9020);
#6533=LINE('',#39752,#9021);
#6534=LINE('',#39753,#9022);
#6535=LINE('',#39756,#9023);
#6536=LINE('',#39761,#9024);
#6537=LINE('',#39762,#9025);
#6538=LINE('',#39766,#9026);
#6539=LINE('',#39770,#9027);
#6540=LINE('',#39771,#9028);
#6541=LINE('',#39774,#9029);
#6542=LINE('',#39775,#9030);
#6543=LINE('',#39777,#9031);
#6544=LINE('',#39781,#9032);
#6545=LINE('',#39782,#9033);
#6546=LINE('',#39785,#9034);
#6547=LINE('',#39808,#9035);
#6548=LINE('',#39831,#9036);
#6549=LINE('',#39834,#9037);
#6550=LINE('',#39835,#9038);
#6551=LINE('',#39839,#9039);
#6552=LINE('',#39843,#9040);
#6553=LINE('',#39847,#9041);
#6554=LINE('',#39851,#9042);
#6555=LINE('',#39855,#9043);
#6556=LINE('',#39857,#9044);
#6557=LINE('',#39861,#9045);
#6558=LINE('',#39862,#9046);
#6559=LINE('',#39863,#9047);
#6560=LINE('',#39866,#9048);
#6561=LINE('',#39870,#9049);
#6562=LINE('',#39871,#9050);
#6563=LINE('',#39875,#9051);
#6564=LINE('',#39880,#9052);
#6565=LINE('',#39882,#9053);
#6566=LINE('',#39883,#9054);
#6567=LINE('',#39887,#9055);
#6568=LINE('',#39891,#9056);
#6569=LINE('',#39892,#9057);
#6570=LINE('',#39894,#9058);
#6571=LINE('',#39895,#9059);
#6572=LINE('',#39898,#9060);
#6573=LINE('',#39921,#9061);
#6574=LINE('',#39944,#9062);
#6575=LINE('',#39953,#9063);
#6576=LINE('',#39957,#9064);
#6577=LINE('',#39961,#9065);
#6578=LINE('',#39965,#9066);
#6579=LINE('',#40008,#9067);
#6580=LINE('',#40010,#9068);
#6581=LINE('',#40023,#9069);
#6582=LINE('',#40028,#9070);
#6583=LINE('',#40071,#9071);
#6584=LINE('',#40122,#9072);
#6585=LINE('',#40124,#9073);
#6586=LINE('',#40125,#9074);
#6587=LINE('',#40129,#9075);
#6588=LINE('',#40132,#9076);
#6589=LINE('',#40133,#9077);
#6590=LINE('',#40136,#9078);
#6591=LINE('',#40138,#9079);
#6592=LINE('',#40142,#9080);
#6593=LINE('',#40145,#9081);
#6594=LINE('',#40146,#9082);
#6595=LINE('',#40151,#9083);
#6596=LINE('',#40155,#9084);
#6597=LINE('',#40156,#9085);
#6598=LINE('',#40159,#9086);
#6599=LINE('',#40204,#9087);
#6600=LINE('',#40254,#9088);
#6601=LINE('',#40258,#9089);
#6602=LINE('',#40262,#9090);
#6603=LINE('',#40266,#9091);
#6604=LINE('',#40267,#9092);
#6605=LINE('',#40271,#9093);
#6606=LINE('',#40272,#9094);
#6607=LINE('',#40274,#9095);
#6608=LINE('',#40276,#9096);
#6609=LINE('',#40278,#9097);
#6610=LINE('',#40280,#9098);
#6611=LINE('',#40283,#9099);
#6612=LINE('',#40287,#9100);
#6613=LINE('',#40288,#9101);
#6614=LINE('',#40292,#9102);
#6615=LINE('',#40294,#9103);
#6616=LINE('',#40466,#9104);
#6617=LINE('',#40467,#9105);
#6618=LINE('',#40469,#9106);
#6619=LINE('',#40470,#9107);
#6620=LINE('',#40505,#9108);
#6621=LINE('',#40510,#9109);
#6622=LINE('',#40552,#9110);
#6623=LINE('',#40554,#9111);
#6624=LINE('',#40607,#9112);
#6625=LINE('',#40733,#9113);
#6626=LINE('',#40734,#9114);
#6627=LINE('',#40736,#9115);
#6628=LINE('',#40737,#9116);
#6629=LINE('',#40815,#9117);
#6630=LINE('',#40817,#9118);
#6631=LINE('',#40831,#9119);
#6632=LINE('',#40836,#9120);
#6633=LINE('',#40879,#9121);
#6634=LINE('',#41009,#9122);
#6635=LINE('',#41010,#9123);
#6636=LINE('',#41012,#9124);
#6637=LINE('',#41013,#9125);
#6638=LINE('',#41048,#9126);
#6639=LINE('',#41053,#9127);
#6640=LINE('',#41095,#9128);
#6641=LINE('',#41097,#9129);
#6642=LINE('',#41150,#9130);
#6643=LINE('',#41276,#9131);
#6644=LINE('',#41277,#9132);
#6645=LINE('',#41279,#9133);
#6646=LINE('',#41280,#9134);
#6647=LINE('',#41317,#9135);
#6648=LINE('',#41321,#9136);
#6649=LINE('',#41329,#9137);
#6650=LINE('',#41331,#9138);
#6651=LINE('',#41336,#9139);
#6652=LINE('',#41340,#9140);
#6653=LINE('',#41343,#9141);
#6654=LINE('',#41356,#9142);
#6655=LINE('',#41361,#9143);
#6656=LINE('',#41373,#9144);
#6657=LINE('',#41388,#9145);
#6658=LINE('',#41403,#9146);
#6659=LINE('',#41418,#9147);
#6660=LINE('',#41433,#9148);
#6661=LINE('',#41448,#9149);
#6662=LINE('',#41471,#9150);
#6663=LINE('',#41476,#9151);
#6664=LINE('',#41484,#9152);
#6665=LINE('',#41495,#9153);
#6666=LINE('',#41506,#9154);
#6667=LINE('',#41517,#9155);
#6668=LINE('',#41528,#9156);
#6669=LINE('',#41539,#9157);
#6670=LINE('',#41550,#9158);
#6671=LINE('',#41561,#9159);
#6672=LINE('',#41577,#9160);
#6673=LINE('',#41579,#9161);
#6674=LINE('',#41580,#9162);
#6675=LINE('',#41583,#9163);
#6676=LINE('',#41584,#9164);
#6677=LINE('',#41587,#9165);
#6678=LINE('',#41588,#9166);
#6679=LINE('',#41591,#9167);
#6680=LINE('',#41592,#9168);
#6681=LINE('',#41595,#9169);
#6682=LINE('',#41596,#9170);
#6683=LINE('',#41599,#9171);
#6684=LINE('',#41600,#9172);
#6685=LINE('',#41603,#9173);
#6686=LINE('',#41604,#9174);
#6687=LINE('',#41606,#9175);
#6688=LINE('',#41620,#9176);
#6689=LINE('',#41625,#9177);
#6690=LINE('',#41637,#9178);
#6691=LINE('',#41652,#9179);
#6692=LINE('',#41667,#9180);
#6693=LINE('',#41682,#9181);
#6694=LINE('',#41697,#9182);
#6695=LINE('',#41712,#9183);
#6696=LINE('',#41727,#9184);
#6697=LINE('',#41750,#9185);
#6698=LINE('',#41755,#9186);
#6699=LINE('',#41763,#9187);
#6700=LINE('',#41774,#9188);
#6701=LINE('',#41785,#9189);
#6702=LINE('',#41796,#9190);
#6703=LINE('',#41807,#9191);
#6704=LINE('',#41818,#9192);
#6705=LINE('',#41829,#9193);
#6706=LINE('',#41840,#9194);
#6707=LINE('',#41851,#9195);
#6708=LINE('',#41862,#9196);
#6709=LINE('',#41873,#9197);
#6710=LINE('',#41889,#9198);
#6711=LINE('',#41891,#9199);
#6712=LINE('',#41892,#9200);
#6713=LINE('',#41900,#9201);
#6714=LINE('',#41911,#9202);
#6715=LINE('',#41922,#9203);
#6716=LINE('',#41933,#9204);
#6717=LINE('',#41944,#9205);
#6718=LINE('',#41955,#9206);
#6719=LINE('',#41966,#9207);
#6720=LINE('',#41977,#9208);
#6721=LINE('',#41988,#9209);
#6722=LINE('',#41999,#9210);
#6723=LINE('',#42005,#9211);
#6724=LINE('',#42006,#9212);
#6725=LINE('',#42014,#9213);
#6726=LINE('',#42025,#9214);
#6727=LINE('',#42036,#9215);
#6728=LINE('',#42047,#9216);
#6729=LINE('',#42058,#9217);
#6730=LINE('',#42069,#9218);
#6731=LINE('',#42080,#9219);
#6732=LINE('',#42091,#9220);
#6733=LINE('',#42097,#9221);
#6734=LINE('',#42098,#9222);
#6735=LINE('',#42100,#9223);
#6736=LINE('',#42104,#9224);
#6737=LINE('',#42106,#9225);
#6738=LINE('',#42107,#9226);
#6739=LINE('',#42110,#9227);
#6740=LINE('',#42111,#9228);
#6741=LINE('',#42114,#9229);
#6742=LINE('',#42115,#9230);
#6743=LINE('',#42118,#9231);
#6744=LINE('',#42119,#9232);
#6745=LINE('',#42122,#9233);
#6746=LINE('',#42123,#9234);
#6747=LINE('',#42126,#9235);
#6748=LINE('',#42127,#9236);
#6749=LINE('',#42130,#9237);
#6750=LINE('',#42131,#9238);
#6751=LINE('',#42134,#9239);
#6752=LINE('',#42135,#9240);
#6753=LINE('',#42138,#9241);
#6754=LINE('',#42139,#9242);
#6755=LINE('',#42141,#9243);
#6756=LINE('',#42146,#9244);
#6757=LINE('',#42148,#9245);
#8790=VECTOR('',#30861,1.);
#8791=VECTOR('',#30862,1.);
#8792=VECTOR('',#30863,1.);
#8793=VECTOR('',#30864,1.);
#8794=VECTOR('',#30865,1.);
#8795=VECTOR('',#30868,1.);
#8796=VECTOR('',#30869,1.);
#8797=VECTOR('',#30870,1.);
#8798=VECTOR('',#30871,1.);
#8799=VECTOR('',#30872,1.);
#8800=VECTOR('',#30875,1.);
#8801=VECTOR('',#30876,1.);
#8802=VECTOR('',#30879,1.);
#8803=VECTOR('',#30880,1.);
#8804=VECTOR('',#30883,1.);
#8805=VECTOR('',#30884,1.);
#8806=VECTOR('',#30887,1.);
#8807=VECTOR('',#30888,1.);
#8808=VECTOR('',#30889,1.);
#8809=VECTOR('',#30890,1.);
#8810=VECTOR('',#30893,1.);
#8811=VECTOR('',#30894,1.);
#8812=VECTOR('',#30895,1.);
#8813=VECTOR('',#30896,1.);
#8814=VECTOR('',#30897,1.);
#8815=VECTOR('',#30898,1.);
#8816=VECTOR('',#30901,1.);
#8817=VECTOR('',#30902,1.);
#8818=VECTOR('',#30903,1.);
#8819=VECTOR('',#30904,1.);
#8820=VECTOR('',#30905,1.);
#8821=VECTOR('',#30908,1.);
#8822=VECTOR('',#30909,1.);
#8823=VECTOR('',#30910,1.);
#8824=VECTOR('',#30913,1.);
#8825=VECTOR('',#30914,1.);
#8826=VECTOR('',#30915,1.);
#8827=VECTOR('',#30918,1.);
#8828=VECTOR('',#30919,1.);
#8829=VECTOR('',#30922,1.);
#8830=VECTOR('',#30923,1.);
#8831=VECTOR('',#30926,1.);
#8832=VECTOR('',#30927,1.);
#8833=VECTOR('',#30934,0.925000000000001);
#8834=VECTOR('',#30939,1.);
#8835=VECTOR('',#30940,1.);
#8836=VECTOR('',#30941,1.);
#8837=VECTOR('',#30942,1.);
#8838=VECTOR('',#30951,0.875);
#8839=VECTOR('',#30956,0.925000000000001);
#8840=VECTOR('',#30961,0.875);
#8841=VECTOR('',#30966,0.925000000000001);
#8842=VECTOR('',#30971,0.875);
#8843=VECTOR('',#30976,0.925000000000001);
#8844=VECTOR('',#30981,0.875);
#8845=VECTOR('',#30988,0.925000000000001);
#8846=VECTOR('',#30991,1.);
#8847=VECTOR('',#30992,1.);
#8848=VECTOR('',#30993,1.);
#8849=VECTOR('',#30994,1.);
#8850=VECTOR('',#31003,0.925000000000001);
#8851=VECTOR('',#31006,0.925000000000001);
#8852=VECTOR('',#31009,0.925000000000001);
#8853=VECTOR('',#31014,0.925000000000001);
#8854=VECTOR('',#31019,1.);
#8855=VECTOR('',#31020,1.);
#8856=VECTOR('',#31021,1.);
#8857=VECTOR('',#31022,1.);
#8858=VECTOR('',#31033,0.875);
#8859=VECTOR('',#31036,0.925000000000001);
#8860=VECTOR('',#31043,0.875);
#8861=VECTOR('',#31046,0.925000000000001);
#8862=VECTOR('',#31053,0.875);
#8863=VECTOR('',#31056,0.925000000000001);
#8864=VECTOR('',#31063,0.875);
#8865=VECTOR('',#31066,1.);
#8866=VECTOR('',#31071,1.);
#8867=VECTOR('',#31074,1.);
#8868=VECTOR('',#31075,1.);
#8869=VECTOR('',#31078,1.);
#8870=VECTOR('',#31081,1.);
#8871=VECTOR('',#31084,1.);
#8872=VECTOR('',#31085,1.);
#8873=VECTOR('',#31088,1.8);
#8874=VECTOR('',#31097,0.925000000000001);
#8875=VECTOR('',#31100,1.);
#8876=VECTOR('',#31101,1.);
#8877=VECTOR('',#31102,1.);
#8878=VECTOR('',#31103,1.);
#8879=VECTOR('',#31112,0.925000000000001);
#8880=VECTOR('',#31115,0.925000000000001);
#8881=VECTOR('',#31118,0.925000000000001);
#8882=VECTOR('',#31121,1.);
#8883=VECTOR('',#31124,1.);
#8884=VECTOR('',#31129,1.);
#8885=VECTOR('',#31130,1.);
#8886=VECTOR('',#31131,1.);
#8887=VECTOR('',#31134,1.);
#8888=VECTOR('',#31139,1.);
#8889=VECTOR('',#31140,1.);
#8890=VECTOR('',#31141,1.);
#8891=VECTOR('',#31144,1.);
#8892=VECTOR('',#31151,1.);
#8893=VECTOR('',#31152,1.);
#8894=VECTOR('',#31155,1.);
#8895=VECTOR('',#31162,1.);
#8896=VECTOR('',#31163,1.);
#8897=VECTOR('',#31166,1.);
#8898=VECTOR('',#31167,1.);
#8899=VECTOR('',#31168,1.);
#8900=VECTOR('',#31173,1.);
#8901=VECTOR('',#31176,1.);
#8902=VECTOR('',#31177,1.);
#8903=VECTOR('',#31178,1.);
#8904=VECTOR('',#31181,1.);
#8905=VECTOR('',#31184,1.);
#8906=VECTOR('',#31187,1.);
#8907=VECTOR('',#31190,1.);
#8908=VECTOR('',#31193,1.);
#8909=VECTOR('',#31198,1.);
#8910=VECTOR('',#31199,1.);
#8911=VECTOR('',#31204,1.);
#8912=VECTOR('',#31205,1.);
#8913=VECTOR('',#31206,1.);
#8914=VECTOR('',#31209,1.);
#8915=VECTOR('',#31214,1.);
#8916=VECTOR('',#31215,1.);
#8917=VECTOR('',#31218,1.);
#8918=VECTOR('',#31225,1.);
#8919=VECTOR('',#31226,1.);
#8920=VECTOR('',#31227,1.);
#8921=VECTOR('',#31230,1.);
#8922=VECTOR('',#31235,1.);
#8923=VECTOR('',#31236,1.);
#8924=VECTOR('',#31239,1.);
#8925=VECTOR('',#31248,1.);
#8926=VECTOR('',#31249,1.);
#8927=VECTOR('',#31250,1.);
#8928=VECTOR('',#31251,1.);
#8929=VECTOR('',#31252,1.);
#8930=VECTOR('',#31253,1.);
#8931=VECTOR('',#31254,1.);
#8932=VECTOR('',#31255,1.);
#8933=VECTOR('',#31256,1.);
#8934=VECTOR('',#31257,1.);
#8935=VECTOR('',#31258,1.);
#8936=VECTOR('',#31259,1.);
#8937=VECTOR('',#31260,1.);
#8938=VECTOR('',#31261,1.);
#8939=VECTOR('',#31262,1.);
#8940=VECTOR('',#31263,1.);
#8941=VECTOR('',#31264,1.);
#8942=VECTOR('',#31265,1.);
#8943=VECTOR('',#31266,1.);
#8944=VECTOR('',#31267,1.);
#8945=VECTOR('',#31268,1.);
#8946=VECTOR('',#31269,1.);
#8947=VECTOR('',#31272,1.);
#8948=VECTOR('',#31275,1.);
#8949=VECTOR('',#31278,1.);
#8950=VECTOR('',#31281,1.);
#8951=VECTOR('',#31286,1.);
#8952=VECTOR('',#31291,1.);
#8953=VECTOR('',#31292,1.);
#8954=VECTOR('',#31293,1.);
#8955=VECTOR('',#31296,1.8);
#8956=VECTOR('',#31303,1.);
#8957=VECTOR('',#31308,1.);
#8958=VECTOR('',#31309,1.);
#8959=VECTOR('',#31310,1.);
#8960=VECTOR('',#31313,1.8);
#8961=VECTOR('',#31320,1.);
#8962=VECTOR('',#31321,1.);
#8963=VECTOR('',#31322,1.);
#8964=VECTOR('',#31325,1.);
#8965=VECTOR('',#31330,1.);
#8966=VECTOR('',#31331,1.);
#8967=VECTOR('',#31334,1.);
#8968=VECTOR('',#31339,1.);
#8969=VECTOR('',#31342,1.);
#8970=VECTOR('',#31347,1.);
#8971=VECTOR('',#31348,1.);
#8972=VECTOR('',#31355,1.);
#8973=VECTOR('',#31360,1.);
#8974=VECTOR('',#31361,1.);
#8975=VECTOR('',#31364,1.);
#8976=VECTOR('',#31365,1.);
#8977=VECTOR('',#31366,1.);
#8978=VECTOR('',#31371,1.);
#8979=VECTOR('',#31374,1.);
#8980=VECTOR('',#31377,1.);
#8981=VECTOR('',#31378,1.);
#8982=VECTOR('',#31383,1.);
#8983=VECTOR('',#31384,1.);
#8984=VECTOR('',#31387,1.);
#8985=VECTOR('',#31388,1.);
#8986=VECTOR('',#31391,1.);
#8987=VECTOR('',#31392,1.);
#8988=VECTOR('',#31397,1.);
#8989=VECTOR('',#31400,1.);
#8990=VECTOR('',#31401,1.);
#8991=VECTOR('',#31406,1.);
#8992=VECTOR('',#31409,1.);
#8993=VECTOR('',#31412,1.);
#8994=VECTOR('',#31415,1.);
#8995=VECTOR('',#31420,1.);
#8996=VECTOR('',#31423,1.);
#8997=VECTOR('',#31426,1.);
#8998=VECTOR('',#31427,1.);
#8999=VECTOR('',#31430,1.);
#9000=VECTOR('',#31431,1.);
#9001=VECTOR('',#31432,1.);
#9002=VECTOR('',#31433,1.);
#9003=VECTOR('',#31436,1.);
#9004=VECTOR('',#31437,1.);
#9005=VECTOR('',#31440,1.);
#9006=VECTOR('',#31445,1.);
#9007=VECTOR('',#31446,1.);
#9008=VECTOR('',#31447,1.);
#9009=VECTOR('',#31450,1.8);
#9010=VECTOR('',#31455,1.);
#9011=VECTOR('',#31456,1.);
#9012=VECTOR('',#31459,1.);
#9013=VECTOR('',#31460,1.);
#9014=VECTOR('',#31463,1.);
#9015=VECTOR('',#31466,1.);
#9016=VECTOR('',#31471,1.);
#9017=VECTOR('',#31472,1.);
#9018=VECTOR('',#31473,1.);
#9019=VECTOR('',#31476,1.);
#9020=VECTOR('',#31483,1.);
#9021=VECTOR('',#31484,1.);
#9022=VECTOR('',#31485,1.);
#9023=VECTOR('',#31488,1.);
#9024=VECTOR('',#31495,1.);
#9025=VECTOR('',#31496,1.);
#9026=VECTOR('',#31499,1.);
#9027=VECTOR('',#31506,1.);
#9028=VECTOR('',#31507,1.);
#9029=VECTOR('',#31510,1.);
#9030=VECTOR('',#31511,1.);
#9031=VECTOR('',#31512,1.);
#9032=VECTOR('',#31517,1.);
#9033=VECTOR('',#31518,1.);
#9034=VECTOR('',#31521,1.);
#9035=VECTOR('',#31522,1.);
#9036=VECTOR('',#31523,1.);
#9037=VECTOR('',#31526,1.);
#9038=VECTOR('',#31527,1.);
#9039=VECTOR('',#31530,1.);
#9040=VECTOR('',#31533,1.);
#9041=VECTOR('',#31536,1.);
#9042=VECTOR('',#31539,1.);
#9043=VECTOR('',#31544,1.);
#9044=VECTOR('',#31545,1.);
#9045=VECTOR('',#31550,1.);
#9046=VECTOR('',#31551,1.);
#9047=VECTOR('',#31552,1.);
#9048=VECTOR('',#31555,1.);
#9049=VECTOR('',#31560,1.);
#9050=VECTOR('',#31561,1.);
#9051=VECTOR('',#31564,1.);
#9052=VECTOR('',#31571,1.);
#9053=VECTOR('',#31572,1.);
#9054=VECTOR('',#31573,1.);
#9055=VECTOR('',#31576,1.);
#9056=VECTOR('',#31583,1.);
#9057=VECTOR('',#31584,1.);
#9058=VECTOR('',#31587,1.);
#9059=VECTOR('',#31588,1.);
#9060=VECTOR('',#31591,1.);
#9061=VECTOR('',#31592,1.);
#9062=VECTOR('',#31593,1.);
#9063=VECTOR('',#31606,1.);
#9064=VECTOR('',#31609,1.);
#9065=VECTOR('',#31612,1.);
#9066=VECTOR('',#31615,1.);
#9067=VECTOR('',#31618,1.);
#9068=VECTOR('',#31619,1.);
#9069=VECTOR('',#31622,1.);
#9070=VECTOR('',#31627,1.);
#9071=VECTOR('',#31630,1.8);
#9072=VECTOR('',#31637,1.);
#9073=VECTOR('',#31638,1.);
#9074=VECTOR('',#31639,1.);
#9075=VECTOR('',#31644,1.);
#9076=VECTOR('',#31647,1.);
#9077=VECTOR('',#31648,1.);
#9078=VECTOR('',#31653,1.);
#9079=VECTOR('',#31656,1.);
#9080=VECTOR('',#31661,1.);
#9081=VECTOR('',#31664,1.);
#9082=VECTOR('',#31665,1.);
#9083=VECTOR('',#31672,1.);
#9084=VECTOR('',#31677,1.);
#9085=VECTOR('',#31678,1.);
#9086=VECTOR('',#31681,1.);
#9087=VECTOR('',#31682,1.);
#9088=VECTOR('',#31683,1.);
#9089=VECTOR('',#31688,1.);
#9090=VECTOR('',#31691,1.);
#9091=VECTOR('',#31694,1.);
#9092=VECTOR('',#31695,1.);
#9093=VECTOR('',#31702,1.);
#9094=VECTOR('',#31703,1.);
#9095=VECTOR('',#31706,1.);
#9096=VECTOR('',#31709,1.);
#9097=VECTOR('',#31712,1.);
#9098=VECTOR('',#31715,1.);
#9099=VECTOR('',#31718,1.);
#9100=VECTOR('',#31723,1.);
#9101=VECTOR('',#31724,1.);
#9102=VECTOR('',#31731,1.);
#9103=VECTOR('',#31734,1.);
#9104=VECTOR('',#31737,1.);
#9105=VECTOR('',#31738,1.);
#9106=VECTOR('',#31741,1.);
#9107=VECTOR('',#31742,1.);
#9108=VECTOR('',#31745,1.);
#9109=VECTOR('',#31750,1.);
#9110=VECTOR('',#31751,1.);
#9111=VECTOR('',#31752,1.);
#9112=VECTOR('',#31755,1.8);
#9113=VECTOR('',#31760,1.);
#9114=VECTOR('',#31761,1.);
#9115=VECTOR('',#31764,1.);
#9116=VECTOR('',#31765,1.);
#9117=VECTOR('',#31766,1.);
#9118=VECTOR('',#31767,1.);
#9119=VECTOR('',#31770,1.);
#9120=VECTOR('',#31775,1.);
#9121=VECTOR('',#31778,1.8);
#9122=VECTOR('',#31783,1.);
#9123=VECTOR('',#31784,1.);
#9124=VECTOR('',#31787,1.);
#9125=VECTOR('',#31788,1.);
#9126=VECTOR('',#31791,1.);
#9127=VECTOR('',#31796,1.);
#9128=VECTOR('',#31797,1.);
#9129=VECTOR('',#31798,1.);
#9130=VECTOR('',#31801,1.8);
#9131=VECTOR('',#31806,1.);
#9132=VECTOR('',#31807,1.);
#9133=VECTOR('',#31810,1.);
#9134=VECTOR('',#31811,1.);
#9135=VECTOR('',#31816,0.555);
#9136=VECTOR('',#31821,0.504999999999999);
#9137=VECTOR('',#31832,0.555);
#9138=VECTOR('',#31835,1.);
#9139=VECTOR('',#31840,0.555);
#9140=VECTOR('',#31845,0.504999999999999);
#9141=VECTOR('',#31850,0.555);
#9142=VECTOR('',#31851,1.);
#9143=VECTOR('',#31852,1.);
#9144=VECTOR('',#31853,1.);
#9145=VECTOR('',#31854,1.);
#9146=VECTOR('',#31855,1.);
#9147=VECTOR('',#31856,1.);
#9148=VECTOR('',#31857,1.);
#9149=VECTOR('',#31858,1.);
#9150=VECTOR('',#31859,1.);
#9151=VECTOR('',#31860,1.);
#9152=VECTOR('',#31861,1.);
#9153=VECTOR('',#31862,1.);
#9154=VECTOR('',#31863,1.);
#9155=VECTOR('',#31864,1.);
#9156=VECTOR('',#31865,1.);
#9157=VECTOR('',#31866,1.);
#9158=VECTOR('',#31867,1.);
#9159=VECTOR('',#31868,1.);
#9160=VECTOR('',#31873,1.);
#9161=VECTOR('',#31874,1.);
#9162=VECTOR('',#31875,1.);
#9163=VECTOR('',#31878,1.);
#9164=VECTOR('',#31879,1.);
#9165=VECTOR('',#31882,1.);
#9166=VECTOR('',#31883,1.);
#9167=VECTOR('',#31886,1.);
#9168=VECTOR('',#31887,1.);
#9169=VECTOR('',#31890,1.);
#9170=VECTOR('',#31891,1.);
#9171=VECTOR('',#31894,1.);
#9172=VECTOR('',#31895,1.);
#9173=VECTOR('',#31898,1.);
#9174=VECTOR('',#31899,1.);
#9175=VECTOR('',#31902,1.);
#9176=VECTOR('',#31905,1.);
#9177=VECTOR('',#31906,1.);
#9178=VECTOR('',#31907,1.);
#9179=VECTOR('',#31908,1.);
#9180=VECTOR('',#31909,1.);
#9181=VECTOR('',#31910,1.);
#9182=VECTOR('',#31911,1.);
#9183=VECTOR('',#31912,1.);
#9184=VECTOR('',#31913,1.);
#9185=VECTOR('',#31914,1.);
#9186=VECTOR('',#31915,1.);
#9187=VECTOR('',#31916,1.);
#9188=VECTOR('',#31917,1.);
#9189=VECTOR('',#31918,1.);
#9190=VECTOR('',#31919,1.);
#9191=VECTOR('',#31920,1.);
#9192=VECTOR('',#31921,1.);
#9193=VECTOR('',#31922,1.);
#9194=VECTOR('',#31923,1.);
#9195=VECTOR('',#31924,1.);
#9196=VECTOR('',#31925,1.);
#9197=VECTOR('',#31926,1.);
#9198=VECTOR('',#31931,1.);
#9199=VECTOR('',#31932,1.);
#9200=VECTOR('',#31933,1.);
#9201=VECTOR('',#31934,1.);
#9202=VECTOR('',#31935,1.);
#9203=VECTOR('',#31936,1.);
#9204=VECTOR('',#31937,1.);
#9205=VECTOR('',#31938,1.);
#9206=VECTOR('',#31939,1.);
#9207=VECTOR('',#31940,1.);
#9208=VECTOR('',#31941,1.);
#9209=VECTOR('',#31942,1.);
#9210=VECTOR('',#31943,1.);
#9211=VECTOR('',#31946,1.);
#9212=VECTOR('',#31947,1.);
#9213=VECTOR('',#31948,1.);
#9214=VECTOR('',#31949,1.);
#9215=VECTOR('',#31950,1.);
#9216=VECTOR('',#31951,1.);
#9217=VECTOR('',#31952,1.);
#9218=VECTOR('',#31953,1.);
#9219=VECTOR('',#31954,1.);
#9220=VECTOR('',#31955,1.);
#9221=VECTOR('',#31958,1.);
#9222=VECTOR('',#31959,1.);
#9223=VECTOR('',#31962,1.);
#9224=VECTOR('',#31967,1.);
#9225=VECTOR('',#31968,1.);
#9226=VECTOR('',#31969,1.);
#9227=VECTOR('',#31972,1.);
#9228=VECTOR('',#31973,1.);
#9229=VECTOR('',#31976,1.);
#9230=VECTOR('',#31977,1.);
#9231=VECTOR('',#31980,1.);
#9232=VECTOR('',#31981,1.);
#9233=VECTOR('',#31984,1.);
#9234=VECTOR('',#31985,1.);
#9235=VECTOR('',#31988,1.);
#9236=VECTOR('',#31989,1.);
#9237=VECTOR('',#31992,1.);
#9238=VECTOR('',#31993,1.);
#9239=VECTOR('',#31996,1.);
#9240=VECTOR('',#31997,1.);
#9241=VECTOR('',#32000,1.);
#9242=VECTOR('',#32001,1.);
#9243=VECTOR('',#32004,1.);
#9244=VECTOR('',#32013,1.);
#9245=VECTOR('',#32016,1.);
#11278=VERTEX_POINT('',#37680);
#11279=VERTEX_POINT('',#37681);
#11280=VERTEX_POINT('',#37683);
#11281=VERTEX_POINT('',#37685);
#11282=VERTEX_POINT('',#37687);
#11283=VERTEX_POINT('',#37691);
#11284=VERTEX_POINT('',#37693);
#11285=VERTEX_POINT('',#37695);
#11286=VERTEX_POINT('',#37697);
#11287=VERTEX_POINT('',#37701);
#11288=VERTEX_POINT('',#37705);
#11289=VERTEX_POINT('',#37709);
#11290=VERTEX_POINT('',#37713);
#11291=VERTEX_POINT('',#37715);
#11292=VERTEX_POINT('',#37717);
#11293=VERTEX_POINT('',#37721);
#11294=VERTEX_POINT('',#37723);
#11295=VERTEX_POINT('',#37725);
#11296=VERTEX_POINT('',#37727);
#11297=VERTEX_POINT('',#37729);
#11298=VERTEX_POINT('',#37733);
#11299=VERTEX_POINT('',#37734);
#11300=VERTEX_POINT('',#37736);
#11301=VERTEX_POINT('',#37738);
#11302=VERTEX_POINT('',#37740);
#11303=VERTEX_POINT('',#37744);
#11304=VERTEX_POINT('',#37746);
#11305=VERTEX_POINT('',#37750);
#11306=VERTEX_POINT('',#37761);
#11307=VERTEX_POINT('',#37766);
#11308=VERTEX_POINT('',#37768);
#11309=VERTEX_POINT('',#37772);
#11310=VERTEX_POINT('',#37773);
#11311=VERTEX_POINT('',#37775);
#11312=VERTEX_POINT('',#37777);
#11313=VERTEX_POINT('',#37780);
#11314=VERTEX_POINT('',#37782);
#11315=VERTEX_POINT('',#37784);
#11316=VERTEX_POINT('',#37787);
#11317=VERTEX_POINT('',#37791);
#11318=VERTEX_POINT('',#37795);
#11319=VERTEX_POINT('',#37799);
#11320=VERTEX_POINT('',#37803);
#11321=VERTEX_POINT('',#37807);
#11322=VERTEX_POINT('',#37811);
#11323=VERTEX_POINT('',#37815);
#11324=VERTEX_POINT('',#37819);
#11325=VERTEX_POINT('',#37820);
#11326=VERTEX_POINT('',#37822);
#11327=VERTEX_POINT('',#37824);
#11328=VERTEX_POINT('',#37827);
#11329=VERTEX_POINT('',#37829);
#11330=VERTEX_POINT('',#37831);
#11331=VERTEX_POINT('',#37840);
#11332=VERTEX_POINT('',#37842);
#11333=VERTEX_POINT('',#37846);
#11334=VERTEX_POINT('',#37847);
#11335=VERTEX_POINT('',#37849);
#11336=VERTEX_POINT('',#37851);
#11337=VERTEX_POINT('',#37854);
#11338=VERTEX_POINT('',#37856);
#11339=VERTEX_POINT('',#37858);
#11340=VERTEX_POINT('',#37861);
#11341=VERTEX_POINT('',#37865);
#11342=VERTEX_POINT('',#37869);
#11343=VERTEX_POINT('',#37873);
#11344=VERTEX_POINT('',#37877);
#11345=VERTEX_POINT('',#37881);
#11346=VERTEX_POINT('',#37885);
#11347=VERTEX_POINT('',#37889);
#11348=VERTEX_POINT('',#37890);
#11349=VERTEX_POINT('',#37892);
#11350=VERTEX_POINT('',#37894);
#11351=VERTEX_POINT('',#37896);
#11352=VERTEX_POINT('',#37935);
#11353=VERTEX_POINT('',#37936);
#11354=VERTEX_POINT('',#37938);
#11355=VERTEX_POINT('',#37948);
#11356=VERTEX_POINT('',#38008);
#11357=VERTEX_POINT('',#38010);
#11358=VERTEX_POINT('',#38012);
#11359=VERTEX_POINT('',#38014);
#11360=VERTEX_POINT('',#38016);
#11361=VERTEX_POINT('',#38018);
#11362=VERTEX_POINT('',#38023);
#11363=VERTEX_POINT('',#38034);
#11364=VERTEX_POINT('',#38041);
#11365=VERTEX_POINT('',#38043);
#11366=VERTEX_POINT('',#38045);
#11367=VERTEX_POINT('',#38050);
#11368=VERTEX_POINT('',#38088);
#11369=VERTEX_POINT('',#38095);
#11370=VERTEX_POINT('',#38099);
#11371=VERTEX_POINT('',#38100);
#11372=VERTEX_POINT('',#38102);
#11373=VERTEX_POINT('',#38104);
#11374=VERTEX_POINT('',#38107);
#11375=VERTEX_POINT('',#38109);
#11376=VERTEX_POINT('',#38111);
#11377=VERTEX_POINT('',#38120);
#11378=VERTEX_POINT('',#38121);
#11379=VERTEX_POINT('',#38123);
#11380=VERTEX_POINT('',#38125);
#11381=VERTEX_POINT('',#38129);
#11382=VERTEX_POINT('',#38134);
#11383=VERTEX_POINT('',#38138);
#11384=VERTEX_POINT('',#38140);
#11385=VERTEX_POINT('',#38144);
#11386=VERTEX_POINT('',#38149);
#11387=VERTEX_POINT('',#38153);
#11388=VERTEX_POINT('',#38154);
#11389=VERTEX_POINT('',#38163);
#11390=VERTEX_POINT('',#38165);
#11391=VERTEX_POINT('',#38171);
#11392=VERTEX_POINT('',#38173);
#11393=VERTEX_POINT('',#38178);
#11394=VERTEX_POINT('',#38189);
#11395=VERTEX_POINT('',#38194);
#11396=VERTEX_POINT('',#38196);
#11397=VERTEX_POINT('',#38201);
#11398=VERTEX_POINT('',#38213);
#11399=VERTEX_POINT('',#38218);
#11400=VERTEX_POINT('',#38220);
#11401=VERTEX_POINT('',#38224);
#11402=VERTEX_POINT('',#38225);
#11403=VERTEX_POINT('',#38227);
#11404=VERTEX_POINT('',#38229);
#11405=VERTEX_POINT('',#38231);
#11406=VERTEX_POINT('',#38233);
#11407=VERTEX_POINT('',#38235);
#11408=VERTEX_POINT('',#38237);
#11409=VERTEX_POINT('',#38241);
#11410=VERTEX_POINT('',#38243);
#11411=VERTEX_POINT('',#38247);
#11412=VERTEX_POINT('',#38252);
#11413=VERTEX_POINT('',#38256);
#11414=VERTEX_POINT('',#38260);
#11415=VERTEX_POINT('',#38261);
#11416=VERTEX_POINT('',#38266);
#11417=VERTEX_POINT('',#38271);
#11418=VERTEX_POINT('',#38283);
#11419=VERTEX_POINT('',#38284);
#11420=VERTEX_POINT('',#38288);
#11421=VERTEX_POINT('',#38292);
#11422=VERTEX_POINT('',#38296);
#11423=VERTEX_POINT('',#38300);
#11424=VERTEX_POINT('',#38304);
#11425=VERTEX_POINT('',#38308);
#11426=VERTEX_POINT('',#38312);
#11427=VERTEX_POINT('',#38316);
#11428=VERTEX_POINT('',#38323);
#11429=VERTEX_POINT('',#38324);
#11430=VERTEX_POINT('',#38326);
#11431=VERTEX_POINT('',#38328);
#11432=VERTEX_POINT('',#38330);
#11433=VERTEX_POINT('',#38332);
#11434=VERTEX_POINT('',#38334);
#11435=VERTEX_POINT('',#38336);
#11436=VERTEX_POINT('',#38339);
#11437=VERTEX_POINT('',#38340);
#11438=VERTEX_POINT('',#38344);
#11439=VERTEX_POINT('',#38348);
#11440=VERTEX_POINT('',#38352);
#11441=VERTEX_POINT('',#38356);
#11442=VERTEX_POINT('',#38360);
#11443=VERTEX_POINT('',#38364);
#11444=VERTEX_POINT('',#38368);
#11445=VERTEX_POINT('',#38372);
#11446=VERTEX_POINT('',#38376);
#11447=VERTEX_POINT('',#38380);
#11448=VERTEX_POINT('',#38384);
#11449=VERTEX_POINT('',#38391);
#11450=VERTEX_POINT('',#38392);
#11451=VERTEX_POINT('',#38394);
#11452=VERTEX_POINT('',#38396);
#11453=VERTEX_POINT('',#38398);
#11454=VERTEX_POINT('',#38402);
#11455=VERTEX_POINT('',#38406);
#11456=VERTEX_POINT('',#38410);
#11457=VERTEX_POINT('',#38414);
#11458=VERTEX_POINT('',#38418);
#11459=VERTEX_POINT('',#38422);
#11460=VERTEX_POINT('',#38426);
#11461=VERTEX_POINT('',#38430);
#11462=VERTEX_POINT('',#38432);
#11463=VERTEX_POINT('',#38436);
#11464=VERTEX_POINT('',#38440);
#11465=VERTEX_POINT('',#38444);
#11466=VERTEX_POINT('',#38448);
#11467=VERTEX_POINT('',#38452);
#11468=VERTEX_POINT('',#38456);
#11469=VERTEX_POINT('',#38460);
#11470=VERTEX_POINT('',#38464);
#11471=VERTEX_POINT('',#38471);
#11472=VERTEX_POINT('',#38472);
#11473=VERTEX_POINT('',#38474);
#11474=VERTEX_POINT('',#38476);
#11475=VERTEX_POINT('',#38478);
#11476=VERTEX_POINT('',#38480);
#11477=VERTEX_POINT('',#38482);
#11478=VERTEX_POINT('',#38484);
#11479=VERTEX_POINT('',#38486);
#11480=VERTEX_POINT('',#38488);
#11481=VERTEX_POINT('',#38492);
#11482=VERTEX_POINT('',#38493);
#11483=VERTEX_POINT('',#38495);
#11484=VERTEX_POINT('',#38497);
#11485=VERTEX_POINT('',#38499);
#11486=VERTEX_POINT('',#38501);
#11487=VERTEX_POINT('',#38503);
#11488=VERTEX_POINT('',#38505);
#11489=VERTEX_POINT('',#38509);
#11490=VERTEX_POINT('',#38511);
#11491=VERTEX_POINT('',#38513);
#11492=VERTEX_POINT('',#38560);
#11493=VERTEX_POINT('',#38562);
#11494=VERTEX_POINT('',#38616);
#11495=VERTEX_POINT('',#38618);
#11496=VERTEX_POINT('',#38620);
#11497=VERTEX_POINT('',#38625);
#11498=VERTEX_POINT('',#38657);
#11499=VERTEX_POINT('',#38664);
#11500=VERTEX_POINT('',#38666);
#11501=VERTEX_POINT('',#38668);
#11502=VERTEX_POINT('',#38711);
#11503=VERTEX_POINT('',#38713);
#11504=VERTEX_POINT('',#38766);
#11505=VERTEX_POINT('',#38768);
#11506=VERTEX_POINT('',#38770);
#11507=VERTEX_POINT('',#38775);
#11508=VERTEX_POINT('',#38813);
#11509=VERTEX_POINT('',#38820);
#11510=VERTEX_POINT('',#38822);
#11511=VERTEX_POINT('',#38826);
#11512=VERTEX_POINT('',#38830);
#11513=VERTEX_POINT('',#38839);
#11514=VERTEX_POINT('',#38843);
#11515=VERTEX_POINT('',#38849);
#11516=VERTEX_POINT('',#38853);
#11517=VERTEX_POINT('',#38857);
#11518=VERTEX_POINT('',#38859);
#11519=VERTEX_POINT('',#38864);
#11520=VERTEX_POINT('',#38875);
#11521=VERTEX_POINT('',#38891);
#11522=VERTEX_POINT('',#38897);
#11523=VERTEX_POINT('',#38902);
#11524=VERTEX_POINT('',#38907);
#11525=VERTEX_POINT('',#38909);
#11526=VERTEX_POINT('',#38914);
#11527=VERTEX_POINT('',#38925);
#11528=VERTEX_POINT('',#38938);
#11529=VERTEX_POINT('',#38945);
#11530=VERTEX_POINT('',#38950);
#11531=VERTEX_POINT('',#38955);
#11532=VERTEX_POINT('',#38959);
#11533=VERTEX_POINT('',#38961);
#11534=VERTEX_POINT('',#38963);
#11535=VERTEX_POINT('',#38965);
#11536=VERTEX_POINT('',#38967);
#11537=VERTEX_POINT('',#39093);
#11538=VERTEX_POINT('',#39097);
#11539=VERTEX_POINT('',#39115);
#11540=VERTEX_POINT('',#39120);
#11541=VERTEX_POINT('',#39131);
#11542=VERTEX_POINT('',#39148);
#11543=VERTEX_POINT('',#39154);
#11544=VERTEX_POINT('',#39163);
#11545=VERTEX_POINT('',#39168);
#11546=VERTEX_POINT('',#39179);
#11547=VERTEX_POINT('',#39198);
#11548=VERTEX_POINT('',#39205);
#11549=VERTEX_POINT('',#39469);
#11550=VERTEX_POINT('',#39471);
#11551=VERTEX_POINT('',#39473);
#11552=VERTEX_POINT('',#39516);
#11553=VERTEX_POINT('',#39518);
#11554=VERTEX_POINT('',#39571);
#11555=VERTEX_POINT('',#39573);
#11556=VERTEX_POINT('',#39575);
#11557=VERTEX_POINT('',#39580);
#11558=VERTEX_POINT('',#39612);
#11559=VERTEX_POINT('',#39728);
#11560=VERTEX_POINT('',#39729);
#11561=VERTEX_POINT('',#39731);
#11562=VERTEX_POINT('',#39733);
#11563=VERTEX_POINT('',#39737);
#11564=VERTEX_POINT('',#39738);
#11565=VERTEX_POINT('',#39743);
#11566=VERTEX_POINT('',#39744);
#11567=VERTEX_POINT('',#39749);
#11568=VERTEX_POINT('',#39750);
#11569=VERTEX_POINT('',#39755);
#11570=VERTEX_POINT('',#39760);
#11571=VERTEX_POINT('',#39764);
#11572=VERTEX_POINT('',#39765);
#11573=VERTEX_POINT('',#39773);
#11574=VERTEX_POINT('',#39776);
#11575=VERTEX_POINT('',#39780);
#11576=VERTEX_POINT('',#39784);
#11577=VERTEX_POINT('',#39786);
#11578=VERTEX_POINT('',#39791);
#11579=VERTEX_POINT('',#39802);
#11580=VERTEX_POINT('',#39807);
#11581=VERTEX_POINT('',#39809);
#11582=VERTEX_POINT('',#39814);
#11583=VERTEX_POINT('',#39825);
#11584=VERTEX_POINT('',#39830);
#11585=VERTEX_POINT('',#39832);
#11586=VERTEX_POINT('',#39837);
#11587=VERTEX_POINT('',#39838);
#11588=VERTEX_POINT('',#39840);
#11589=VERTEX_POINT('',#39842);
#11590=VERTEX_POINT('',#39844);
#11591=VERTEX_POINT('',#39846);
#11592=VERTEX_POINT('',#39848);
#11593=VERTEX_POINT('',#39850);
#11594=VERTEX_POINT('',#39854);
#11595=VERTEX_POINT('',#39856);
#11596=VERTEX_POINT('',#39860);
#11597=VERTEX_POINT('',#39865);
#11598=VERTEX_POINT('',#39869);
#11599=VERTEX_POINT('',#39873);
#11600=VERTEX_POINT('',#39874);
#11601=VERTEX_POINT('',#39879);
#11602=VERTEX_POINT('',#39881);
#11603=VERTEX_POINT('',#39885);
#11604=VERTEX_POINT('',#39886);
#11605=VERTEX_POINT('',#39897);
#11606=VERTEX_POINT('',#39899);
#11607=VERTEX_POINT('',#39904);
#11608=VERTEX_POINT('',#39915);
#11609=VERTEX_POINT('',#39920);
#11610=VERTEX_POINT('',#39922);
#11611=VERTEX_POINT('',#39927);
#11612=VERTEX_POINT('',#39939);
#11613=VERTEX_POINT('',#39951);
#11614=VERTEX_POINT('',#39952);
#11615=VERTEX_POINT('',#39954);
#11616=VERTEX_POINT('',#39956);
#11617=VERTEX_POINT('',#39958);
#11618=VERTEX_POINT('',#39960);
#11619=VERTEX_POINT('',#39962);
#11620=VERTEX_POINT('',#39964);
#11621=VERTEX_POINT('',#40007);
#11622=VERTEX_POINT('',#40009);
#11623=VERTEX_POINT('',#40022);
#11624=VERTEX_POINT('',#40024);
#11625=VERTEX_POINT('',#40026);
#11626=VERTEX_POINT('',#40070);
#11627=VERTEX_POINT('',#40072);
#11628=VERTEX_POINT('',#40074);
#11629=VERTEX_POINT('',#40079);
#11630=VERTEX_POINT('',#40114);
#11631=VERTEX_POINT('',#40121);
#11632=VERTEX_POINT('',#40123);
#11633=VERTEX_POINT('',#40127);
#11634=VERTEX_POINT('',#40131);
#11635=VERTEX_POINT('',#40140);
#11636=VERTEX_POINT('',#40144);
#11637=VERTEX_POINT('',#40150);
#11638=VERTEX_POINT('',#40154);
#11639=VERTEX_POINT('',#40158);
#11640=VERTEX_POINT('',#40160);
#11641=VERTEX_POINT('',#40165);
#11642=VERTEX_POINT('',#40176);
#11643=VERTEX_POINT('',#40191);
#11644=VERTEX_POINT('',#40198);
#11645=VERTEX_POINT('',#40203);
#11646=VERTEX_POINT('',#40205);
#11647=VERTEX_POINT('',#40210);
#11648=VERTEX_POINT('',#40221);
#11649=VERTEX_POINT('',#40237);
#11650=VERTEX_POINT('',#40243);
#11651=VERTEX_POINT('',#40248);
#11652=VERTEX_POINT('',#40253);
#11653=VERTEX_POINT('',#40257);
#11654=VERTEX_POINT('',#40259);
#11655=VERTEX_POINT('',#40261);
#11656=VERTEX_POINT('',#40263);
#11657=VERTEX_POINT('',#40265);
#11658=VERTEX_POINT('',#40282);
#11659=VERTEX_POINT('',#40286);
#11660=VERTEX_POINT('',#40296);
#11661=VERTEX_POINT('',#40301);
#11662=VERTEX_POINT('',#40312);
#11663=VERTEX_POINT('',#40329);
#11664=VERTEX_POINT('',#40339);
#11665=VERTEX_POINT('',#40344);
#11666=VERTEX_POINT('',#40355);
#11667=VERTEX_POINT('',#40370);
#11668=VERTEX_POINT('',#40377);
#11669=VERTEX_POINT('',#40504);
#11670=VERTEX_POINT('',#40506);
#11671=VERTEX_POINT('',#40508);
#11672=VERTEX_POINT('',#40551);
#11673=VERTEX_POINT('',#40553);
#11674=VERTEX_POINT('',#40606);
#11675=VERTEX_POINT('',#40608);
#11676=VERTEX_POINT('',#40610);
#11677=VERTEX_POINT('',#40615);
#11678=VERTEX_POINT('',#40647);
#11679=VERTEX_POINT('',#40814);
#11680=VERTEX_POINT('',#40816);
#11681=VERTEX_POINT('',#40830);
#11682=VERTEX_POINT('',#40832);
#11683=VERTEX_POINT('',#40834);
#11684=VERTEX_POINT('',#40878);
#11685=VERTEX_POINT('',#40880);
#11686=VERTEX_POINT('',#40882);
#11687=VERTEX_POINT('',#40887);
#11688=VERTEX_POINT('',#40919);
#11689=VERTEX_POINT('',#41047);
#11690=VERTEX_POINT('',#41049);
#11691=VERTEX_POINT('',#41051);
#11692=VERTEX_POINT('',#41094);
#11693=VERTEX_POINT('',#41096);
#11694=VERTEX_POINT('',#41149);
#11695=VERTEX_POINT('',#41151);
#11696=VERTEX_POINT('',#41153);
#11697=VERTEX_POINT('',#41158);
#11698=VERTEX_POINT('',#41190);
#11699=VERTEX_POINT('',#41314);
#11700=VERTEX_POINT('',#41316);
#11701=VERTEX_POINT('',#41320);
#11702=VERTEX_POINT('',#41324);
#11703=VERTEX_POINT('',#41327);
#11704=VERTEX_POINT('',#41332);
#11705=VERTEX_POINT('',#41335);
#11706=VERTEX_POINT('',#41339);
#11707=VERTEX_POINT('',#41350);
#11708=VERTEX_POINT('',#41351);
#11709=VERTEX_POINT('',#41355);
#11710=VERTEX_POINT('',#41357);
#11711=VERTEX_POINT('',#41368);
#11712=VERTEX_POINT('',#41372);
#11713=VERTEX_POINT('',#41383);
#11714=VERTEX_POINT('',#41387);
#11715=VERTEX_POINT('',#41398);
#11716=VERTEX_POINT('',#41402);
#11717=VERTEX_POINT('',#41413);
#11718=VERTEX_POINT('',#41417);
#11719=VERTEX_POINT('',#41428);
#11720=VERTEX_POINT('',#41432);
#11721=VERTEX_POINT('',#41443);
#11722=VERTEX_POINT('',#41447);
#11723=VERTEX_POINT('',#41470);
#11724=VERTEX_POINT('',#41472);
#11725=VERTEX_POINT('',#41483);
#11726=VERTEX_POINT('',#41494);
#11727=VERTEX_POINT('',#41505);
#11728=VERTEX_POINT('',#41516);
#11729=VERTEX_POINT('',#41527);
#11730=VERTEX_POINT('',#41538);
#11731=VERTEX_POINT('',#41549);
#11732=VERTEX_POINT('',#41560);
#11733=VERTEX_POINT('',#41576);
#11734=VERTEX_POINT('',#41578);
#11735=VERTEX_POINT('',#41582);
#11736=VERTEX_POINT('',#41586);
#11737=VERTEX_POINT('',#41590);
#11738=VERTEX_POINT('',#41594);
#11739=VERTEX_POINT('',#41598);
#11740=VERTEX_POINT('',#41602);
#11741=VERTEX_POINT('',#41614);
#11742=VERTEX_POINT('',#41615);
#11743=VERTEX_POINT('',#41619);
#11744=VERTEX_POINT('',#41621);
#11745=VERTEX_POINT('',#41632);
#11746=VERTEX_POINT('',#41636);
#11747=VERTEX_POINT('',#41647);
#11748=VERTEX_POINT('',#41651);
#11749=VERTEX_POINT('',#41662);
#11750=VERTEX_POINT('',#41666);
#11751=VERTEX_POINT('',#41677);
#11752=VERTEX_POINT('',#41681);
#11753=VERTEX_POINT('',#41692);
#11754=VERTEX_POINT('',#41696);
#11755=VERTEX_POINT('',#41707);
#11756=VERTEX_POINT('',#41711);
#11757=VERTEX_POINT('',#41722);
#11758=VERTEX_POINT('',#41726);
#11759=VERTEX_POINT('',#41749);
#11760=VERTEX_POINT('',#41751);
#11761=VERTEX_POINT('',#41762);
#11762=VERTEX_POINT('',#41773);
#11763=VERTEX_POINT('',#41784);
#11764=VERTEX_POINT('',#41795);
#11765=VERTEX_POINT('',#41806);
#11766=VERTEX_POINT('',#41817);
#11767=VERTEX_POINT('',#41828);
#11768=VERTEX_POINT('',#41839);
#11769=VERTEX_POINT('',#41850);
#11770=VERTEX_POINT('',#41861);
#11771=VERTEX_POINT('',#41872);
#11772=VERTEX_POINT('',#41888);
#11773=VERTEX_POINT('',#41890);
#11774=VERTEX_POINT('',#41899);
#11775=VERTEX_POINT('',#41910);
#11776=VERTEX_POINT('',#41921);
#11777=VERTEX_POINT('',#41932);
#11778=VERTEX_POINT('',#41943);
#11779=VERTEX_POINT('',#41954);
#11780=VERTEX_POINT('',#41965);
#11781=VERTEX_POINT('',#41976);
#11782=VERTEX_POINT('',#41987);
#11783=VERTEX_POINT('',#41998);
#11784=VERTEX_POINT('',#42004);
#11785=VERTEX_POINT('',#42013);
#11786=VERTEX_POINT('',#42024);
#11787=VERTEX_POINT('',#42035);
#11788=VERTEX_POINT('',#42046);
#11789=VERTEX_POINT('',#42057);
#11790=VERTEX_POINT('',#42068);
#11791=VERTEX_POINT('',#42079);
#11792=VERTEX_POINT('',#42090);
#11793=VERTEX_POINT('',#42096);
#11794=VERTEX_POINT('',#42103);
#11795=VERTEX_POINT('',#42105);
#11796=VERTEX_POINT('',#42109);
#11797=VERTEX_POINT('',#42113);
#11798=VERTEX_POINT('',#42117);
#11799=VERTEX_POINT('',#42121);
#11800=VERTEX_POINT('',#42125);
#11801=VERTEX_POINT('',#42129);
#11802=VERTEX_POINT('',#42133);
#11803=VERTEX_POINT('',#42137);
#13843=EDGE_CURVE('',#11278,#11279,#6302,.T.);
#13844=EDGE_CURVE('',#11279,#11280,#6303,.T.);
#13845=EDGE_CURVE('',#11280,#11281,#6304,.T.);
#13846=EDGE_CURVE('',#11281,#11282,#6305,.T.);
#13847=EDGE_CURVE('',#11282,#11278,#6306,.T.);
#13848=EDGE_CURVE('',#11280,#11283,#6307,.T.);
#13849=EDGE_CURVE('',#11284,#11283,#6308,.T.);
#13850=EDGE_CURVE('',#11285,#11284,#6309,.T.);
#13851=EDGE_CURVE('',#11285,#11286,#6310,.T.);
#13852=EDGE_CURVE('',#11281,#11286,#6311,.T.);
#13853=EDGE_CURVE('',#11287,#11279,#6312,.T.);
#13854=EDGE_CURVE('',#11283,#11287,#6313,.T.);
#13855=EDGE_CURVE('',#11278,#11288,#6314,.T.);
#13856=EDGE_CURVE('',#11288,#11287,#6315,.T.);
#13857=EDGE_CURVE('',#11288,#11289,#6316,.T.);
#13858=EDGE_CURVE('',#11289,#11284,#6317,.T.);
#13859=EDGE_CURVE('',#11289,#11290,#6318,.T.);
#13860=EDGE_CURVE('',#11291,#11290,#6319,.T.);
#13861=EDGE_CURVE('',#11292,#11291,#6320,.T.);
#13862=EDGE_CURVE('',#11292,#11285,#6321,.T.);
#13863=EDGE_CURVE('',#11293,#11288,#6322,.T.);
#13864=EDGE_CURVE('',#11294,#11293,#6323,.T.);
#13865=EDGE_CURVE('',#11295,#11294,#6324,.T.);
#13866=EDGE_CURVE('',#11296,#11295,#6325,.T.);
#13867=EDGE_CURVE('',#11297,#11296,#6326,.T.);
#13868=EDGE_CURVE('',#11290,#11297,#6327,.T.);
#13869=EDGE_CURVE('',#11298,#11299,#6328,.T.);
#13870=EDGE_CURVE('',#11299,#11300,#6329,.T.);
#13871=EDGE_CURVE('',#11300,#11301,#6330,.T.);
#13872=EDGE_CURVE('',#11301,#11302,#6331,.T.);
#13873=EDGE_CURVE('',#11302,#11298,#6332,.T.);
#13874=EDGE_CURVE('',#11303,#11302,#6333,.T.);
#13875=EDGE_CURVE('',#11304,#11303,#6334,.T.);
#13876=EDGE_CURVE('',#11298,#11304,#6335,.T.);
#13877=EDGE_CURVE('',#11305,#11301,#6336,.T.);
#13878=EDGE_CURVE('',#11305,#11292,#6337,.T.);
#13879=EDGE_CURVE('',#11303,#11291,#6338,.T.);
#13880=EDGE_CURVE('',#11286,#11305,#6339,.T.);
#13881=EDGE_CURVE('',#11300,#11282,#6340,.T.);
#13882=EDGE_CURVE('',#11304,#11297,#6341,.T.);
#13883=EDGE_CURVE('',#11297,#11299,#6342,.T.);
#13884=EDGE_CURVE('',#11306,#11296,#6343,.T.);
#13885=EDGE_CURVE('',#11306,#11299,#6344,.T.);
#13886=EDGE_CURVE('',#11307,#11307,#2045,.T.);
#13887=EDGE_CURVE('',#11307,#11308,#6345,.T.);
#13888=EDGE_CURVE('',#11308,#11308,#2046,.T.);
#13889=EDGE_CURVE('',#11309,#11310,#6346,.T.);
#13890=EDGE_CURVE('',#11311,#11309,#6347,.T.);
#13891=EDGE_CURVE('',#11312,#11311,#6348,.T.);
#13892=EDGE_CURVE('',#11310,#11312,#6349,.T.);
#13893=EDGE_CURVE('',#11313,#11313,#2047,.T.);
#13894=EDGE_CURVE('',#11314,#11314,#2048,.T.);
#13895=EDGE_CURVE('',#11315,#11315,#2049,.T.);
#13896=EDGE_CURVE('',#11308,#11316,#6350,.T.);
#13897=EDGE_CURVE('',#11316,#11316,#2050,.T.);
#13898=EDGE_CURVE('',#11313,#11317,#6351,.T.);
#13899=EDGE_CURVE('',#11317,#11317,#2051,.T.);
#13900=EDGE_CURVE('',#11317,#11318,#6352,.T.);
#13901=EDGE_CURVE('',#11318,#11318,#2052,.T.);
#13902=EDGE_CURVE('',#11315,#11319,#6353,.T.);
#13903=EDGE_CURVE('',#11319,#11319,#2053,.T.);
#13904=EDGE_CURVE('',#11319,#11320,#6354,.T.);
#13905=EDGE_CURVE('',#11320,#11320,#2054,.T.);
#13906=EDGE_CURVE('',#11314,#11321,#6355,.T.);
#13907=EDGE_CURVE('',#11321,#11321,#2055,.T.);
#13908=EDGE_CURVE('',#11321,#11322,#6356,.T.);
#13909=EDGE_CURVE('',#11322,#11322,#2056,.T.);
#13910=EDGE_CURVE('',#11323,#11323,#2057,.T.);
#13911=EDGE_CURVE('',#11323,#11322,#6357,.T.);
#13912=EDGE_CURVE('',#11324,#11325,#6358,.T.);
#13913=EDGE_CURVE('',#11326,#11324,#6359,.T.);
#13914=EDGE_CURVE('',#11327,#11326,#6360,.T.);
#13915=EDGE_CURVE('',#11325,#11327,#6361,.T.);
#13916=EDGE_CURVE('',#11328,#11328,#2058,.T.);
#13917=EDGE_CURVE('',#11329,#11329,#2059,.T.);
#13918=EDGE_CURVE('',#11330,#11330,#2060,.T.);
#13919=EDGE_CURVE('',#11328,#11320,#6362,.T.);
#13920=EDGE_CURVE('',#11330,#11318,#6363,.T.);
#13921=EDGE_CURVE('',#11329,#11316,#6364,.T.);
#13922=EDGE_CURVE('',#11331,#11331,#2061,.T.);
#13923=EDGE_CURVE('',#11331,#11332,#6365,.T.);
#13924=EDGE_CURVE('',#11332,#11332,#2062,.T.);
#13925=EDGE_CURVE('',#11333,#11334,#6366,.T.);
#13926=EDGE_CURVE('',#11335,#11333,#6367,.T.);
#13927=EDGE_CURVE('',#11336,#11335,#6368,.T.);
#13928=EDGE_CURVE('',#11334,#11336,#6369,.T.);
#13929=EDGE_CURVE('',#11337,#11337,#2063,.T.);
#13930=EDGE_CURVE('',#11338,#11338,#2064,.T.);
#13931=EDGE_CURVE('',#11339,#11339,#2065,.T.);
#13932=EDGE_CURVE('',#11340,#11340,#2066,.T.);
#13933=EDGE_CURVE('',#11340,#11332,#6370,.T.);
#13934=EDGE_CURVE('',#11337,#11341,#6371,.T.);
#13935=EDGE_CURVE('',#11341,#11341,#2067,.T.);
#13936=EDGE_CURVE('',#11342,#11342,#2068,.T.);
#13937=EDGE_CURVE('',#11342,#11341,#6372,.T.);
#13938=EDGE_CURVE('',#11339,#11343,#6373,.T.);
#13939=EDGE_CURVE('',#11343,#11343,#2069,.T.);
#13940=EDGE_CURVE('',#11344,#11344,#2070,.T.);
#13941=EDGE_CURVE('',#11344,#11343,#6374,.T.);
#13942=EDGE_CURVE('',#11338,#11345,#6375,.T.);
#13943=EDGE_CURVE('',#11345,#11345,#2071,.T.);
#13944=EDGE_CURVE('',#11346,#11346,#2072,.T.);
#13945=EDGE_CURVE('',#11346,#11345,#6376,.T.);
#13946=EDGE_CURVE('',#11347,#11348,#6377,.T.);
#13947=EDGE_CURVE('',#11348,#11349,#2073,.T.);
#13948=EDGE_CURVE('',#11349,#11350,#2074,.T.);
#13949=EDGE_CURVE('',#11350,#11351,#6378,.T.);
#13950=EDGE_CURVE('',#11351,#11347,#2075,.T.);
#13951=EDGE_CURVE('',#11352,#11353,#6379,.T.);
#13952=EDGE_CURVE('',#11353,#11354,#551,.T.);
#13953=EDGE_CURVE('',#11354,#11355,#6380,.T.);
#13954=EDGE_CURVE('',#11355,#11352,#552,.T.);
#13955=EDGE_CURVE('',#11354,#11351,#553,.T.);
#13956=EDGE_CURVE('',#11350,#11355,#554,.T.);
#13957=EDGE_CURVE('',#11347,#11353,#555,.T.);
#13958=EDGE_CURVE('',#11352,#11348,#556,.T.);
#13959=EDGE_CURVE('',#11347,#11356,#6381,.T.);
#13960=EDGE_CURVE('',#11357,#11356,#2076,.T.);
#13961=EDGE_CURVE('',#11357,#11358,#6382,.T.);
#13962=EDGE_CURVE('',#11359,#11358,#2077,.T.);
#13963=EDGE_CURVE('',#11359,#11360,#6383,.T.);
#13964=EDGE_CURVE('',#11361,#11360,#557,.T.);
#13965=EDGE_CURVE('',#11362,#11361,#558,.T.);
#13966=EDGE_CURVE('',#11363,#11362,#559,.T.);
#13967=EDGE_CURVE('',#11363,#11351,#6384,.T.);
#13968=EDGE_CURVE('',#11349,#11364,#6385,.T.);
#13969=EDGE_CURVE('',#11365,#11364,#2078,.T.);
#13970=EDGE_CURVE('',#11366,#11365,#560,.T.);
#13971=EDGE_CURVE('',#11367,#11366,#561,.T.);
#13972=EDGE_CURVE('',#11368,#11367,#562,.T.);
#13973=EDGE_CURVE('',#11364,#11368,#2079,.T.);
#13974=EDGE_CURVE('',#11369,#11369,#2080,.T.);
#13975=EDGE_CURVE('',#11369,#11346,#6386,.T.);
#13976=EDGE_CURVE('',#11370,#11371,#6387,.T.);
#13977=EDGE_CURVE('',#11372,#11370,#6388,.T.);
#13978=EDGE_CURVE('',#11373,#11372,#6389,.T.);
#13979=EDGE_CURVE('',#11371,#11373,#6390,.T.);
#13980=EDGE_CURVE('',#11374,#11374,#2081,.T.);
#13981=EDGE_CURVE('',#11375,#11375,#2082,.T.);
#13982=EDGE_CURVE('',#11376,#11376,#2083,.T.);
#13983=EDGE_CURVE('',#11374,#11344,#6391,.T.);
#13984=EDGE_CURVE('',#11376,#11342,#6392,.T.);
#13985=EDGE_CURVE('',#11375,#11340,#6393,.T.);
#13986=EDGE_CURVE('',#11377,#11378,#6394,.T.);
#13987=EDGE_CURVE('',#11378,#11379,#2084,.T.);
#13988=EDGE_CURVE('',#11379,#11380,#6395,.T.);
#13989=EDGE_CURVE('',#11380,#11377,#2085,.T.);
#13990=EDGE_CURVE('',#11377,#11381,#6396,.T.);
#13991=EDGE_CURVE('',#11381,#11356,#6397,.T.);
#13992=EDGE_CURVE('',#11356,#11378,#6398,.T.);
#13993=EDGE_CURVE('',#11382,#11357,#6399,.T.);
#13994=EDGE_CURVE('',#11381,#11382,#2086,.T.);
#13995=EDGE_CURVE('',#11382,#11383,#6400,.T.);
#13996=EDGE_CURVE('',#11383,#11384,#6401,.T.);
#13997=EDGE_CURVE('',#11384,#11357,#6402,.T.);
#13998=EDGE_CURVE('',#11385,#11325,#6403,.T.);
#13999=EDGE_CURVE('',#11325,#11384,#2087,.T.);
#14000=EDGE_CURVE('',#11383,#11385,#2088,.T.);
#14001=EDGE_CURVE('',#11385,#11386,#6404,.T.);
#14002=EDGE_CURVE('',#11386,#11324,#6405,.T.);
#14003=EDGE_CURVE('',#11387,#11388,#6406,.T.);
#14004=EDGE_CURVE('',#11388,#11324,#2089,.T.);
#14005=EDGE_CURVE('',#11386,#11387,#2090,.T.);
#14006=EDGE_CURVE('',#11387,#11380,#6407,.T.);
#14007=EDGE_CURVE('',#11379,#11388,#6408,.T.);
#14008=EDGE_CURVE('',#11388,#11295,#6409,.T.);
#14009=EDGE_CURVE('',#11295,#11389,#6410,.T.);
#14010=EDGE_CURVE('',#11389,#11390,#6411,.T.);
#14011=EDGE_CURVE('',#11326,#11390,#2091,.T.);
#14012=EDGE_CURVE('',#11296,#11379,#6412,.T.);
#14013=EDGE_CURVE('',#11378,#11391,#6413,.T.);
#14014=EDGE_CURVE('',#11392,#11391,#563,.T.);
#14015=EDGE_CURVE('',#11393,#11392,#564,.T.);
#14016=EDGE_CURVE('',#11394,#11393,#565,.T.);
#14017=EDGE_CURVE('',#11394,#11395,#6414,.T.);
#14018=EDGE_CURVE('',#11396,#11395,#566,.T.);
#14019=EDGE_CURVE('',#11397,#11396,#567,.T.);
#14020=EDGE_CURVE('',#11398,#11397,#568,.T.);
#14021=EDGE_CURVE('',#11398,#11399,#6415,.T.);
#14022=EDGE_CURVE('',#11400,#11399,#2092,.T.);
#14023=EDGE_CURVE('',#11400,#11306,#6416,.T.);
#14024=EDGE_CURVE('',#11401,#11402,#6417,.T.);
#14025=EDGE_CURVE('',#11403,#11401,#2093,.T.);
#14026=EDGE_CURVE('',#11404,#11403,#6418,.T.);
#14027=EDGE_CURVE('',#11405,#11404,#2094,.T.);
#14028=EDGE_CURVE('',#11406,#11405,#6419,.T.);
#14029=EDGE_CURVE('',#11407,#11406,#2095,.T.);
#14030=EDGE_CURVE('',#11408,#11407,#6420,.T.);
#14031=EDGE_CURVE('',#11402,#11408,#2096,.T.);
#14032=EDGE_CURVE('',#11409,#11400,#6421,.T.);
#14033=EDGE_CURVE('',#11399,#11410,#6422,.T.);
#14034=EDGE_CURVE('',#11410,#11409,#2097,.T.);
#14035=EDGE_CURVE('',#11409,#11411,#6423,.T.);
#14036=EDGE_CURVE('',#11411,#11390,#6424,.T.);
#14037=EDGE_CURVE('',#11390,#11400,#6425,.T.);
#14038=EDGE_CURVE('',#11412,#11326,#6426,.T.);
#14039=EDGE_CURVE('',#11411,#11412,#2098,.T.);
#14040=EDGE_CURVE('',#11412,#11413,#6427,.T.);
#14041=EDGE_CURVE('',#11413,#11327,#6428,.T.);
#14042=EDGE_CURVE('',#11414,#11415,#6429,.T.);
#14043=EDGE_CURVE('',#11415,#11327,#2099,.T.);
#14044=EDGE_CURVE('',#11413,#11414,#2100,.T.);
#14045=EDGE_CURVE('',#11414,#11416,#6430,.T.);
#14046=EDGE_CURVE('',#11416,#11358,#6431,.T.);
#14047=EDGE_CURVE('',#11358,#11415,#6432,.T.);
#14048=EDGE_CURVE('',#11417,#11359,#6433,.T.);
#14049=EDGE_CURVE('',#11416,#11417,#2101,.T.);
#14050=EDGE_CURVE('',#11417,#11410,#6434,.T.);
#14051=EDGE_CURVE('',#11399,#11359,#6435,.T.);
#14052=EDGE_CURVE('',#11415,#11384,#6436,.T.);
#14053=EDGE_CURVE('',#11360,#11363,#2102,.T.);
#14054=EDGE_CURVE('',#11395,#11398,#2103,.T.);
#14055=EDGE_CURVE('',#11391,#11394,#2104,.T.);
#14056=EDGE_CURVE('',#11418,#11419,#569,.T.);
#14057=EDGE_CURVE('',#11419,#11420,#570,.T.);
#14058=EDGE_CURVE('',#11420,#11421,#571,.T.);
#14059=EDGE_CURVE('',#11421,#11422,#572,.T.);
#14060=EDGE_CURVE('',#11422,#11423,#573,.T.);
#14061=EDGE_CURVE('',#11423,#11424,#574,.T.);
#14062=EDGE_CURVE('',#11424,#11425,#575,.T.);
#14063=EDGE_CURVE('',#11425,#11426,#576,.T.);
#14064=EDGE_CURVE('',#11426,#11427,#577,.T.);
#14065=EDGE_CURVE('',#11427,#11418,#578,.T.);
#14066=EDGE_CURVE('',#11428,#11429,#6437,.T.);
#14067=EDGE_CURVE('',#11429,#11430,#6438,.T.);
#14068=EDGE_CURVE('',#11430,#11431,#6439,.T.);
#14069=EDGE_CURVE('',#11431,#11432,#6440,.T.);
#14070=EDGE_CURVE('',#11432,#11433,#6441,.T.);
#14071=EDGE_CURVE('',#11433,#11434,#6442,.T.);
#14072=EDGE_CURVE('',#11434,#11435,#6443,.T.);
#14073=EDGE_CURVE('',#11435,#11428,#6444,.T.);
#14074=EDGE_CURVE('',#11436,#11437,#579,.T.);
#14075=EDGE_CURVE('',#11437,#11438,#580,.T.);
#14076=EDGE_CURVE('',#11438,#11439,#581,.T.);
#14077=EDGE_CURVE('',#11439,#11440,#582,.T.);
#14078=EDGE_CURVE('',#11440,#11441,#583,.T.);
#14079=EDGE_CURVE('',#11441,#11442,#584,.T.);
#14080=EDGE_CURVE('',#11442,#11443,#585,.T.);
#14081=EDGE_CURVE('',#11443,#11444,#586,.T.);
#14082=EDGE_CURVE('',#11444,#11445,#587,.T.);
#14083=EDGE_CURVE('',#11445,#11446,#588,.T.);
#14084=EDGE_CURVE('',#11446,#11447,#589,.T.);
#14085=EDGE_CURVE('',#11447,#11448,#590,.T.);
#14086=EDGE_CURVE('',#11448,#11436,#591,.T.);
#14087=EDGE_CURVE('',#11449,#11450,#6445,.T.);
#14088=EDGE_CURVE('',#11450,#11451,#6446,.T.);
#14089=EDGE_CURVE('',#11451,#11452,#6447,.T.);
#14090=EDGE_CURVE('',#11452,#11453,#592,.T.);
#14091=EDGE_CURVE('',#11453,#11454,#593,.T.);
#14092=EDGE_CURVE('',#11454,#11455,#594,.T.);
#14093=EDGE_CURVE('',#11455,#11456,#595,.T.);
#14094=EDGE_CURVE('',#11456,#11457,#596,.T.);
#14095=EDGE_CURVE('',#11457,#11458,#597,.T.);
#14096=EDGE_CURVE('',#11458,#11459,#598,.T.);
#14097=EDGE_CURVE('',#11459,#11460,#599,.T.);
#14098=EDGE_CURVE('',#11460,#11461,#6448,.T.);
#14099=EDGE_CURVE('',#11461,#11462,#600,.T.);
#14100=EDGE_CURVE('',#11462,#11463,#601,.T.);
#14101=EDGE_CURVE('',#11463,#11464,#602,.T.);
#14102=EDGE_CURVE('',#11464,#11465,#603,.T.);
#14103=EDGE_CURVE('',#11465,#11466,#604,.T.);
#14104=EDGE_CURVE('',#11466,#11467,#605,.T.);
#14105=EDGE_CURVE('',#11467,#11468,#606,.T.);
#14106=EDGE_CURVE('',#11468,#11469,#607,.T.);
#14107=EDGE_CURVE('',#11469,#11470,#608,.T.);
#14108=EDGE_CURVE('',#11470,#11449,#609,.T.);
#14109=EDGE_CURVE('',#11471,#11472,#6449,.T.);
#14110=EDGE_CURVE('',#11472,#11473,#6450,.T.);
#14111=EDGE_CURVE('',#11473,#11474,#6451,.T.);
#14112=EDGE_CURVE('',#11474,#11475,#6452,.T.);
#14113=EDGE_CURVE('',#11475,#11476,#6453,.T.);
#14114=EDGE_CURVE('',#11476,#11477,#6454,.T.);
#14115=EDGE_CURVE('',#11477,#11478,#6455,.T.);
#14116=EDGE_CURVE('',#11478,#11479,#6456,.T.);
#14117=EDGE_CURVE('',#11479,#11480,#6457,.T.);
#14118=EDGE_CURVE('',#11480,#11471,#6458,.T.);
#14119=EDGE_CURVE('',#11481,#11482,#6459,.T.);
#14120=EDGE_CURVE('',#11483,#11481,#2105,.T.);
#14121=EDGE_CURVE('',#11484,#11483,#6460,.T.);
#14122=EDGE_CURVE('',#11485,#11484,#2106,.T.);
#14123=EDGE_CURVE('',#11486,#11485,#6461,.T.);
#14124=EDGE_CURVE('',#11487,#11486,#2107,.T.);
#14125=EDGE_CURVE('',#11488,#11487,#6462,.T.);
#14126=EDGE_CURVE('',#11482,#11488,#2108,.T.);
#14127=EDGE_CURVE('',#11398,#11489,#6463,.T.);
#14128=EDGE_CURVE('',#11489,#11490,#2109,.T.);
#14129=EDGE_CURVE('',#11490,#11491,#2110,.T.);
#14130=EDGE_CURVE('',#11491,#11395,#6464,.T.);
#14131=EDGE_CURVE('',#11492,#11397,#6465,.T.);
#14132=EDGE_CURVE('',#11396,#11493,#6466,.T.);
#14133=EDGE_CURVE('',#11493,#11492,#610,.T.);
#14134=EDGE_CURVE('',#11491,#11493,#611,.T.);
#14135=EDGE_CURVE('',#11492,#11489,#612,.T.);
#14136=EDGE_CURVE('',#11490,#11494,#6467,.T.);
#14137=EDGE_CURVE('',#11495,#11494,#2111,.T.);
#14138=EDGE_CURVE('',#11496,#11495,#613,.T.);
#14139=EDGE_CURVE('',#11497,#11496,#614,.T.);
#14140=EDGE_CURVE('',#11498,#11497,#615,.T.);
#14141=EDGE_CURVE('',#11494,#11498,#2112,.T.);
#14142=EDGE_CURVE('',#11363,#11499,#6468,.T.);
#14143=EDGE_CURVE('',#11499,#11500,#2113,.T.);
#14144=EDGE_CURVE('',#11500,#11501,#2114,.T.);
#14145=EDGE_CURVE('',#11501,#11360,#6469,.T.);
#14146=EDGE_CURVE('',#11502,#11362,#6470,.T.);
#14147=EDGE_CURVE('',#11361,#11503,#6471,.T.);
#14148=EDGE_CURVE('',#11503,#11502,#616,.T.);
#14149=EDGE_CURVE('',#11501,#11503,#617,.T.);
#14150=EDGE_CURVE('',#11502,#11499,#618,.T.);
#14151=EDGE_CURVE('',#11500,#11504,#6472,.T.);
#14152=EDGE_CURVE('',#11505,#11504,#2115,.T.);
#14153=EDGE_CURVE('',#11506,#11505,#619,.T.);
#14154=EDGE_CURVE('',#11507,#11506,#620,.T.);
#14155=EDGE_CURVE('',#11508,#11507,#621,.T.);
#14156=EDGE_CURVE('',#11504,#11508,#2116,.T.);
#14157=EDGE_CURVE('',#11482,#11509,#6473,.T.);
#14158=EDGE_CURVE('',#11509,#11510,#6474,.T.);
#14159=EDGE_CURVE('',#11510,#11481,#6475,.T.);
#14160=EDGE_CURVE('',#11488,#11511,#6476,.T.);
#14161=EDGE_CURVE('',#11511,#11509,#2117,.T.);
#14162=EDGE_CURVE('',#11487,#11512,#6477,.T.);
#14163=EDGE_CURVE('',#11512,#11511,#6478,.T.);
#14164=EDGE_CURVE('',#11486,#11310,#6479,.T.);
#14165=EDGE_CURVE('',#11310,#11512,#2118,.T.);
#14166=EDGE_CURVE('',#11485,#11309,#6480,.T.);
#14167=EDGE_CURVE('',#11484,#11513,#6481,.T.);
#14168=EDGE_CURVE('',#11513,#11309,#2119,.T.);
#14169=EDGE_CURVE('',#11483,#11514,#6482,.T.);
#14170=EDGE_CURVE('',#11514,#11513,#6483,.T.);
#14171=EDGE_CURVE('',#11510,#11514,#2120,.T.);
#14172=EDGE_CURVE('',#11513,#11515,#6484,.T.);
#14173=EDGE_CURVE('',#11311,#11515,#2121,.T.);
#14174=EDGE_CURVE('',#11516,#11514,#6485,.T.);
#14175=EDGE_CURVE('',#11515,#11516,#6486,.T.);
#14176=EDGE_CURVE('',#11510,#11517,#6487,.T.);
#14177=EDGE_CURVE('',#11518,#11517,#622,.T.);
#14178=EDGE_CURVE('',#11519,#11518,#623,.T.);
#14179=EDGE_CURVE('',#11520,#11519,#624,.T.);
#14180=EDGE_CURVE('',#11521,#11520,#625,.T.);
#14181=EDGE_CURVE('',#11522,#11521,#626,.T.);
#14182=EDGE_CURVE('',#11523,#11522,#627,.T.);
#14183=EDGE_CURVE('',#11523,#11524,#6488,.T.);
#14184=EDGE_CURVE('',#11525,#11524,#628,.T.);
#14185=EDGE_CURVE('',#11526,#11525,#629,.T.);
#14186=EDGE_CURVE('',#11527,#11526,#630,.T.);
#14187=EDGE_CURVE('',#11528,#11527,#631,.T.);
#14188=EDGE_CURVE('',#11529,#11528,#632,.T.);
#14189=EDGE_CURVE('',#11530,#11529,#633,.T.);
#14190=EDGE_CURVE('',#11530,#11531,#6489,.T.);
#14191=EDGE_CURVE('',#11516,#11531,#2122,.T.);
#14192=EDGE_CURVE('',#11532,#11509,#6490,.T.);
#14193=EDGE_CURVE('',#11533,#11532,#2123,.T.);
#14194=EDGE_CURVE('',#11534,#11533,#6491,.T.);
#14195=EDGE_CURVE('',#11535,#11534,#2124,.T.);
#14196=EDGE_CURVE('',#11536,#11535,#6492,.T.);
#14197=EDGE_CURVE('',#11531,#11536,#6493,.T.);
#14198=EDGE_CURVE('',#11524,#11530,#2125,.T.);
#14199=EDGE_CURVE('',#11517,#11523,#2126,.T.);
#14200=EDGE_CURVE('',#11518,#11497,#6494,.T.);
#14201=EDGE_CURVE('',#11521,#11496,#6495,.T.);
#14202=EDGE_CURVE('',#11523,#11495,#6496,.T.);
#14203=EDGE_CURVE('',#11498,#11517,#6497,.T.);
#14204=EDGE_CURVE('',#11536,#11401,#6498,.T.);
#14205=EDGE_CURVE('',#11402,#11531,#6499,.T.);
#14206=EDGE_CURVE('',#11536,#11537,#2127,.T.);
#14207=EDGE_CURVE('',#11537,#11403,#6500,.T.);
#14208=EDGE_CURVE('',#11538,#11404,#6501,.T.);
#14209=EDGE_CURVE('',#11537,#11538,#6502,.T.);
#14210=EDGE_CURVE('',#11538,#11312,#2128,.T.);
#14211=EDGE_CURVE('',#11312,#11405,#6503,.T.);
#14212=EDGE_CURVE('',#11311,#11406,#6504,.T.);
#14213=EDGE_CURVE('',#11515,#11407,#6505,.T.);
#14214=EDGE_CURVE('',#11516,#11408,#6506,.T.);
#14215=EDGE_CURVE('',#11538,#11512,#6507,.T.);
#14216=EDGE_CURVE('',#11511,#11537,#6508,.T.);
#14217=EDGE_CURVE('',#11539,#11535,#634,.T.);
#14218=EDGE_CURVE('',#11540,#11539,#635,.T.);
#14219=EDGE_CURVE('',#11541,#11540,#636,.T.);
#14220=EDGE_CURVE('',#11542,#11541,#637,.T.);
#14221=EDGE_CURVE('',#11543,#11542,#638,.T.);
#14222=EDGE_CURVE('',#11534,#11543,#639,.T.);
#14223=EDGE_CURVE('',#11544,#11533,#640,.T.);
#14224=EDGE_CURVE('',#11545,#11544,#641,.T.);
#14225=EDGE_CURVE('',#11546,#11545,#642,.T.);
#14226=EDGE_CURVE('',#11547,#11546,#643,.T.);
#14227=EDGE_CURVE('',#11548,#11547,#644,.T.);
#14228=EDGE_CURVE('',#11532,#11548,#645,.T.);
#14229=EDGE_CURVE('',#11539,#11367,#6509,.T.);
#14230=EDGE_CURVE('',#11542,#11366,#6510,.T.);
#14231=EDGE_CURVE('',#11534,#11365,#6511,.T.);
#14232=EDGE_CURVE('',#11368,#11535,#6512,.T.);
#14233=EDGE_CURVE('',#11544,#11507,#6513,.T.);
#14234=EDGE_CURVE('',#11547,#11506,#6514,.T.);
#14235=EDGE_CURVE('',#11532,#11505,#6515,.T.);
#14236=EDGE_CURVE('',#11508,#11533,#6516,.T.);
#14237=EDGE_CURVE('',#11394,#11549,#6517,.T.);
#14238=EDGE_CURVE('',#11549,#11550,#2129,.T.);
#14239=EDGE_CURVE('',#11550,#11551,#2130,.T.);
#14240=EDGE_CURVE('',#11551,#11391,#6518,.T.);
#14241=EDGE_CURVE('',#11552,#11393,#6519,.T.);
#14242=EDGE_CURVE('',#11392,#11553,#6520,.T.);
#14243=EDGE_CURVE('',#11553,#11552,#646,.T.);
#14244=EDGE_CURVE('',#11551,#11553,#647,.T.);
#14245=EDGE_CURVE('',#11552,#11549,#648,.T.);
#14246=EDGE_CURVE('',#11550,#11554,#6521,.T.);
#14247=EDGE_CURVE('',#11555,#11554,#2131,.T.);
#14248=EDGE_CURVE('',#11556,#11555,#649,.T.);
#14249=EDGE_CURVE('',#11557,#11556,#650,.T.);
#14250=EDGE_CURVE('',#11558,#11557,#651,.T.);
#14251=EDGE_CURVE('',#11554,#11558,#2132,.T.);
#14252=EDGE_CURVE('',#11525,#11557,#6522,.T.);
#14253=EDGE_CURVE('',#11528,#11556,#6523,.T.);
#14254=EDGE_CURVE('',#11530,#11555,#6524,.T.);
#14255=EDGE_CURVE('',#11558,#11524,#6525,.T.);
#14256=EDGE_CURVE('',#11559,#11560,#6526,.T.);
#14257=EDGE_CURVE('',#11560,#11561,#2133,.T.);
#14258=EDGE_CURVE('',#11561,#11562,#6527,.T.);
#14259=EDGE_CURVE('',#11562,#11559,#2134,.T.);
#14260=EDGE_CURVE('',#11563,#11564,#6528,.T.);
#14261=EDGE_CURVE('',#11564,#11560,#6529,.T.);
#14262=EDGE_CURVE('',#11559,#11563,#6530,.T.);
#14263=EDGE_CURVE('',#11565,#11566,#6531,.T.);
#14264=EDGE_CURVE('',#11566,#11564,#2135,.T.);
#14265=EDGE_CURVE('',#11563,#11565,#2136,.T.);
#14266=EDGE_CURVE('',#11567,#11568,#6532,.T.);
#14267=EDGE_CURVE('',#11568,#11566,#6533,.T.);
#14268=EDGE_CURVE('',#11565,#11567,#6534,.T.);
#14269=EDGE_CURVE('',#11569,#11371,#6535,.T.);
#14270=EDGE_CURVE('',#11371,#11568,#2137,.T.);
#14271=EDGE_CURVE('',#11567,#11569,#2138,.T.);
#14272=EDGE_CURVE('',#11570,#11370,#6536,.T.);
#14273=EDGE_CURVE('',#11569,#11570,#6537,.T.);
#14274=EDGE_CURVE('',#11571,#11572,#6538,.T.);
#14275=EDGE_CURVE('',#11572,#11370,#2139,.T.);
#14276=EDGE_CURVE('',#11570,#11571,#2140,.T.);
#14277=EDGE_CURVE('',#11561,#11572,#6539,.T.);
#14278=EDGE_CURVE('',#11571,#11562,#6540,.T.);
#14279=EDGE_CURVE('',#11572,#11573,#6541,.T.);
#14280=EDGE_CURVE('',#11573,#11294,#6542,.T.);
#14281=EDGE_CURVE('',#11294,#11574,#6543,.T.);
#14282=EDGE_CURVE('',#11372,#11574,#2141,.T.);
#14283=EDGE_CURVE('',#11575,#11561,#6544,.T.);
#14284=EDGE_CURVE('',#11575,#11573,#6545,.T.);
#14285=EDGE_CURVE('',#11560,#11576,#6546,.T.);
#14286=EDGE_CURVE('',#11577,#11576,#652,.T.);
#14287=EDGE_CURVE('',#11578,#11577,#653,.T.);
#14288=EDGE_CURVE('',#11579,#11578,#654,.T.);
#14289=EDGE_CURVE('',#11579,#11580,#6547,.T.);
#14290=EDGE_CURVE('',#11581,#11580,#655,.T.);
#14291=EDGE_CURVE('',#11582,#11581,#656,.T.);
#14292=EDGE_CURVE('',#11583,#11582,#657,.T.);
#14293=EDGE_CURVE('',#11583,#11584,#6548,.T.);
#14294=EDGE_CURVE('',#11585,#11584,#2142,.T.);
#14295=EDGE_CURVE('',#11585,#11293,#6549,.T.);
#14296=EDGE_CURVE('',#11293,#11575,#6550,.T.);
#14297=EDGE_CURVE('',#11586,#11587,#6551,.T.);
#14298=EDGE_CURVE('',#11588,#11586,#2143,.T.);
#14299=EDGE_CURVE('',#11589,#11588,#6552,.T.);
#14300=EDGE_CURVE('',#11590,#11589,#2144,.T.);
#14301=EDGE_CURVE('',#11591,#11590,#6553,.T.);
#14302=EDGE_CURVE('',#11592,#11591,#2145,.T.);
#14303=EDGE_CURVE('',#11593,#11592,#6554,.T.);
#14304=EDGE_CURVE('',#11587,#11593,#2146,.T.);
#14305=EDGE_CURVE('',#11594,#11585,#6555,.T.);
#14306=EDGE_CURVE('',#11584,#11595,#6556,.T.);
#14307=EDGE_CURVE('',#11595,#11594,#2147,.T.);
#14308=EDGE_CURVE('',#11594,#11596,#6557,.T.);
#14309=EDGE_CURVE('',#11596,#11574,#6558,.T.);
#14310=EDGE_CURVE('',#11574,#11585,#6559,.T.);
#14311=EDGE_CURVE('',#11597,#11372,#6560,.T.);
#14312=EDGE_CURVE('',#11596,#11597,#2148,.T.);
#14313=EDGE_CURVE('',#11597,#11598,#6561,.T.);
#14314=EDGE_CURVE('',#11598,#11373,#6562,.T.);
#14315=EDGE_CURVE('',#11599,#11600,#6563,.T.);
#14316=EDGE_CURVE('',#11600,#11373,#2149,.T.);
#14317=EDGE_CURVE('',#11598,#11599,#2150,.T.);
#14318=EDGE_CURVE('',#11599,#11601,#6564,.T.);
#14319=EDGE_CURVE('',#11601,#11602,#6565,.T.);
#14320=EDGE_CURVE('',#11602,#11600,#6566,.T.);
#14321=EDGE_CURVE('',#11603,#11604,#6567,.T.);
#14322=EDGE_CURVE('',#11604,#11602,#2151,.T.);
#14323=EDGE_CURVE('',#11601,#11603,#2152,.T.);
#14324=EDGE_CURVE('',#11603,#11595,#6568,.T.);
#14325=EDGE_CURVE('',#11584,#11604,#6569,.T.);
#14326=EDGE_CURVE('',#11600,#11568,#6570,.T.);
#14327=EDGE_CURVE('',#11566,#11602,#6571,.T.);
#14328=EDGE_CURVE('',#11604,#11605,#6572,.T.);
#14329=EDGE_CURVE('',#11606,#11605,#658,.T.);
#14330=EDGE_CURVE('',#11607,#11606,#659,.T.);
#14331=EDGE_CURVE('',#11608,#11607,#660,.T.);
#14332=EDGE_CURVE('',#11608,#11609,#6573,.T.);
#14333=EDGE_CURVE('',#11610,#11609,#661,.T.);
#14334=EDGE_CURVE('',#11611,#11610,#662,.T.);
#14335=EDGE_CURVE('',#11612,#11611,#663,.T.);
#14336=EDGE_CURVE('',#11612,#11564,#6574,.T.);
#14337=EDGE_CURVE('',#11609,#11612,#2153,.T.);
#14338=EDGE_CURVE('',#11605,#11608,#2154,.T.);
#14339=EDGE_CURVE('',#11580,#11583,#2155,.T.);
#14340=EDGE_CURVE('',#11576,#11579,#2156,.T.);
#14341=EDGE_CURVE('',#11613,#11614,#6575,.T.);
#14342=EDGE_CURVE('',#11615,#11613,#2157,.T.);
#14343=EDGE_CURVE('',#11616,#11615,#6576,.T.);
#14344=EDGE_CURVE('',#11617,#11616,#2158,.T.);
#14345=EDGE_CURVE('',#11618,#11617,#6577,.T.);
#14346=EDGE_CURVE('',#11619,#11618,#2159,.T.);
#14347=EDGE_CURVE('',#11620,#11619,#6578,.T.);
#14348=EDGE_CURVE('',#11614,#11620,#2160,.T.);
#14349=EDGE_CURVE('',#11621,#11607,#6579,.T.);
#14350=EDGE_CURVE('',#11606,#11622,#6580,.T.);
#14351=EDGE_CURVE('',#11622,#11621,#664,.T.);
#14352=EDGE_CURVE('',#11608,#11623,#6581,.T.);
#14353=EDGE_CURVE('',#11623,#11624,#2161,.T.);
#14354=EDGE_CURVE('',#11624,#11625,#2162,.T.);
#14355=EDGE_CURVE('',#11625,#11605,#6582,.T.);
#14356=EDGE_CURVE('',#11621,#11623,#665,.T.);
#14357=EDGE_CURVE('',#11625,#11622,#666,.T.);
#14358=EDGE_CURVE('',#11624,#11626,#6583,.T.);
#14359=EDGE_CURVE('',#11627,#11626,#2163,.T.);
#14360=EDGE_CURVE('',#11628,#11627,#667,.T.);
#14361=EDGE_CURVE('',#11629,#11628,#668,.T.);
#14362=EDGE_CURVE('',#11630,#11629,#669,.T.);
#14363=EDGE_CURVE('',#11626,#11630,#2164,.T.);
#14364=EDGE_CURVE('',#11631,#11613,#6584,.T.);
#14365=EDGE_CURVE('',#11614,#11632,#6585,.T.);
#14366=EDGE_CURVE('',#11632,#11631,#6586,.T.);
#14367=EDGE_CURVE('',#11631,#11633,#2165,.T.);
#14368=EDGE_CURVE('',#11633,#11615,#6587,.T.);
#14369=EDGE_CURVE('',#11634,#11616,#6588,.T.);
#14370=EDGE_CURVE('',#11633,#11634,#6589,.T.);
#14371=EDGE_CURVE('',#11634,#11333,#2166,.T.);
#14372=EDGE_CURVE('',#11333,#11617,#6590,.T.);
#14373=EDGE_CURVE('',#11334,#11618,#6591,.T.);
#14374=EDGE_CURVE('',#11334,#11635,#2167,.T.);
#14375=EDGE_CURVE('',#11635,#11619,#6592,.T.);
#14376=EDGE_CURVE('',#11636,#11620,#6593,.T.);
#14377=EDGE_CURVE('',#11635,#11636,#6594,.T.);
#14378=EDGE_CURVE('',#11636,#11632,#2168,.T.);
#14379=EDGE_CURVE('',#11634,#11637,#6595,.T.);
#14380=EDGE_CURVE('',#11335,#11637,#2169,.T.);
#14381=EDGE_CURVE('',#11638,#11633,#6596,.T.);
#14382=EDGE_CURVE('',#11637,#11638,#6597,.T.);
#14383=EDGE_CURVE('',#11631,#11639,#6598,.T.);
#14384=EDGE_CURVE('',#11640,#11639,#670,.T.);
#14385=EDGE_CURVE('',#11641,#11640,#671,.T.);
#14386=EDGE_CURVE('',#11642,#11641,#672,.T.);
#14387=EDGE_CURVE('',#11643,#11642,#673,.T.);
#14388=EDGE_CURVE('',#11644,#11643,#674,.T.);
#14389=EDGE_CURVE('',#11644,#11645,#6599,.T.);
#14390=EDGE_CURVE('',#11646,#11645,#675,.T.);
#14391=EDGE_CURVE('',#11647,#11646,#676,.T.);
#14392=EDGE_CURVE('',#11648,#11647,#677,.T.);
#14393=EDGE_CURVE('',#11649,#11648,#678,.T.);
#14394=EDGE_CURVE('',#11650,#11649,#679,.T.);
#14395=EDGE_CURVE('',#11651,#11650,#680,.T.);
#14396=EDGE_CURVE('',#11651,#11652,#6600,.T.);
#14397=EDGE_CURVE('',#11638,#11652,#2170,.T.);
#14398=EDGE_CURVE('',#11653,#11632,#6601,.T.);
#14399=EDGE_CURVE('',#11654,#11653,#2171,.T.);
#14400=EDGE_CURVE('',#11655,#11654,#6602,.T.);
#14401=EDGE_CURVE('',#11656,#11655,#2172,.T.);
#14402=EDGE_CURVE('',#11657,#11656,#6603,.T.);
#14403=EDGE_CURVE('',#11652,#11657,#6604,.T.);
#14404=EDGE_CURVE('',#11645,#11651,#2173,.T.);
#14405=EDGE_CURVE('',#11639,#11644,#2174,.T.);
#14406=EDGE_CURVE('',#11587,#11652,#6605,.T.);
#14407=EDGE_CURVE('',#11657,#11586,#6606,.T.);
#14408=EDGE_CURVE('',#11593,#11638,#6607,.T.);
#14409=EDGE_CURVE('',#11592,#11637,#6608,.T.);
#14410=EDGE_CURVE('',#11591,#11335,#6609,.T.);
#14411=EDGE_CURVE('',#11590,#11336,#6610,.T.);
#14412=EDGE_CURVE('',#11589,#11658,#6611,.T.);
#14413=EDGE_CURVE('',#11658,#11336,#2175,.T.);
#14414=EDGE_CURVE('',#11588,#11659,#6612,.T.);
#14415=EDGE_CURVE('',#11659,#11658,#6613,.T.);
#14416=EDGE_CURVE('',#11657,#11659,#2176,.T.);
#14417=EDGE_CURVE('',#11658,#11635,#6614,.T.);
#14418=EDGE_CURVE('',#11636,#11659,#6615,.T.);
#14419=EDGE_CURVE('',#11660,#11656,#681,.T.);
#14420=EDGE_CURVE('',#11661,#11660,#682,.T.);
#14421=EDGE_CURVE('',#11662,#11661,#683,.T.);
#14422=EDGE_CURVE('',#11663,#11662,#684,.T.);
#14423=EDGE_CURVE('',#11655,#11663,#685,.T.);
#14424=EDGE_CURVE('',#11664,#11654,#686,.T.);
#14425=EDGE_CURVE('',#11665,#11664,#687,.T.);
#14426=EDGE_CURVE('',#11666,#11665,#688,.T.);
#14427=EDGE_CURVE('',#11667,#11666,#689,.T.);
#14428=EDGE_CURVE('',#11668,#11667,#690,.T.);
#14429=EDGE_CURVE('',#11653,#11668,#691,.T.);
#14430=EDGE_CURVE('',#11664,#11629,#6616,.T.);
#14431=EDGE_CURVE('',#11667,#11628,#6617,.T.);
#14432=EDGE_CURVE('',#11653,#11627,#6618,.T.);
#14433=EDGE_CURVE('',#11630,#11654,#6619,.T.);
#14434=EDGE_CURVE('',#11579,#11669,#6620,.T.);
#14435=EDGE_CURVE('',#11669,#11670,#2177,.T.);
#14436=EDGE_CURVE('',#11670,#11671,#2178,.T.);
#14437=EDGE_CURVE('',#11671,#11576,#6621,.T.);
#14438=EDGE_CURVE('',#11672,#11578,#6622,.T.);
#14439=EDGE_CURVE('',#11577,#11673,#6623,.T.);
#14440=EDGE_CURVE('',#11673,#11672,#692,.T.);
#14441=EDGE_CURVE('',#11671,#11673,#693,.T.);
#14442=EDGE_CURVE('',#11672,#11669,#694,.T.);
#14443=EDGE_CURVE('',#11670,#11674,#6624,.T.);
#14444=EDGE_CURVE('',#11675,#11674,#2179,.T.);
#14445=EDGE_CURVE('',#11676,#11675,#695,.T.);
#14446=EDGE_CURVE('',#11677,#11676,#696,.T.);
#14447=EDGE_CURVE('',#11678,#11677,#697,.T.);
#14448=EDGE_CURVE('',#11674,#11678,#2180,.T.);
#14449=EDGE_CURVE('',#11646,#11677,#6625,.T.);
#14450=EDGE_CURVE('',#11649,#11676,#6626,.T.);
#14451=EDGE_CURVE('',#11651,#11675,#6627,.T.);
#14452=EDGE_CURVE('',#11678,#11645,#6628,.T.);
#14453=EDGE_CURVE('',#11679,#11611,#6629,.T.);
#14454=EDGE_CURVE('',#11610,#11680,#6630,.T.);
#14455=EDGE_CURVE('',#11680,#11679,#698,.T.);
#14456=EDGE_CURVE('',#11612,#11681,#6631,.T.);
#14457=EDGE_CURVE('',#11681,#11682,#2181,.T.);
#14458=EDGE_CURVE('',#11682,#11683,#2182,.T.);
#14459=EDGE_CURVE('',#11683,#11609,#6632,.T.);
#14460=EDGE_CURVE('',#11679,#11681,#699,.T.);
#14461=EDGE_CURVE('',#11683,#11680,#700,.T.);
#14462=EDGE_CURVE('',#11682,#11684,#6633,.T.);
#14463=EDGE_CURVE('',#11685,#11684,#2183,.T.);
#14464=EDGE_CURVE('',#11686,#11685,#701,.T.);
#14465=EDGE_CURVE('',#11687,#11686,#702,.T.);
#14466=EDGE_CURVE('',#11688,#11687,#703,.T.);
#14467=EDGE_CURVE('',#11684,#11688,#2184,.T.);
#14468=EDGE_CURVE('',#11660,#11687,#6634,.T.);
#14469=EDGE_CURVE('',#11663,#11686,#6635,.T.);
#14470=EDGE_CURVE('',#11655,#11685,#6636,.T.);
#14471=EDGE_CURVE('',#11688,#11656,#6637,.T.);
#14472=EDGE_CURVE('',#11583,#11689,#6638,.T.);
#14473=EDGE_CURVE('',#11689,#11690,#2185,.T.);
#14474=EDGE_CURVE('',#11690,#11691,#2186,.T.);
#14475=EDGE_CURVE('',#11691,#11580,#6639,.T.);
#14476=EDGE_CURVE('',#11692,#11582,#6640,.T.);
#14477=EDGE_CURVE('',#11581,#11693,#6641,.T.);
#14478=EDGE_CURVE('',#11693,#11692,#704,.T.);
#14479=EDGE_CURVE('',#11691,#11693,#705,.T.);
#14480=EDGE_CURVE('',#11692,#11689,#706,.T.);
#14481=EDGE_CURVE('',#11690,#11694,#6642,.T.);
#14482=EDGE_CURVE('',#11695,#11694,#2187,.T.);
#14483=EDGE_CURVE('',#11696,#11695,#707,.T.);
#14484=EDGE_CURVE('',#11697,#11696,#708,.T.);
#14485=EDGE_CURVE('',#11698,#11697,#709,.T.);
#14486=EDGE_CURVE('',#11694,#11698,#2188,.T.);
#14487=EDGE_CURVE('',#11640,#11697,#6643,.T.);
#14488=EDGE_CURVE('',#11643,#11696,#6644,.T.);
#14489=EDGE_CURVE('',#11644,#11695,#6645,.T.);
#14490=EDGE_CURVE('',#11698,#11639,#6646,.T.);
#14491=EDGE_CURVE('',#11699,#11699,#2189,.T.);
#14492=EDGE_CURVE('',#11699,#11700,#6647,.T.);
#14493=EDGE_CURVE('',#11700,#11700,#2190,.T.);
#14494=EDGE_CURVE('',#11700,#11701,#6648,.T.);
#14495=EDGE_CURVE('',#11701,#11701,#2191,.T.);
#14496=EDGE_CURVE('',#11702,#11702,#2192,.T.);
#14497=EDGE_CURVE('',#11703,#11703,#2193,.T.);
#14498=EDGE_CURVE('',#11703,#11701,#6649,.T.);
#14499=EDGE_CURVE('',#11573,#11389,#6650,.T.);
#14500=EDGE_CURVE('',#11704,#11704,#2194,.T.);
#14501=EDGE_CURVE('',#11702,#11705,#6651,.T.);
#14502=EDGE_CURVE('',#11705,#11705,#2195,.T.);
#14503=EDGE_CURVE('',#11705,#11706,#6652,.T.);
#14504=EDGE_CURVE('',#11706,#11706,#2196,.T.);
#14505=EDGE_CURVE('',#11704,#11706,#6653,.T.);
#14506=EDGE_CURVE('',#11707,#11708,#710,.T.);
#14507=EDGE_CURVE('',#11707,#11709,#6654,.T.);
#14508=EDGE_CURVE('',#11709,#11710,#711,.T.);
#14509=EDGE_CURVE('',#11708,#11710,#6655,.T.);
#14510=EDGE_CURVE('',#11711,#11707,#712,.T.);
#14511=EDGE_CURVE('',#11711,#11712,#6656,.T.);
#14512=EDGE_CURVE('',#11712,#11709,#713,.T.);
#14513=EDGE_CURVE('',#11713,#11711,#714,.T.);
#14514=EDGE_CURVE('',#11713,#11714,#6657,.T.);
#14515=EDGE_CURVE('',#11714,#11712,#715,.T.);
#14516=EDGE_CURVE('',#11715,#11713,#716,.T.);
#14517=EDGE_CURVE('',#11715,#11716,#6658,.T.);
#14518=EDGE_CURVE('',#11716,#11714,#717,.T.);
#14519=EDGE_CURVE('',#11717,#11715,#718,.T.);
#14520=EDGE_CURVE('',#11717,#11718,#6659,.T.);
#14521=EDGE_CURVE('',#11718,#11716,#719,.T.);
#14522=EDGE_CURVE('',#11719,#11717,#720,.T.);
#14523=EDGE_CURVE('',#11719,#11720,#6660,.T.);
#14524=EDGE_CURVE('',#11720,#11718,#721,.T.);
#14525=EDGE_CURVE('',#11721,#11719,#722,.T.);
#14526=EDGE_CURVE('',#11721,#11722,#6661,.T.);
#14527=EDGE_CURVE('',#11722,#11720,#723,.T.);
#14528=EDGE_CURVE('',#11708,#11721,#724,.T.);
#14529=EDGE_CURVE('',#11710,#11722,#725,.T.);
#14530=EDGE_CURVE('',#11418,#11723,#6662,.T.);
#14531=EDGE_CURVE('',#11723,#11724,#726,.T.);
#14532=EDGE_CURVE('',#11419,#11724,#6663,.T.);
#14533=EDGE_CURVE('',#11427,#11725,#6664,.T.);
#14534=EDGE_CURVE('',#11725,#11723,#727,.T.);
#14535=EDGE_CURVE('',#11426,#11726,#6665,.T.);
#14536=EDGE_CURVE('',#11726,#11725,#728,.T.);
#14537=EDGE_CURVE('',#11425,#11727,#6666,.T.);
#14538=EDGE_CURVE('',#11727,#11726,#729,.T.);
#14539=EDGE_CURVE('',#11424,#11728,#6667,.T.);
#14540=EDGE_CURVE('',#11728,#11727,#730,.T.);
#14541=EDGE_CURVE('',#11423,#11729,#6668,.T.);
#14542=EDGE_CURVE('',#11729,#11728,#731,.T.);
#14543=EDGE_CURVE('',#11422,#11730,#6669,.T.);
#14544=EDGE_CURVE('',#11730,#11729,#732,.T.);
#14545=EDGE_CURVE('',#11421,#11731,#6670,.T.);
#14546=EDGE_CURVE('',#11731,#11730,#733,.T.);
#14547=EDGE_CURVE('',#11420,#11732,#6671,.T.);
#14548=EDGE_CURVE('',#11732,#11731,#734,.T.);
#14549=EDGE_CURVE('',#11724,#11732,#735,.T.);
#14550=EDGE_CURVE('',#11428,#11733,#6672,.T.);
#14551=EDGE_CURVE('',#11733,#11734,#6673,.T.);
#14552=EDGE_CURVE('',#11429,#11734,#6674,.T.);
#14553=EDGE_CURVE('',#11435,#11735,#6675,.T.);
#14554=EDGE_CURVE('',#11735,#11733,#6676,.T.);
#14555=EDGE_CURVE('',#11434,#11736,#6677,.T.);
#14556=EDGE_CURVE('',#11736,#11735,#6678,.T.);
#14557=EDGE_CURVE('',#11433,#11737,#6679,.T.);
#14558=EDGE_CURVE('',#11737,#11736,#6680,.T.);
#14559=EDGE_CURVE('',#11432,#11738,#6681,.T.);
#14560=EDGE_CURVE('',#11738,#11737,#6682,.T.);
#14561=EDGE_CURVE('',#11431,#11739,#6683,.T.);
#14562=EDGE_CURVE('',#11739,#11738,#6684,.T.);
#14563=EDGE_CURVE('',#11430,#11740,#6685,.T.);
#14564=EDGE_CURVE('',#11740,#11739,#6686,.T.);
#14565=EDGE_CURVE('',#11734,#11740,#6687,.T.);
#14566=EDGE_CURVE('',#11741,#11742,#736,.T.);
#14567=EDGE_CURVE('',#11741,#11743,#6688,.T.);
#14568=EDGE_CURVE('',#11743,#11744,#737,.T.);
#14569=EDGE_CURVE('',#11742,#11744,#6689,.T.);
#14570=EDGE_CURVE('',#11745,#11741,#738,.T.);
#14571=EDGE_CURVE('',#11745,#11746,#6690,.T.);
#14572=EDGE_CURVE('',#11746,#11743,#739,.T.);
#14573=EDGE_CURVE('',#11747,#11745,#740,.T.);
#14574=EDGE_CURVE('',#11747,#11748,#6691,.T.);
#14575=EDGE_CURVE('',#11748,#11746,#741,.T.);
#14576=EDGE_CURVE('',#11749,#11747,#742,.T.);
#14577=EDGE_CURVE('',#11749,#11750,#6692,.T.);
#14578=EDGE_CURVE('',#11750,#11748,#743,.T.);
#14579=EDGE_CURVE('',#11751,#11749,#744,.T.);
#14580=EDGE_CURVE('',#11751,#11752,#6693,.T.);
#14581=EDGE_CURVE('',#11752,#11750,#745,.T.);
#14582=EDGE_CURVE('',#11753,#11751,#746,.T.);
#14583=EDGE_CURVE('',#11753,#11754,#6694,.T.);
#14584=EDGE_CURVE('',#11754,#11752,#747,.T.);
#14585=EDGE_CURVE('',#11755,#11753,#748,.T.);
#14586=EDGE_CURVE('',#11755,#11756,#6695,.T.);
#14587=EDGE_CURVE('',#11756,#11754,#749,.T.);
#14588=EDGE_CURVE('',#11757,#11755,#750,.T.);
#14589=EDGE_CURVE('',#11757,#11758,#6696,.T.);
#14590=EDGE_CURVE('',#11758,#11756,#751,.T.);
#14591=EDGE_CURVE('',#11742,#11757,#752,.T.);
#14592=EDGE_CURVE('',#11744,#11758,#753,.T.);
#14593=EDGE_CURVE('',#11436,#11759,#6697,.T.);
#14594=EDGE_CURVE('',#11759,#11760,#754,.T.);
#14595=EDGE_CURVE('',#11437,#11760,#6698,.T.);
#14596=EDGE_CURVE('',#11448,#11761,#6699,.T.);
#14597=EDGE_CURVE('',#11761,#11759,#755,.T.);
#14598=EDGE_CURVE('',#11447,#11762,#6700,.T.);
#14599=EDGE_CURVE('',#11762,#11761,#756,.T.);
#14600=EDGE_CURVE('',#11446,#11763,#6701,.T.);
#14601=EDGE_CURVE('',#11763,#11762,#757,.T.);
#14602=EDGE_CURVE('',#11445,#11764,#6702,.T.);
#14603=EDGE_CURVE('',#11764,#11763,#758,.T.);
#14604=EDGE_CURVE('',#11444,#11765,#6703,.T.);
#14605=EDGE_CURVE('',#11765,#11764,#759,.T.);
#14606=EDGE_CURVE('',#11443,#11766,#6704,.T.);
#14607=EDGE_CURVE('',#11766,#11765,#760,.T.);
#14608=EDGE_CURVE('',#11442,#11767,#6705,.T.);
#14609=EDGE_CURVE('',#11767,#11766,#761,.T.);
#14610=EDGE_CURVE('',#11441,#11768,#6706,.T.);
#14611=EDGE_CURVE('',#11768,#11767,#762,.T.);
#14612=EDGE_CURVE('',#11440,#11769,#6707,.T.);
#14613=EDGE_CURVE('',#11769,#11768,#763,.T.);
#14614=EDGE_CURVE('',#11439,#11770,#6708,.T.);
#14615=EDGE_CURVE('',#11770,#11769,#764,.T.);
#14616=EDGE_CURVE('',#11438,#11771,#6709,.T.);
#14617=EDGE_CURVE('',#11771,#11770,#765,.T.);
#14618=EDGE_CURVE('',#11760,#11771,#766,.T.);
#14619=EDGE_CURVE('',#11449,#11772,#6710,.T.);
#14620=EDGE_CURVE('',#11772,#11773,#6711,.T.);
#14621=EDGE_CURVE('',#11450,#11773,#6712,.T.);
#14622=EDGE_CURVE('',#11470,#11774,#6713,.T.);
#14623=EDGE_CURVE('',#11774,#11772,#767,.T.);
#14624=EDGE_CURVE('',#11469,#11775,#6714,.T.);
#14625=EDGE_CURVE('',#11775,#11774,#768,.T.);
#14626=EDGE_CURVE('',#11468,#11776,#6715,.T.);
#14627=EDGE_CURVE('',#11776,#11775,#769,.T.);
#14628=EDGE_CURVE('',#11467,#11777,#6716,.T.);
#14629=EDGE_CURVE('',#11777,#11776,#770,.T.);
#14630=EDGE_CURVE('',#11466,#11778,#6717,.T.);
#14631=EDGE_CURVE('',#11778,#11777,#771,.T.);
#14632=EDGE_CURVE('',#11465,#11779,#6718,.T.);
#14633=EDGE_CURVE('',#11779,#11778,#772,.T.);
#14634=EDGE_CURVE('',#11464,#11780,#6719,.T.);
#14635=EDGE_CURVE('',#11780,#11779,#773,.T.);
#14636=EDGE_CURVE('',#11463,#11781,#6720,.T.);
#14637=EDGE_CURVE('',#11781,#11780,#774,.T.);
#14638=EDGE_CURVE('',#11462,#11782,#6721,.T.);
#14639=EDGE_CURVE('',#11782,#11781,#775,.T.);
#14640=EDGE_CURVE('',#11461,#11783,#6722,.T.);
#14641=EDGE_CURVE('',#11783,#11782,#776,.T.);
#14642=EDGE_CURVE('',#11460,#11784,#6723,.T.);
#14643=EDGE_CURVE('',#11784,#11783,#6724,.T.);
#14644=EDGE_CURVE('',#11459,#11785,#6725,.T.);
#14645=EDGE_CURVE('',#11785,#11784,#777,.T.);
#14646=EDGE_CURVE('',#11458,#11786,#6726,.T.);
#14647=EDGE_CURVE('',#11786,#11785,#778,.T.);
#14648=EDGE_CURVE('',#11457,#11787,#6727,.T.);
#14649=EDGE_CURVE('',#11787,#11786,#779,.T.);
#14650=EDGE_CURVE('',#11456,#11788,#6728,.T.);
#14651=EDGE_CURVE('',#11788,#11787,#780,.T.);
#14652=EDGE_CURVE('',#11455,#11789,#6729,.T.);
#14653=EDGE_CURVE('',#11789,#11788,#781,.T.);
#14654=EDGE_CURVE('',#11454,#11790,#6730,.T.);
#14655=EDGE_CURVE('',#11790,#11789,#782,.T.);
#14656=EDGE_CURVE('',#11453,#11791,#6731,.T.);
#14657=EDGE_CURVE('',#11791,#11790,#783,.T.);
#14658=EDGE_CURVE('',#11452,#11792,#6732,.T.);
#14659=EDGE_CURVE('',#11792,#11791,#784,.T.);
#14660=EDGE_CURVE('',#11451,#11793,#6733,.T.);
#14661=EDGE_CURVE('',#11793,#11792,#6734,.T.);
#14662=EDGE_CURVE('',#11773,#11793,#6735,.T.);
#14663=EDGE_CURVE('',#11471,#11794,#6736,.T.);
#14664=EDGE_CURVE('',#11794,#11795,#6737,.T.);
#14665=EDGE_CURVE('',#11472,#11795,#6738,.T.);
#14666=EDGE_CURVE('',#11480,#11796,#6739,.T.);
#14667=EDGE_CURVE('',#11796,#11794,#6740,.T.);
#14668=EDGE_CURVE('',#11479,#11797,#6741,.T.);
#14669=EDGE_CURVE('',#11797,#11796,#6742,.T.);
#14670=EDGE_CURVE('',#11478,#11798,#6743,.T.);
#14671=EDGE_CURVE('',#11798,#11797,#6744,.T.);
#14672=EDGE_CURVE('',#11477,#11799,#6745,.T.);
#14673=EDGE_CURVE('',#11799,#11798,#6746,.T.);
#14674=EDGE_CURVE('',#11476,#11800,#6747,.T.);
#14675=EDGE_CURVE('',#11800,#11799,#6748,.T.);
#14676=EDGE_CURVE('',#11475,#11801,#6749,.T.);
#14677=EDGE_CURVE('',#11801,#11800,#6750,.T.);
#14678=EDGE_CURVE('',#11474,#11802,#6751,.T.);
#14679=EDGE_CURVE('',#11802,#11801,#6752,.T.);
#14680=EDGE_CURVE('',#11473,#11803,#6753,.T.);
#14681=EDGE_CURVE('',#11803,#11802,#6754,.T.);
#14682=EDGE_CURVE('',#11795,#11803,#6755,.T.);
#14683=EDGE_CURVE('',#11278,#11575,#6756,.T.);
#14684=EDGE_CURVE('',#11389,#11306,#6757,.T.);
#17919=ORIENTED_EDGE('',*,*,#13843,.T.);
#17920=ORIENTED_EDGE('',*,*,#13844,.T.);
#17921=ORIENTED_EDGE('',*,*,#13845,.T.);
#17922=ORIENTED_EDGE('',*,*,#13846,.T.);
#17923=ORIENTED_EDGE('',*,*,#13847,.T.);
#17924=ORIENTED_EDGE('',*,*,#13845,.F.);
#17925=ORIENTED_EDGE('',*,*,#13848,.T.);
#17926=ORIENTED_EDGE('',*,*,#13849,.F.);
#17927=ORIENTED_EDGE('',*,*,#13850,.F.);
#17928=ORIENTED_EDGE('',*,*,#13851,.T.);
#17929=ORIENTED_EDGE('',*,*,#13852,.F.);
#17930=ORIENTED_EDGE('',*,*,#13844,.F.);
#17931=ORIENTED_EDGE('',*,*,#13853,.F.);
#17932=ORIENTED_EDGE('',*,*,#13854,.F.);
#17933=ORIENTED_EDGE('',*,*,#13848,.F.);
#17934=ORIENTED_EDGE('',*,*,#13843,.F.);
#17935=ORIENTED_EDGE('',*,*,#13855,.T.);
#17936=ORIENTED_EDGE('',*,*,#13856,.T.);
#17937=ORIENTED_EDGE('',*,*,#13853,.T.);
#17938=ORIENTED_EDGE('',*,*,#13856,.F.);
#17939=ORIENTED_EDGE('',*,*,#13857,.T.);
#17940=ORIENTED_EDGE('',*,*,#13858,.T.);
#17941=ORIENTED_EDGE('',*,*,#13849,.T.);
#17942=ORIENTED_EDGE('',*,*,#13854,.T.);
#17943=ORIENTED_EDGE('',*,*,#13858,.F.);
#17944=ORIENTED_EDGE('',*,*,#13859,.T.);
#17945=ORIENTED_EDGE('',*,*,#13860,.F.);
#17946=ORIENTED_EDGE('',*,*,#13861,.F.);
#17947=ORIENTED_EDGE('',*,*,#13862,.T.);
#17948=ORIENTED_EDGE('',*,*,#13850,.T.);
#17949=ORIENTED_EDGE('',*,*,#13857,.F.);
#17950=ORIENTED_EDGE('',*,*,#13863,.F.);
#17951=ORIENTED_EDGE('',*,*,#13864,.F.);
#17952=ORIENTED_EDGE('',*,*,#13865,.F.);
#17953=ORIENTED_EDGE('',*,*,#13866,.F.);
#17954=ORIENTED_EDGE('',*,*,#13867,.F.);
#17955=ORIENTED_EDGE('',*,*,#13868,.F.);
#17956=ORIENTED_EDGE('',*,*,#13859,.F.);
#17957=ORIENTED_EDGE('',*,*,#13869,.T.);
#17958=ORIENTED_EDGE('',*,*,#13870,.T.);
#17959=ORIENTED_EDGE('',*,*,#13871,.T.);
#17960=ORIENTED_EDGE('',*,*,#13872,.T.);
#17961=ORIENTED_EDGE('',*,*,#13873,.T.);
#17962=ORIENTED_EDGE('',*,*,#13873,.F.);
#17963=ORIENTED_EDGE('',*,*,#13874,.F.);
#17964=ORIENTED_EDGE('',*,*,#13875,.F.);
#17965=ORIENTED_EDGE('',*,*,#13876,.F.);
#17966=ORIENTED_EDGE('',*,*,#13872,.F.);
#17967=ORIENTED_EDGE('',*,*,#13877,.F.);
#17968=ORIENTED_EDGE('',*,*,#13878,.T.);
#17969=ORIENTED_EDGE('',*,*,#13861,.T.);
#17970=ORIENTED_EDGE('',*,*,#13879,.F.);
#17971=ORIENTED_EDGE('',*,*,#13874,.T.);
#17972=ORIENTED_EDGE('',*,*,#13846,.F.);
#17973=ORIENTED_EDGE('',*,*,#13852,.T.);
#17974=ORIENTED_EDGE('',*,*,#13880,.T.);
#17975=ORIENTED_EDGE('',*,*,#13877,.T.);
#17976=ORIENTED_EDGE('',*,*,#13871,.F.);
#17977=ORIENTED_EDGE('',*,*,#13881,.T.);
#17978=ORIENTED_EDGE('',*,*,#13869,.F.);
#17979=ORIENTED_EDGE('',*,*,#13876,.T.);
#17980=ORIENTED_EDGE('',*,*,#13882,.T.);
#17981=ORIENTED_EDGE('',*,*,#13883,.T.);
#17982=ORIENTED_EDGE('',*,*,#13883,.F.);
#17983=ORIENTED_EDGE('',*,*,#13867,.T.);
#17984=ORIENTED_EDGE('',*,*,#13884,.F.);
#17985=ORIENTED_EDGE('',*,*,#13885,.T.);
#17986=ORIENTED_EDGE('',*,*,#13882,.F.);
#17987=ORIENTED_EDGE('',*,*,#13875,.T.);
#17988=ORIENTED_EDGE('',*,*,#13879,.T.);
#17989=ORIENTED_EDGE('',*,*,#13860,.T.);
#17990=ORIENTED_EDGE('',*,*,#13868,.T.);
#17991=ORIENTED_EDGE('',*,*,#13886,.T.);
#17992=ORIENTED_EDGE('',*,*,#13887,.T.);
#17993=ORIENTED_EDGE('',*,*,#13888,.T.);
#17994=ORIENTED_EDGE('',*,*,#13887,.F.);
#17995=ORIENTED_EDGE('',*,*,#13889,.F.);
#17996=ORIENTED_EDGE('',*,*,#13890,.F.);
#17997=ORIENTED_EDGE('',*,*,#13891,.F.);
#17998=ORIENTED_EDGE('',*,*,#13892,.F.);
#17999=ORIENTED_EDGE('',*,*,#13893,.F.);
#18000=ORIENTED_EDGE('',*,*,#13894,.F.);
#18001=ORIENTED_EDGE('',*,*,#13895,.F.);
#18002=ORIENTED_EDGE('',*,*,#13886,.F.);
#18003=ORIENTED_EDGE('',*,*,#13888,.F.);
#18004=ORIENTED_EDGE('',*,*,#13896,.T.);
#18005=ORIENTED_EDGE('',*,*,#13897,.F.);
#18006=ORIENTED_EDGE('',*,*,#13896,.F.);
#18007=ORIENTED_EDGE('',*,*,#13893,.T.);
#18008=ORIENTED_EDGE('',*,*,#13898,.T.);
#18009=ORIENTED_EDGE('',*,*,#13899,.T.);
#18010=ORIENTED_EDGE('',*,*,#13898,.F.);
#18011=ORIENTED_EDGE('',*,*,#13899,.F.);
#18012=ORIENTED_EDGE('',*,*,#13900,.T.);
#18013=ORIENTED_EDGE('',*,*,#13901,.F.);
#18014=ORIENTED_EDGE('',*,*,#13900,.F.);
#18015=ORIENTED_EDGE('',*,*,#13895,.T.);
#18016=ORIENTED_EDGE('',*,*,#13902,.T.);
#18017=ORIENTED_EDGE('',*,*,#13903,.T.);
#18018=ORIENTED_EDGE('',*,*,#13902,.F.);
#18019=ORIENTED_EDGE('',*,*,#13903,.F.);
#18020=ORIENTED_EDGE('',*,*,#13904,.T.);
#18021=ORIENTED_EDGE('',*,*,#13905,.F.);
#18022=ORIENTED_EDGE('',*,*,#13904,.F.);
#18023=ORIENTED_EDGE('',*,*,#13894,.T.);
#18024=ORIENTED_EDGE('',*,*,#13906,.T.);
#18025=ORIENTED_EDGE('',*,*,#13907,.T.);
#18026=ORIENTED_EDGE('',*,*,#13906,.F.);
#18027=ORIENTED_EDGE('',*,*,#13907,.F.);
#18028=ORIENTED_EDGE('',*,*,#13908,.T.);
#18029=ORIENTED_EDGE('',*,*,#13909,.F.);
#18030=ORIENTED_EDGE('',*,*,#13908,.F.);
#18031=ORIENTED_EDGE('',*,*,#13910,.T.);
#18032=ORIENTED_EDGE('',*,*,#13911,.T.);
#18033=ORIENTED_EDGE('',*,*,#13909,.T.);
#18034=ORIENTED_EDGE('',*,*,#13911,.F.);
#18035=ORIENTED_EDGE('',*,*,#13912,.F.);
#18036=ORIENTED_EDGE('',*,*,#13913,.F.);
#18037=ORIENTED_EDGE('',*,*,#13914,.F.);
#18038=ORIENTED_EDGE('',*,*,#13915,.F.);
#18039=ORIENTED_EDGE('',*,*,#13916,.F.);
#18040=ORIENTED_EDGE('',*,*,#13917,.F.);
#18041=ORIENTED_EDGE('',*,*,#13918,.F.);
#18042=ORIENTED_EDGE('',*,*,#13910,.F.);
#18043=ORIENTED_EDGE('',*,*,#13916,.T.);
#18044=ORIENTED_EDGE('',*,*,#13919,.T.);
#18045=ORIENTED_EDGE('',*,*,#13905,.T.);
#18046=ORIENTED_EDGE('',*,*,#13919,.F.);
#18047=ORIENTED_EDGE('',*,*,#13918,.T.);
#18048=ORIENTED_EDGE('',*,*,#13920,.T.);
#18049=ORIENTED_EDGE('',*,*,#13901,.T.);
#18050=ORIENTED_EDGE('',*,*,#13920,.F.);
#18051=ORIENTED_EDGE('',*,*,#13917,.T.);
#18052=ORIENTED_EDGE('',*,*,#13921,.T.);
#18053=ORIENTED_EDGE('',*,*,#13897,.T.);
#18054=ORIENTED_EDGE('',*,*,#13921,.F.);
#18055=ORIENTED_EDGE('',*,*,#13922,.T.);
#18056=ORIENTED_EDGE('',*,*,#13923,.T.);
#18057=ORIENTED_EDGE('',*,*,#13924,.T.);
#18058=ORIENTED_EDGE('',*,*,#13923,.F.);
#18059=ORIENTED_EDGE('',*,*,#13925,.F.);
#18060=ORIENTED_EDGE('',*,*,#13926,.F.);
#18061=ORIENTED_EDGE('',*,*,#13927,.F.);
#18062=ORIENTED_EDGE('',*,*,#13928,.F.);
#18063=ORIENTED_EDGE('',*,*,#13929,.F.);
#18064=ORIENTED_EDGE('',*,*,#13930,.F.);
#18065=ORIENTED_EDGE('',*,*,#13931,.F.);
#18066=ORIENTED_EDGE('',*,*,#13922,.F.);
#18067=ORIENTED_EDGE('',*,*,#13932,.F.);
#18068=ORIENTED_EDGE('',*,*,#13933,.T.);
#18069=ORIENTED_EDGE('',*,*,#13924,.F.);
#18070=ORIENTED_EDGE('',*,*,#13933,.F.);
#18071=ORIENTED_EDGE('',*,*,#13929,.T.);
#18072=ORIENTED_EDGE('',*,*,#13934,.T.);
#18073=ORIENTED_EDGE('',*,*,#13935,.T.);
#18074=ORIENTED_EDGE('',*,*,#13934,.F.);
#18075=ORIENTED_EDGE('',*,*,#13936,.F.);
#18076=ORIENTED_EDGE('',*,*,#13937,.T.);
#18077=ORIENTED_EDGE('',*,*,#13935,.F.);
#18078=ORIENTED_EDGE('',*,*,#13937,.F.);
#18079=ORIENTED_EDGE('',*,*,#13931,.T.);
#18080=ORIENTED_EDGE('',*,*,#13938,.T.);
#18081=ORIENTED_EDGE('',*,*,#13939,.T.);
#18082=ORIENTED_EDGE('',*,*,#13938,.F.);
#18083=ORIENTED_EDGE('',*,*,#13940,.F.);
#18084=ORIENTED_EDGE('',*,*,#13941,.T.);
#18085=ORIENTED_EDGE('',*,*,#13939,.F.);
#18086=ORIENTED_EDGE('',*,*,#13941,.F.);
#18087=ORIENTED_EDGE('',*,*,#13930,.T.);
#18088=ORIENTED_EDGE('',*,*,#13942,.T.);
#18089=ORIENTED_EDGE('',*,*,#13943,.T.);
#18090=ORIENTED_EDGE('',*,*,#13942,.F.);
#18091=ORIENTED_EDGE('',*,*,#13944,.F.);
#18092=ORIENTED_EDGE('',*,*,#13945,.T.);
#18093=ORIENTED_EDGE('',*,*,#13943,.F.);
#18094=ORIENTED_EDGE('',*,*,#13945,.F.);
#18095=ORIENTED_EDGE('',*,*,#13946,.T.);
#18096=ORIENTED_EDGE('',*,*,#13947,.T.);
#18097=ORIENTED_EDGE('',*,*,#13948,.T.);
#18098=ORIENTED_EDGE('',*,*,#13949,.T.);
#18099=ORIENTED_EDGE('',*,*,#13950,.T.);
#18100=ORIENTED_EDGE('',*,*,#13951,.T.);
#18101=ORIENTED_EDGE('',*,*,#13952,.T.);
#18102=ORIENTED_EDGE('',*,*,#13953,.T.);
#18103=ORIENTED_EDGE('',*,*,#13954,.T.);
#18104=ORIENTED_EDGE('',*,*,#13953,.F.);
#18105=ORIENTED_EDGE('',*,*,#13955,.T.);
#18106=ORIENTED_EDGE('',*,*,#13949,.F.);
#18107=ORIENTED_EDGE('',*,*,#13956,.T.);
#18108=ORIENTED_EDGE('',*,*,#13946,.F.);
#18109=ORIENTED_EDGE('',*,*,#13957,.T.);
#18110=ORIENTED_EDGE('',*,*,#13951,.F.);
#18111=ORIENTED_EDGE('',*,*,#13958,.T.);
#18112=ORIENTED_EDGE('',*,*,#13955,.F.);
#18113=ORIENTED_EDGE('',*,*,#13952,.F.);
#18114=ORIENTED_EDGE('',*,*,#13957,.F.);
#18115=ORIENTED_EDGE('',*,*,#13959,.T.);
#18116=ORIENTED_EDGE('',*,*,#13960,.F.);
#18117=ORIENTED_EDGE('',*,*,#13961,.T.);
#18118=ORIENTED_EDGE('',*,*,#13962,.F.);
#18119=ORIENTED_EDGE('',*,*,#13963,.T.);
#18120=ORIENTED_EDGE('',*,*,#13964,.F.);
#18121=ORIENTED_EDGE('',*,*,#13965,.F.);
#18122=ORIENTED_EDGE('',*,*,#13966,.F.);
#18123=ORIENTED_EDGE('',*,*,#13967,.T.);
#18124=ORIENTED_EDGE('',*,*,#13954,.F.);
#18125=ORIENTED_EDGE('',*,*,#13956,.F.);
#18126=ORIENTED_EDGE('',*,*,#13948,.F.);
#18127=ORIENTED_EDGE('',*,*,#13968,.T.);
#18128=ORIENTED_EDGE('',*,*,#13969,.F.);
#18129=ORIENTED_EDGE('',*,*,#13970,.F.);
#18130=ORIENTED_EDGE('',*,*,#13971,.F.);
#18131=ORIENTED_EDGE('',*,*,#13972,.F.);
#18132=ORIENTED_EDGE('',*,*,#13973,.F.);
#18133=ORIENTED_EDGE('',*,*,#13968,.F.);
#18134=ORIENTED_EDGE('',*,*,#13947,.F.);
#18135=ORIENTED_EDGE('',*,*,#13958,.F.);
#18136=ORIENTED_EDGE('',*,*,#13974,.T.);
#18137=ORIENTED_EDGE('',*,*,#13975,.T.);
#18138=ORIENTED_EDGE('',*,*,#13944,.T.);
#18139=ORIENTED_EDGE('',*,*,#13975,.F.);
#18140=ORIENTED_EDGE('',*,*,#13976,.F.);
#18141=ORIENTED_EDGE('',*,*,#13977,.F.);
#18142=ORIENTED_EDGE('',*,*,#13978,.F.);
#18143=ORIENTED_EDGE('',*,*,#13979,.F.);
#18144=ORIENTED_EDGE('',*,*,#13980,.F.);
#18145=ORIENTED_EDGE('',*,*,#13981,.F.);
#18146=ORIENTED_EDGE('',*,*,#13982,.F.);
#18147=ORIENTED_EDGE('',*,*,#13974,.F.);
#18148=ORIENTED_EDGE('',*,*,#13980,.T.);
#18149=ORIENTED_EDGE('',*,*,#13983,.T.);
#18150=ORIENTED_EDGE('',*,*,#13940,.T.);
#18151=ORIENTED_EDGE('',*,*,#13983,.F.);
#18152=ORIENTED_EDGE('',*,*,#13982,.T.);
#18153=ORIENTED_EDGE('',*,*,#13984,.T.);
#18154=ORIENTED_EDGE('',*,*,#13936,.T.);
#18155=ORIENTED_EDGE('',*,*,#13984,.F.);
#18156=ORIENTED_EDGE('',*,*,#13981,.T.);
#18157=ORIENTED_EDGE('',*,*,#13985,.T.);
#18158=ORIENTED_EDGE('',*,*,#13932,.T.);
#18159=ORIENTED_EDGE('',*,*,#13985,.F.);
#18160=ORIENTED_EDGE('',*,*,#13986,.T.);
#18161=ORIENTED_EDGE('',*,*,#13987,.T.);
#18162=ORIENTED_EDGE('',*,*,#13988,.T.);
#18163=ORIENTED_EDGE('',*,*,#13989,.T.);
#18164=ORIENTED_EDGE('',*,*,#13986,.F.);
#18165=ORIENTED_EDGE('',*,*,#13990,.T.);
#18166=ORIENTED_EDGE('',*,*,#13991,.T.);
#18167=ORIENTED_EDGE('',*,*,#13992,.T.);
#18168=ORIENTED_EDGE('',*,*,#13993,.T.);
#18169=ORIENTED_EDGE('',*,*,#13960,.T.);
#18170=ORIENTED_EDGE('',*,*,#13991,.F.);
#18171=ORIENTED_EDGE('',*,*,#13994,.T.);
#18172=ORIENTED_EDGE('',*,*,#13993,.F.);
#18173=ORIENTED_EDGE('',*,*,#13995,.T.);
#18174=ORIENTED_EDGE('',*,*,#13996,.T.);
#18175=ORIENTED_EDGE('',*,*,#13997,.T.);
#18176=ORIENTED_EDGE('',*,*,#13998,.T.);
#18177=ORIENTED_EDGE('',*,*,#13999,.T.);
#18178=ORIENTED_EDGE('',*,*,#13996,.F.);
#18179=ORIENTED_EDGE('',*,*,#14000,.T.);
#18180=ORIENTED_EDGE('',*,*,#13998,.F.);
#18181=ORIENTED_EDGE('',*,*,#14001,.T.);
#18182=ORIENTED_EDGE('',*,*,#14002,.T.);
#18183=ORIENTED_EDGE('',*,*,#13912,.T.);
#18184=ORIENTED_EDGE('',*,*,#14003,.T.);
#18185=ORIENTED_EDGE('',*,*,#14004,.T.);
#18186=ORIENTED_EDGE('',*,*,#14002,.F.);
#18187=ORIENTED_EDGE('',*,*,#14005,.T.);
#18188=ORIENTED_EDGE('',*,*,#14003,.F.);
#18189=ORIENTED_EDGE('',*,*,#14006,.T.);
#18190=ORIENTED_EDGE('',*,*,#13988,.F.);
#18191=ORIENTED_EDGE('',*,*,#14007,.T.);
#18192=ORIENTED_EDGE('',*,*,#14004,.F.);
#18193=ORIENTED_EDGE('',*,*,#14008,.T.);
#18194=ORIENTED_EDGE('',*,*,#14009,.T.);
#18195=ORIENTED_EDGE('',*,*,#14010,.T.);
#18196=ORIENTED_EDGE('',*,*,#14011,.F.);
#18197=ORIENTED_EDGE('',*,*,#13913,.T.);
#18198=ORIENTED_EDGE('',*,*,#14007,.F.);
#18199=ORIENTED_EDGE('',*,*,#14012,.F.);
#18200=ORIENTED_EDGE('',*,*,#13866,.T.);
#18201=ORIENTED_EDGE('',*,*,#14008,.F.);
#18202=ORIENTED_EDGE('',*,*,#13987,.F.);
#18203=ORIENTED_EDGE('',*,*,#14013,.T.);
#18204=ORIENTED_EDGE('',*,*,#14014,.F.);
#18205=ORIENTED_EDGE('',*,*,#14015,.F.);
#18206=ORIENTED_EDGE('',*,*,#14016,.F.);
#18207=ORIENTED_EDGE('',*,*,#14017,.T.);
#18208=ORIENTED_EDGE('',*,*,#14018,.F.);
#18209=ORIENTED_EDGE('',*,*,#14019,.F.);
#18210=ORIENTED_EDGE('',*,*,#14020,.F.);
#18211=ORIENTED_EDGE('',*,*,#14021,.T.);
#18212=ORIENTED_EDGE('',*,*,#14022,.F.);
#18213=ORIENTED_EDGE('',*,*,#14023,.T.);
#18214=ORIENTED_EDGE('',*,*,#13884,.T.);
#18215=ORIENTED_EDGE('',*,*,#14012,.T.);
#18216=ORIENTED_EDGE('',*,*,#13989,.F.);
#18217=ORIENTED_EDGE('',*,*,#14006,.F.);
#18218=ORIENTED_EDGE('',*,*,#14005,.F.);
#18219=ORIENTED_EDGE('',*,*,#14001,.F.);
#18220=ORIENTED_EDGE('',*,*,#14000,.F.);
#18221=ORIENTED_EDGE('',*,*,#13995,.F.);
#18222=ORIENTED_EDGE('',*,*,#13994,.F.);
#18223=ORIENTED_EDGE('',*,*,#13990,.F.);
#18224=ORIENTED_EDGE('',*,*,#14024,.F.);
#18225=ORIENTED_EDGE('',*,*,#14025,.F.);
#18226=ORIENTED_EDGE('',*,*,#14026,.F.);
#18227=ORIENTED_EDGE('',*,*,#14027,.F.);
#18228=ORIENTED_EDGE('',*,*,#14028,.F.);
#18229=ORIENTED_EDGE('',*,*,#14029,.F.);
#18230=ORIENTED_EDGE('',*,*,#14030,.F.);
#18231=ORIENTED_EDGE('',*,*,#14031,.F.);
#18232=ORIENTED_EDGE('',*,*,#14032,.T.);
#18233=ORIENTED_EDGE('',*,*,#14022,.T.);
#18234=ORIENTED_EDGE('',*,*,#14033,.T.);
#18235=ORIENTED_EDGE('',*,*,#14034,.T.);
#18236=ORIENTED_EDGE('',*,*,#14032,.F.);
#18237=ORIENTED_EDGE('',*,*,#14035,.T.);
#18238=ORIENTED_EDGE('',*,*,#14036,.T.);
#18239=ORIENTED_EDGE('',*,*,#14037,.T.);
#18240=ORIENTED_EDGE('',*,*,#14038,.T.);
#18241=ORIENTED_EDGE('',*,*,#14011,.T.);
#18242=ORIENTED_EDGE('',*,*,#14036,.F.);
#18243=ORIENTED_EDGE('',*,*,#14039,.T.);
#18244=ORIENTED_EDGE('',*,*,#14038,.F.);
#18245=ORIENTED_EDGE('',*,*,#14040,.T.);
#18246=ORIENTED_EDGE('',*,*,#14041,.T.);
#18247=ORIENTED_EDGE('',*,*,#13914,.T.);
#18248=ORIENTED_EDGE('',*,*,#14042,.T.);
#18249=ORIENTED_EDGE('',*,*,#14043,.T.);
#18250=ORIENTED_EDGE('',*,*,#14041,.F.);
#18251=ORIENTED_EDGE('',*,*,#14044,.T.);
#18252=ORIENTED_EDGE('',*,*,#14042,.F.);
#18253=ORIENTED_EDGE('',*,*,#14045,.T.);
#18254=ORIENTED_EDGE('',*,*,#14046,.T.);
#18255=ORIENTED_EDGE('',*,*,#14047,.T.);
#18256=ORIENTED_EDGE('',*,*,#14048,.T.);
#18257=ORIENTED_EDGE('',*,*,#13962,.T.);
#18258=ORIENTED_EDGE('',*,*,#14046,.F.);
#18259=ORIENTED_EDGE('',*,*,#14049,.T.);
#18260=ORIENTED_EDGE('',*,*,#14048,.F.);
#18261=ORIENTED_EDGE('',*,*,#14050,.T.);
#18262=ORIENTED_EDGE('',*,*,#14033,.F.);
#18263=ORIENTED_EDGE('',*,*,#14051,.T.);
#18264=ORIENTED_EDGE('',*,*,#13997,.F.);
#18265=ORIENTED_EDGE('',*,*,#14052,.F.);
#18266=ORIENTED_EDGE('',*,*,#14047,.F.);
#18267=ORIENTED_EDGE('',*,*,#13961,.F.);
#18268=ORIENTED_EDGE('',*,*,#13950,.F.);
#18269=ORIENTED_EDGE('',*,*,#13967,.F.);
#18270=ORIENTED_EDGE('',*,*,#14053,.F.);
#18271=ORIENTED_EDGE('',*,*,#13963,.F.);
#18272=ORIENTED_EDGE('',*,*,#14051,.F.);
#18273=ORIENTED_EDGE('',*,*,#14021,.F.);
#18274=ORIENTED_EDGE('',*,*,#14054,.F.);
#18275=ORIENTED_EDGE('',*,*,#14017,.F.);
#18276=ORIENTED_EDGE('',*,*,#14055,.F.);
#18277=ORIENTED_EDGE('',*,*,#14013,.F.);
#18278=ORIENTED_EDGE('',*,*,#13992,.F.);
#18279=ORIENTED_EDGE('',*,*,#13959,.F.);
#18280=ORIENTED_EDGE('',*,*,#14056,.T.);
#18281=ORIENTED_EDGE('',*,*,#14057,.T.);
#18282=ORIENTED_EDGE('',*,*,#14058,.T.);
#18283=ORIENTED_EDGE('',*,*,#14059,.T.);
#18284=ORIENTED_EDGE('',*,*,#14060,.T.);
#18285=ORIENTED_EDGE('',*,*,#14061,.T.);
#18286=ORIENTED_EDGE('',*,*,#14062,.T.);
#18287=ORIENTED_EDGE('',*,*,#14063,.T.);
#18288=ORIENTED_EDGE('',*,*,#14064,.T.);
#18289=ORIENTED_EDGE('',*,*,#14065,.T.);
#18290=ORIENTED_EDGE('',*,*,#14066,.T.);
#18291=ORIENTED_EDGE('',*,*,#14067,.T.);
#18292=ORIENTED_EDGE('',*,*,#14068,.T.);
#18293=ORIENTED_EDGE('',*,*,#14069,.T.);
#18294=ORIENTED_EDGE('',*,*,#14070,.T.);
#18295=ORIENTED_EDGE('',*,*,#14071,.T.);
#18296=ORIENTED_EDGE('',*,*,#14072,.T.);
#18297=ORIENTED_EDGE('',*,*,#14073,.T.);
#18298=ORIENTED_EDGE('',*,*,#14074,.T.);
#18299=ORIENTED_EDGE('',*,*,#14075,.T.);
#18300=ORIENTED_EDGE('',*,*,#14076,.T.);
#18301=ORIENTED_EDGE('',*,*,#14077,.T.);
#18302=ORIENTED_EDGE('',*,*,#14078,.T.);
#18303=ORIENTED_EDGE('',*,*,#14079,.T.);
#18304=ORIENTED_EDGE('',*,*,#14080,.T.);
#18305=ORIENTED_EDGE('',*,*,#14081,.T.);
#18306=ORIENTED_EDGE('',*,*,#14082,.T.);
#18307=ORIENTED_EDGE('',*,*,#14083,.T.);
#18308=ORIENTED_EDGE('',*,*,#14084,.T.);
#18309=ORIENTED_EDGE('',*,*,#14085,.T.);
#18310=ORIENTED_EDGE('',*,*,#14086,.T.);
#18311=ORIENTED_EDGE('',*,*,#14087,.T.);
#18312=ORIENTED_EDGE('',*,*,#14088,.T.);
#18313=ORIENTED_EDGE('',*,*,#14089,.T.);
#18314=ORIENTED_EDGE('',*,*,#14090,.T.);
#18315=ORIENTED_EDGE('',*,*,#14091,.T.);
#18316=ORIENTED_EDGE('',*,*,#14092,.T.);
#18317=ORIENTED_EDGE('',*,*,#14093,.T.);
#18318=ORIENTED_EDGE('',*,*,#14094,.T.);
#18319=ORIENTED_EDGE('',*,*,#14095,.T.);
#18320=ORIENTED_EDGE('',*,*,#14096,.T.);
#18321=ORIENTED_EDGE('',*,*,#14097,.T.);
#18322=ORIENTED_EDGE('',*,*,#14098,.T.);
#18323=ORIENTED_EDGE('',*,*,#14099,.T.);
#18324=ORIENTED_EDGE('',*,*,#14100,.T.);
#18325=ORIENTED_EDGE('',*,*,#14101,.T.);
#18326=ORIENTED_EDGE('',*,*,#14102,.T.);
#18327=ORIENTED_EDGE('',*,*,#14103,.T.);
#18328=ORIENTED_EDGE('',*,*,#14104,.T.);
#18329=ORIENTED_EDGE('',*,*,#14105,.T.);
#18330=ORIENTED_EDGE('',*,*,#14106,.T.);
#18331=ORIENTED_EDGE('',*,*,#14107,.T.);
#18332=ORIENTED_EDGE('',*,*,#14108,.T.);
#18333=ORIENTED_EDGE('',*,*,#14109,.T.);
#18334=ORIENTED_EDGE('',*,*,#14110,.T.);
#18335=ORIENTED_EDGE('',*,*,#14111,.T.);
#18336=ORIENTED_EDGE('',*,*,#14112,.T.);
#18337=ORIENTED_EDGE('',*,*,#14113,.T.);
#18338=ORIENTED_EDGE('',*,*,#14114,.T.);
#18339=ORIENTED_EDGE('',*,*,#14115,.T.);
#18340=ORIENTED_EDGE('',*,*,#14116,.T.);
#18341=ORIENTED_EDGE('',*,*,#14117,.T.);
#18342=ORIENTED_EDGE('',*,*,#14118,.T.);
#18343=ORIENTED_EDGE('',*,*,#14034,.F.);
#18344=ORIENTED_EDGE('',*,*,#14050,.F.);
#18345=ORIENTED_EDGE('',*,*,#14049,.F.);
#18346=ORIENTED_EDGE('',*,*,#14045,.F.);
#18347=ORIENTED_EDGE('',*,*,#14044,.F.);
#18348=ORIENTED_EDGE('',*,*,#14040,.F.);
#18349=ORIENTED_EDGE('',*,*,#14039,.F.);
#18350=ORIENTED_EDGE('',*,*,#14035,.F.);
#18351=ORIENTED_EDGE('',*,*,#14119,.F.);
#18352=ORIENTED_EDGE('',*,*,#14120,.F.);
#18353=ORIENTED_EDGE('',*,*,#14121,.F.);
#18354=ORIENTED_EDGE('',*,*,#14122,.F.);
#18355=ORIENTED_EDGE('',*,*,#14123,.F.);
#18356=ORIENTED_EDGE('',*,*,#14124,.F.);
#18357=ORIENTED_EDGE('',*,*,#14125,.F.);
#18358=ORIENTED_EDGE('',*,*,#14126,.F.);
#18359=ORIENTED_EDGE('',*,*,#14127,.T.);
#18360=ORIENTED_EDGE('',*,*,#14128,.T.);
#18361=ORIENTED_EDGE('',*,*,#14129,.T.);
#18362=ORIENTED_EDGE('',*,*,#14130,.T.);
#18363=ORIENTED_EDGE('',*,*,#14054,.T.);
#18364=ORIENTED_EDGE('',*,*,#14131,.T.);
#18365=ORIENTED_EDGE('',*,*,#14019,.T.);
#18366=ORIENTED_EDGE('',*,*,#14132,.T.);
#18367=ORIENTED_EDGE('',*,*,#14133,.T.);
#18368=ORIENTED_EDGE('',*,*,#14132,.F.);
#18369=ORIENTED_EDGE('',*,*,#14018,.T.);
#18370=ORIENTED_EDGE('',*,*,#14130,.F.);
#18371=ORIENTED_EDGE('',*,*,#14134,.T.);
#18372=ORIENTED_EDGE('',*,*,#14127,.F.);
#18373=ORIENTED_EDGE('',*,*,#14020,.T.);
#18374=ORIENTED_EDGE('',*,*,#14131,.F.);
#18375=ORIENTED_EDGE('',*,*,#14135,.T.);
#18376=ORIENTED_EDGE('',*,*,#14133,.F.);
#18377=ORIENTED_EDGE('',*,*,#14134,.F.);
#18378=ORIENTED_EDGE('',*,*,#14129,.F.);
#18379=ORIENTED_EDGE('',*,*,#14136,.T.);
#18380=ORIENTED_EDGE('',*,*,#14137,.F.);
#18381=ORIENTED_EDGE('',*,*,#14138,.F.);
#18382=ORIENTED_EDGE('',*,*,#14139,.F.);
#18383=ORIENTED_EDGE('',*,*,#14140,.F.);
#18384=ORIENTED_EDGE('',*,*,#14141,.F.);
#18385=ORIENTED_EDGE('',*,*,#14136,.F.);
#18386=ORIENTED_EDGE('',*,*,#14128,.F.);
#18387=ORIENTED_EDGE('',*,*,#14135,.F.);
#18388=ORIENTED_EDGE('',*,*,#14142,.T.);
#18389=ORIENTED_EDGE('',*,*,#14143,.T.);
#18390=ORIENTED_EDGE('',*,*,#14144,.T.);
#18391=ORIENTED_EDGE('',*,*,#14145,.T.);
#18392=ORIENTED_EDGE('',*,*,#14053,.T.);
#18393=ORIENTED_EDGE('',*,*,#14146,.T.);
#18394=ORIENTED_EDGE('',*,*,#13965,.T.);
#18395=ORIENTED_EDGE('',*,*,#14147,.T.);
#18396=ORIENTED_EDGE('',*,*,#14148,.T.);
#18397=ORIENTED_EDGE('',*,*,#14147,.F.);
#18398=ORIENTED_EDGE('',*,*,#13964,.T.);
#18399=ORIENTED_EDGE('',*,*,#14145,.F.);
#18400=ORIENTED_EDGE('',*,*,#14149,.T.);
#18401=ORIENTED_EDGE('',*,*,#14142,.F.);
#18402=ORIENTED_EDGE('',*,*,#13966,.T.);
#18403=ORIENTED_EDGE('',*,*,#14146,.F.);
#18404=ORIENTED_EDGE('',*,*,#14150,.T.);
#18405=ORIENTED_EDGE('',*,*,#14148,.F.);
#18406=ORIENTED_EDGE('',*,*,#14149,.F.);
#18407=ORIENTED_EDGE('',*,*,#14144,.F.);
#18408=ORIENTED_EDGE('',*,*,#14151,.T.);
#18409=ORIENTED_EDGE('',*,*,#14152,.F.);
#18410=ORIENTED_EDGE('',*,*,#14153,.F.);
#18411=ORIENTED_EDGE('',*,*,#14154,.F.);
#18412=ORIENTED_EDGE('',*,*,#14155,.F.);
#18413=ORIENTED_EDGE('',*,*,#14156,.F.);
#18414=ORIENTED_EDGE('',*,*,#14151,.F.);
#18415=ORIENTED_EDGE('',*,*,#14143,.F.);
#18416=ORIENTED_EDGE('',*,*,#14150,.F.);
#18417=ORIENTED_EDGE('',*,*,#14157,.T.);
#18418=ORIENTED_EDGE('',*,*,#14158,.T.);
#18419=ORIENTED_EDGE('',*,*,#14159,.T.);
#18420=ORIENTED_EDGE('',*,*,#14119,.T.);
#18421=ORIENTED_EDGE('',*,*,#14160,.T.);
#18422=ORIENTED_EDGE('',*,*,#14161,.T.);
#18423=ORIENTED_EDGE('',*,*,#14157,.F.);
#18424=ORIENTED_EDGE('',*,*,#14126,.T.);
#18425=ORIENTED_EDGE('',*,*,#14162,.T.);
#18426=ORIENTED_EDGE('',*,*,#14163,.T.);
#18427=ORIENTED_EDGE('',*,*,#14160,.F.);
#18428=ORIENTED_EDGE('',*,*,#14125,.T.);
#18429=ORIENTED_EDGE('',*,*,#14164,.T.);
#18430=ORIENTED_EDGE('',*,*,#14165,.T.);
#18431=ORIENTED_EDGE('',*,*,#14162,.F.);
#18432=ORIENTED_EDGE('',*,*,#14124,.T.);
#18433=ORIENTED_EDGE('',*,*,#14166,.T.);
#18434=ORIENTED_EDGE('',*,*,#13889,.T.);
#18435=ORIENTED_EDGE('',*,*,#14164,.F.);
#18436=ORIENTED_EDGE('',*,*,#14123,.T.);
#18437=ORIENTED_EDGE('',*,*,#14167,.T.);
#18438=ORIENTED_EDGE('',*,*,#14168,.T.);
#18439=ORIENTED_EDGE('',*,*,#14166,.F.);
#18440=ORIENTED_EDGE('',*,*,#14122,.T.);
#18441=ORIENTED_EDGE('',*,*,#14169,.T.);
#18442=ORIENTED_EDGE('',*,*,#14170,.T.);
#18443=ORIENTED_EDGE('',*,*,#14167,.F.);
#18444=ORIENTED_EDGE('',*,*,#14121,.T.);
#18445=ORIENTED_EDGE('',*,*,#14159,.F.);
#18446=ORIENTED_EDGE('',*,*,#14171,.T.);
#18447=ORIENTED_EDGE('',*,*,#14169,.F.);
#18448=ORIENTED_EDGE('',*,*,#14120,.T.);
#18449=ORIENTED_EDGE('',*,*,#14168,.F.);
#18450=ORIENTED_EDGE('',*,*,#14172,.T.);
#18451=ORIENTED_EDGE('',*,*,#14173,.F.);
#18452=ORIENTED_EDGE('',*,*,#13890,.T.);
#18453=ORIENTED_EDGE('',*,*,#14170,.F.);
#18454=ORIENTED_EDGE('',*,*,#14174,.F.);
#18455=ORIENTED_EDGE('',*,*,#14175,.F.);
#18456=ORIENTED_EDGE('',*,*,#14172,.F.);
#18457=ORIENTED_EDGE('',*,*,#14171,.F.);
#18458=ORIENTED_EDGE('',*,*,#14176,.T.);
#18459=ORIENTED_EDGE('',*,*,#14177,.F.);
#18460=ORIENTED_EDGE('',*,*,#14178,.F.);
#18461=ORIENTED_EDGE('',*,*,#14179,.F.);
#18462=ORIENTED_EDGE('',*,*,#14180,.F.);
#18463=ORIENTED_EDGE('',*,*,#14181,.F.);
#18464=ORIENTED_EDGE('',*,*,#14182,.F.);
#18465=ORIENTED_EDGE('',*,*,#14183,.T.);
#18466=ORIENTED_EDGE('',*,*,#14184,.F.);
#18467=ORIENTED_EDGE('',*,*,#14185,.F.);
#18468=ORIENTED_EDGE('',*,*,#14186,.F.);
#18469=ORIENTED_EDGE('',*,*,#14187,.F.);
#18470=ORIENTED_EDGE('',*,*,#14188,.F.);
#18471=ORIENTED_EDGE('',*,*,#14189,.F.);
#18472=ORIENTED_EDGE('',*,*,#14190,.T.);
#18473=ORIENTED_EDGE('',*,*,#14191,.F.);
#18474=ORIENTED_EDGE('',*,*,#14174,.T.);
#18475=ORIENTED_EDGE('',*,*,#14158,.F.);
#18476=ORIENTED_EDGE('',*,*,#14192,.F.);
#18477=ORIENTED_EDGE('',*,*,#14193,.F.);
#18478=ORIENTED_EDGE('',*,*,#14194,.F.);
#18479=ORIENTED_EDGE('',*,*,#14195,.F.);
#18480=ORIENTED_EDGE('',*,*,#14196,.F.);
#18481=ORIENTED_EDGE('',*,*,#14197,.F.);
#18482=ORIENTED_EDGE('',*,*,#14190,.F.);
#18483=ORIENTED_EDGE('',*,*,#14198,.F.);
#18484=ORIENTED_EDGE('',*,*,#14183,.F.);
#18485=ORIENTED_EDGE('',*,*,#14199,.F.);
#18486=ORIENTED_EDGE('',*,*,#14176,.F.);
#18487=ORIENTED_EDGE('',*,*,#14200,.T.);
#18488=ORIENTED_EDGE('',*,*,#14139,.T.);
#18489=ORIENTED_EDGE('',*,*,#14201,.F.);
#18490=ORIENTED_EDGE('',*,*,#14180,.T.);
#18491=ORIENTED_EDGE('',*,*,#14179,.T.);
#18492=ORIENTED_EDGE('',*,*,#14178,.T.);
#18493=ORIENTED_EDGE('',*,*,#14202,.T.);
#18494=ORIENTED_EDGE('',*,*,#14137,.T.);
#18495=ORIENTED_EDGE('',*,*,#14141,.T.);
#18496=ORIENTED_EDGE('',*,*,#14203,.T.);
#18497=ORIENTED_EDGE('',*,*,#14199,.T.);
#18498=ORIENTED_EDGE('',*,*,#14202,.F.);
#18499=ORIENTED_EDGE('',*,*,#14182,.T.);
#18500=ORIENTED_EDGE('',*,*,#14181,.T.);
#18501=ORIENTED_EDGE('',*,*,#14201,.T.);
#18502=ORIENTED_EDGE('',*,*,#14138,.T.);
#18503=ORIENTED_EDGE('',*,*,#14200,.F.);
#18504=ORIENTED_EDGE('',*,*,#14177,.T.);
#18505=ORIENTED_EDGE('',*,*,#14203,.F.);
#18506=ORIENTED_EDGE('',*,*,#14140,.T.);
#18507=ORIENTED_EDGE('',*,*,#14204,.T.);
#18508=ORIENTED_EDGE('',*,*,#14024,.T.);
#18509=ORIENTED_EDGE('',*,*,#14205,.T.);
#18510=ORIENTED_EDGE('',*,*,#14197,.T.);
#18511=ORIENTED_EDGE('',*,*,#14204,.F.);
#18512=ORIENTED_EDGE('',*,*,#14206,.T.);
#18513=ORIENTED_EDGE('',*,*,#14207,.T.);
#18514=ORIENTED_EDGE('',*,*,#14025,.T.);
#18515=ORIENTED_EDGE('',*,*,#14208,.T.);
#18516=ORIENTED_EDGE('',*,*,#14026,.T.);
#18517=ORIENTED_EDGE('',*,*,#14207,.F.);
#18518=ORIENTED_EDGE('',*,*,#14209,.T.);
#18519=ORIENTED_EDGE('',*,*,#14208,.F.);
#18520=ORIENTED_EDGE('',*,*,#14210,.T.);
#18521=ORIENTED_EDGE('',*,*,#14211,.T.);
#18522=ORIENTED_EDGE('',*,*,#14027,.T.);
#18523=ORIENTED_EDGE('',*,*,#14212,.T.);
#18524=ORIENTED_EDGE('',*,*,#14028,.T.);
#18525=ORIENTED_EDGE('',*,*,#14211,.F.);
#18526=ORIENTED_EDGE('',*,*,#13891,.T.);
#18527=ORIENTED_EDGE('',*,*,#14212,.F.);
#18528=ORIENTED_EDGE('',*,*,#14173,.T.);
#18529=ORIENTED_EDGE('',*,*,#14213,.T.);
#18530=ORIENTED_EDGE('',*,*,#14029,.T.);
#18531=ORIENTED_EDGE('',*,*,#14214,.T.);
#18532=ORIENTED_EDGE('',*,*,#14030,.T.);
#18533=ORIENTED_EDGE('',*,*,#14213,.F.);
#18534=ORIENTED_EDGE('',*,*,#14175,.T.);
#18535=ORIENTED_EDGE('',*,*,#14214,.F.);
#18536=ORIENTED_EDGE('',*,*,#14191,.T.);
#18537=ORIENTED_EDGE('',*,*,#14205,.F.);
#18538=ORIENTED_EDGE('',*,*,#14031,.T.);
#18539=ORIENTED_EDGE('',*,*,#14165,.F.);
#18540=ORIENTED_EDGE('',*,*,#13892,.T.);
#18541=ORIENTED_EDGE('',*,*,#14210,.F.);
#18542=ORIENTED_EDGE('',*,*,#14215,.T.);
#18543=ORIENTED_EDGE('',*,*,#14163,.F.);
#18544=ORIENTED_EDGE('',*,*,#14215,.F.);
#18545=ORIENTED_EDGE('',*,*,#14209,.F.);
#18546=ORIENTED_EDGE('',*,*,#14216,.F.);
#18547=ORIENTED_EDGE('',*,*,#14161,.F.);
#18548=ORIENTED_EDGE('',*,*,#14216,.T.);
#18549=ORIENTED_EDGE('',*,*,#14206,.F.);
#18550=ORIENTED_EDGE('',*,*,#14196,.T.);
#18551=ORIENTED_EDGE('',*,*,#14217,.F.);
#18552=ORIENTED_EDGE('',*,*,#14218,.F.);
#18553=ORIENTED_EDGE('',*,*,#14219,.F.);
#18554=ORIENTED_EDGE('',*,*,#14220,.F.);
#18555=ORIENTED_EDGE('',*,*,#14221,.F.);
#18556=ORIENTED_EDGE('',*,*,#14222,.F.);
#18557=ORIENTED_EDGE('',*,*,#14194,.T.);
#18558=ORIENTED_EDGE('',*,*,#14223,.F.);
#18559=ORIENTED_EDGE('',*,*,#14224,.F.);
#18560=ORIENTED_EDGE('',*,*,#14225,.F.);
#18561=ORIENTED_EDGE('',*,*,#14226,.F.);
#18562=ORIENTED_EDGE('',*,*,#14227,.F.);
#18563=ORIENTED_EDGE('',*,*,#14228,.F.);
#18564=ORIENTED_EDGE('',*,*,#14192,.T.);
#18565=ORIENTED_EDGE('',*,*,#14229,.T.);
#18566=ORIENTED_EDGE('',*,*,#13971,.T.);
#18567=ORIENTED_EDGE('',*,*,#14230,.F.);
#18568=ORIENTED_EDGE('',*,*,#14220,.T.);
#18569=ORIENTED_EDGE('',*,*,#14219,.T.);
#18570=ORIENTED_EDGE('',*,*,#14218,.T.);
#18571=ORIENTED_EDGE('',*,*,#14231,.T.);
#18572=ORIENTED_EDGE('',*,*,#13969,.T.);
#18573=ORIENTED_EDGE('',*,*,#13973,.T.);
#18574=ORIENTED_EDGE('',*,*,#14232,.T.);
#18575=ORIENTED_EDGE('',*,*,#14195,.T.);
#18576=ORIENTED_EDGE('',*,*,#14231,.F.);
#18577=ORIENTED_EDGE('',*,*,#14222,.T.);
#18578=ORIENTED_EDGE('',*,*,#14221,.T.);
#18579=ORIENTED_EDGE('',*,*,#14230,.T.);
#18580=ORIENTED_EDGE('',*,*,#13970,.T.);
#18581=ORIENTED_EDGE('',*,*,#14229,.F.);
#18582=ORIENTED_EDGE('',*,*,#14217,.T.);
#18583=ORIENTED_EDGE('',*,*,#14232,.F.);
#18584=ORIENTED_EDGE('',*,*,#13972,.T.);
#18585=ORIENTED_EDGE('',*,*,#14233,.T.);
#18586=ORIENTED_EDGE('',*,*,#14154,.T.);
#18587=ORIENTED_EDGE('',*,*,#14234,.F.);
#18588=ORIENTED_EDGE('',*,*,#14226,.T.);
#18589=ORIENTED_EDGE('',*,*,#14225,.T.);
#18590=ORIENTED_EDGE('',*,*,#14224,.T.);
#18591=ORIENTED_EDGE('',*,*,#14235,.T.);
#18592=ORIENTED_EDGE('',*,*,#14152,.T.);
#18593=ORIENTED_EDGE('',*,*,#14156,.T.);
#18594=ORIENTED_EDGE('',*,*,#14236,.T.);
#18595=ORIENTED_EDGE('',*,*,#14193,.T.);
#18596=ORIENTED_EDGE('',*,*,#14235,.F.);
#18597=ORIENTED_EDGE('',*,*,#14228,.T.);
#18598=ORIENTED_EDGE('',*,*,#14227,.T.);
#18599=ORIENTED_EDGE('',*,*,#14234,.T.);
#18600=ORIENTED_EDGE('',*,*,#14153,.T.);
#18601=ORIENTED_EDGE('',*,*,#14233,.F.);
#18602=ORIENTED_EDGE('',*,*,#14223,.T.);
#18603=ORIENTED_EDGE('',*,*,#14236,.F.);
#18604=ORIENTED_EDGE('',*,*,#14155,.T.);
#18605=ORIENTED_EDGE('',*,*,#14237,.T.);
#18606=ORIENTED_EDGE('',*,*,#14238,.T.);
#18607=ORIENTED_EDGE('',*,*,#14239,.T.);
#18608=ORIENTED_EDGE('',*,*,#14240,.T.);
#18609=ORIENTED_EDGE('',*,*,#14055,.T.);
#18610=ORIENTED_EDGE('',*,*,#14241,.T.);
#18611=ORIENTED_EDGE('',*,*,#14015,.T.);
#18612=ORIENTED_EDGE('',*,*,#14242,.T.);
#18613=ORIENTED_EDGE('',*,*,#14243,.T.);
#18614=ORIENTED_EDGE('',*,*,#14242,.F.);
#18615=ORIENTED_EDGE('',*,*,#14014,.T.);
#18616=ORIENTED_EDGE('',*,*,#14240,.F.);
#18617=ORIENTED_EDGE('',*,*,#14244,.T.);
#18618=ORIENTED_EDGE('',*,*,#14237,.F.);
#18619=ORIENTED_EDGE('',*,*,#14016,.T.);
#18620=ORIENTED_EDGE('',*,*,#14241,.F.);
#18621=ORIENTED_EDGE('',*,*,#14245,.T.);
#18622=ORIENTED_EDGE('',*,*,#14243,.F.);
#18623=ORIENTED_EDGE('',*,*,#14244,.F.);
#18624=ORIENTED_EDGE('',*,*,#14239,.F.);
#18625=ORIENTED_EDGE('',*,*,#14246,.T.);
#18626=ORIENTED_EDGE('',*,*,#14247,.F.);
#18627=ORIENTED_EDGE('',*,*,#14248,.F.);
#18628=ORIENTED_EDGE('',*,*,#14249,.F.);
#18629=ORIENTED_EDGE('',*,*,#14250,.F.);
#18630=ORIENTED_EDGE('',*,*,#14251,.F.);
#18631=ORIENTED_EDGE('',*,*,#14246,.F.);
#18632=ORIENTED_EDGE('',*,*,#14238,.F.);
#18633=ORIENTED_EDGE('',*,*,#14245,.F.);
#18634=ORIENTED_EDGE('',*,*,#14252,.T.);
#18635=ORIENTED_EDGE('',*,*,#14249,.T.);
#18636=ORIENTED_EDGE('',*,*,#14253,.F.);
#18637=ORIENTED_EDGE('',*,*,#14187,.T.);
#18638=ORIENTED_EDGE('',*,*,#14186,.T.);
#18639=ORIENTED_EDGE('',*,*,#14185,.T.);
#18640=ORIENTED_EDGE('',*,*,#14254,.T.);
#18641=ORIENTED_EDGE('',*,*,#14247,.T.);
#18642=ORIENTED_EDGE('',*,*,#14251,.T.);
#18643=ORIENTED_EDGE('',*,*,#14255,.T.);
#18644=ORIENTED_EDGE('',*,*,#14198,.T.);
#18645=ORIENTED_EDGE('',*,*,#14254,.F.);
#18646=ORIENTED_EDGE('',*,*,#14189,.T.);
#18647=ORIENTED_EDGE('',*,*,#14188,.T.);
#18648=ORIENTED_EDGE('',*,*,#14253,.T.);
#18649=ORIENTED_EDGE('',*,*,#14248,.T.);
#18650=ORIENTED_EDGE('',*,*,#14252,.F.);
#18651=ORIENTED_EDGE('',*,*,#14184,.T.);
#18652=ORIENTED_EDGE('',*,*,#14255,.F.);
#18653=ORIENTED_EDGE('',*,*,#14250,.T.);
#18654=ORIENTED_EDGE('',*,*,#14256,.T.);
#18655=ORIENTED_EDGE('',*,*,#14257,.T.);
#18656=ORIENTED_EDGE('',*,*,#14258,.T.);
#18657=ORIENTED_EDGE('',*,*,#14259,.T.);
#18658=ORIENTED_EDGE('',*,*,#14260,.T.);
#18659=ORIENTED_EDGE('',*,*,#14261,.T.);
#18660=ORIENTED_EDGE('',*,*,#14256,.F.);
#18661=ORIENTED_EDGE('',*,*,#14262,.T.);
#18662=ORIENTED_EDGE('',*,*,#14263,.T.);
#18663=ORIENTED_EDGE('',*,*,#14264,.T.);
#18664=ORIENTED_EDGE('',*,*,#14260,.F.);
#18665=ORIENTED_EDGE('',*,*,#14265,.T.);
#18666=ORIENTED_EDGE('',*,*,#14266,.T.);
#18667=ORIENTED_EDGE('',*,*,#14267,.T.);
#18668=ORIENTED_EDGE('',*,*,#14263,.F.);
#18669=ORIENTED_EDGE('',*,*,#14268,.T.);
#18670=ORIENTED_EDGE('',*,*,#14269,.T.);
#18671=ORIENTED_EDGE('',*,*,#14270,.T.);
#18672=ORIENTED_EDGE('',*,*,#14266,.F.);
#18673=ORIENTED_EDGE('',*,*,#14271,.T.);
#18674=ORIENTED_EDGE('',*,*,#14272,.T.);
#18675=ORIENTED_EDGE('',*,*,#13976,.T.);
#18676=ORIENTED_EDGE('',*,*,#14269,.F.);
#18677=ORIENTED_EDGE('',*,*,#14273,.T.);
#18678=ORIENTED_EDGE('',*,*,#14274,.T.);
#18679=ORIENTED_EDGE('',*,*,#14275,.T.);
#18680=ORIENTED_EDGE('',*,*,#14272,.F.);
#18681=ORIENTED_EDGE('',*,*,#14276,.T.);
#18682=ORIENTED_EDGE('',*,*,#14258,.F.);
#18683=ORIENTED_EDGE('',*,*,#14277,.T.);
#18684=ORIENTED_EDGE('',*,*,#14274,.F.);
#18685=ORIENTED_EDGE('',*,*,#14278,.T.);
#18686=ORIENTED_EDGE('',*,*,#14275,.F.);
#18687=ORIENTED_EDGE('',*,*,#14279,.T.);
#18688=ORIENTED_EDGE('',*,*,#14280,.T.);
#18689=ORIENTED_EDGE('',*,*,#14281,.T.);
#18690=ORIENTED_EDGE('',*,*,#14282,.F.);
#18691=ORIENTED_EDGE('',*,*,#13977,.T.);
#18692=ORIENTED_EDGE('',*,*,#14277,.F.);
#18693=ORIENTED_EDGE('',*,*,#14283,.F.);
#18694=ORIENTED_EDGE('',*,*,#14284,.T.);
#18695=ORIENTED_EDGE('',*,*,#14279,.F.);
#18696=ORIENTED_EDGE('',*,*,#14257,.F.);
#18697=ORIENTED_EDGE('',*,*,#14285,.T.);
#18698=ORIENTED_EDGE('',*,*,#14286,.F.);
#18699=ORIENTED_EDGE('',*,*,#14287,.F.);
#18700=ORIENTED_EDGE('',*,*,#14288,.F.);
#18701=ORIENTED_EDGE('',*,*,#14289,.T.);
#18702=ORIENTED_EDGE('',*,*,#14290,.F.);
#18703=ORIENTED_EDGE('',*,*,#14291,.F.);
#18704=ORIENTED_EDGE('',*,*,#14292,.F.);
#18705=ORIENTED_EDGE('',*,*,#14293,.T.);
#18706=ORIENTED_EDGE('',*,*,#14294,.F.);
#18707=ORIENTED_EDGE('',*,*,#14295,.T.);
#18708=ORIENTED_EDGE('',*,*,#14296,.T.);
#18709=ORIENTED_EDGE('',*,*,#14283,.T.);
#18710=ORIENTED_EDGE('',*,*,#14259,.F.);
#18711=ORIENTED_EDGE('',*,*,#14278,.F.);
#18712=ORIENTED_EDGE('',*,*,#14276,.F.);
#18713=ORIENTED_EDGE('',*,*,#14273,.F.);
#18714=ORIENTED_EDGE('',*,*,#14271,.F.);
#18715=ORIENTED_EDGE('',*,*,#14268,.F.);
#18716=ORIENTED_EDGE('',*,*,#14265,.F.);
#18717=ORIENTED_EDGE('',*,*,#14262,.F.);
#18718=ORIENTED_EDGE('',*,*,#14297,.F.);
#18719=ORIENTED_EDGE('',*,*,#14298,.F.);
#18720=ORIENTED_EDGE('',*,*,#14299,.F.);
#18721=ORIENTED_EDGE('',*,*,#14300,.F.);
#18722=ORIENTED_EDGE('',*,*,#14301,.F.);
#18723=ORIENTED_EDGE('',*,*,#14302,.F.);
#18724=ORIENTED_EDGE('',*,*,#14303,.F.);
#18725=ORIENTED_EDGE('',*,*,#14304,.F.);
#18726=ORIENTED_EDGE('',*,*,#14305,.T.);
#18727=ORIENTED_EDGE('',*,*,#14294,.T.);
#18728=ORIENTED_EDGE('',*,*,#14306,.T.);
#18729=ORIENTED_EDGE('',*,*,#14307,.T.);
#18730=ORIENTED_EDGE('',*,*,#14305,.F.);
#18731=ORIENTED_EDGE('',*,*,#14308,.T.);
#18732=ORIENTED_EDGE('',*,*,#14309,.T.);
#18733=ORIENTED_EDGE('',*,*,#14310,.T.);
#18734=ORIENTED_EDGE('',*,*,#14311,.T.);
#18735=ORIENTED_EDGE('',*,*,#14282,.T.);
#18736=ORIENTED_EDGE('',*,*,#14309,.F.);
#18737=ORIENTED_EDGE('',*,*,#14312,.T.);
#18738=ORIENTED_EDGE('',*,*,#14311,.F.);
#18739=ORIENTED_EDGE('',*,*,#14313,.T.);
#18740=ORIENTED_EDGE('',*,*,#14314,.T.);
#18741=ORIENTED_EDGE('',*,*,#13978,.T.);
#18742=ORIENTED_EDGE('',*,*,#14315,.T.);
#18743=ORIENTED_EDGE('',*,*,#14316,.T.);
#18744=ORIENTED_EDGE('',*,*,#14314,.F.);
#18745=ORIENTED_EDGE('',*,*,#14317,.T.);
#18746=ORIENTED_EDGE('',*,*,#14315,.F.);
#18747=ORIENTED_EDGE('',*,*,#14318,.T.);
#18748=ORIENTED_EDGE('',*,*,#14319,.T.);
#18749=ORIENTED_EDGE('',*,*,#14320,.T.);
#18750=ORIENTED_EDGE('',*,*,#14321,.T.);
#18751=ORIENTED_EDGE('',*,*,#14322,.T.);
#18752=ORIENTED_EDGE('',*,*,#14319,.F.);
#18753=ORIENTED_EDGE('',*,*,#14323,.T.);
#18754=ORIENTED_EDGE('',*,*,#14321,.F.);
#18755=ORIENTED_EDGE('',*,*,#14324,.T.);
#18756=ORIENTED_EDGE('',*,*,#14306,.F.);
#18757=ORIENTED_EDGE('',*,*,#14325,.T.);
#18758=ORIENTED_EDGE('',*,*,#14267,.F.);
#18759=ORIENTED_EDGE('',*,*,#14326,.F.);
#18760=ORIENTED_EDGE('',*,*,#14320,.F.);
#18761=ORIENTED_EDGE('',*,*,#14327,.F.);
#18762=ORIENTED_EDGE('',*,*,#14264,.F.);
#18763=ORIENTED_EDGE('',*,*,#14327,.T.);
#18764=ORIENTED_EDGE('',*,*,#14322,.F.);
#18765=ORIENTED_EDGE('',*,*,#14328,.T.);
#18766=ORIENTED_EDGE('',*,*,#14329,.F.);
#18767=ORIENTED_EDGE('',*,*,#14330,.F.);
#18768=ORIENTED_EDGE('',*,*,#14331,.F.);
#18769=ORIENTED_EDGE('',*,*,#14332,.T.);
#18770=ORIENTED_EDGE('',*,*,#14333,.F.);
#18771=ORIENTED_EDGE('',*,*,#14334,.F.);
#18772=ORIENTED_EDGE('',*,*,#14335,.F.);
#18773=ORIENTED_EDGE('',*,*,#14336,.T.);
#18774=ORIENTED_EDGE('',*,*,#14261,.F.);
#18775=ORIENTED_EDGE('',*,*,#14336,.F.);
#18776=ORIENTED_EDGE('',*,*,#14337,.F.);
#18777=ORIENTED_EDGE('',*,*,#14332,.F.);
#18778=ORIENTED_EDGE('',*,*,#14338,.F.);
#18779=ORIENTED_EDGE('',*,*,#14328,.F.);
#18780=ORIENTED_EDGE('',*,*,#14325,.F.);
#18781=ORIENTED_EDGE('',*,*,#14293,.F.);
#18782=ORIENTED_EDGE('',*,*,#14339,.F.);
#18783=ORIENTED_EDGE('',*,*,#14289,.F.);
#18784=ORIENTED_EDGE('',*,*,#14340,.F.);
#18785=ORIENTED_EDGE('',*,*,#14285,.F.);
#18786=ORIENTED_EDGE('',*,*,#14307,.F.);
#18787=ORIENTED_EDGE('',*,*,#14324,.F.);
#18788=ORIENTED_EDGE('',*,*,#14323,.F.);
#18789=ORIENTED_EDGE('',*,*,#14318,.F.);
#18790=ORIENTED_EDGE('',*,*,#14317,.F.);
#18791=ORIENTED_EDGE('',*,*,#14313,.F.);
#18792=ORIENTED_EDGE('',*,*,#14312,.F.);
#18793=ORIENTED_EDGE('',*,*,#14308,.F.);
#18794=ORIENTED_EDGE('',*,*,#14341,.F.);
#18795=ORIENTED_EDGE('',*,*,#14342,.F.);
#18796=ORIENTED_EDGE('',*,*,#14343,.F.);
#18797=ORIENTED_EDGE('',*,*,#14344,.F.);
#18798=ORIENTED_EDGE('',*,*,#14345,.F.);
#18799=ORIENTED_EDGE('',*,*,#14346,.F.);
#18800=ORIENTED_EDGE('',*,*,#14347,.F.);
#18801=ORIENTED_EDGE('',*,*,#14348,.F.);
#18802=ORIENTED_EDGE('',*,*,#14349,.T.);
#18803=ORIENTED_EDGE('',*,*,#14330,.T.);
#18804=ORIENTED_EDGE('',*,*,#14350,.T.);
#18805=ORIENTED_EDGE('',*,*,#14351,.T.);
#18806=ORIENTED_EDGE('',*,*,#14352,.T.);
#18807=ORIENTED_EDGE('',*,*,#14353,.T.);
#18808=ORIENTED_EDGE('',*,*,#14354,.T.);
#18809=ORIENTED_EDGE('',*,*,#14355,.T.);
#18810=ORIENTED_EDGE('',*,*,#14338,.T.);
#18811=ORIENTED_EDGE('',*,*,#14352,.F.);
#18812=ORIENTED_EDGE('',*,*,#14331,.T.);
#18813=ORIENTED_EDGE('',*,*,#14349,.F.);
#18814=ORIENTED_EDGE('',*,*,#14356,.T.);
#18815=ORIENTED_EDGE('',*,*,#14350,.F.);
#18816=ORIENTED_EDGE('',*,*,#14329,.T.);
#18817=ORIENTED_EDGE('',*,*,#14355,.F.);
#18818=ORIENTED_EDGE('',*,*,#14357,.T.);
#18819=ORIENTED_EDGE('',*,*,#14353,.F.);
#18820=ORIENTED_EDGE('',*,*,#14356,.F.);
#18821=ORIENTED_EDGE('',*,*,#14351,.F.);
#18822=ORIENTED_EDGE('',*,*,#14357,.F.);
#18823=ORIENTED_EDGE('',*,*,#14354,.F.);
#18824=ORIENTED_EDGE('',*,*,#14358,.T.);
#18825=ORIENTED_EDGE('',*,*,#14359,.F.);
#18826=ORIENTED_EDGE('',*,*,#14360,.F.);
#18827=ORIENTED_EDGE('',*,*,#14361,.F.);
#18828=ORIENTED_EDGE('',*,*,#14362,.F.);
#18829=ORIENTED_EDGE('',*,*,#14363,.F.);
#18830=ORIENTED_EDGE('',*,*,#14358,.F.);
#18831=ORIENTED_EDGE('',*,*,#14364,.T.);
#18832=ORIENTED_EDGE('',*,*,#14341,.T.);
#18833=ORIENTED_EDGE('',*,*,#14365,.T.);
#18834=ORIENTED_EDGE('',*,*,#14366,.T.);
#18835=ORIENTED_EDGE('',*,*,#14364,.F.);
#18836=ORIENTED_EDGE('',*,*,#14367,.T.);
#18837=ORIENTED_EDGE('',*,*,#14368,.T.);
#18838=ORIENTED_EDGE('',*,*,#14342,.T.);
#18839=ORIENTED_EDGE('',*,*,#14369,.T.);
#18840=ORIENTED_EDGE('',*,*,#14343,.T.);
#18841=ORIENTED_EDGE('',*,*,#14368,.F.);
#18842=ORIENTED_EDGE('',*,*,#14370,.T.);
#18843=ORIENTED_EDGE('',*,*,#14369,.F.);
#18844=ORIENTED_EDGE('',*,*,#14371,.T.);
#18845=ORIENTED_EDGE('',*,*,#14372,.T.);
#18846=ORIENTED_EDGE('',*,*,#14344,.T.);
#18847=ORIENTED_EDGE('',*,*,#14373,.T.);
#18848=ORIENTED_EDGE('',*,*,#14345,.T.);
#18849=ORIENTED_EDGE('',*,*,#14372,.F.);
#18850=ORIENTED_EDGE('',*,*,#13925,.T.);
#18851=ORIENTED_EDGE('',*,*,#14373,.F.);
#18852=ORIENTED_EDGE('',*,*,#14374,.T.);
#18853=ORIENTED_EDGE('',*,*,#14375,.T.);
#18854=ORIENTED_EDGE('',*,*,#14346,.T.);
#18855=ORIENTED_EDGE('',*,*,#14376,.T.);
#18856=ORIENTED_EDGE('',*,*,#14347,.T.);
#18857=ORIENTED_EDGE('',*,*,#14375,.F.);
#18858=ORIENTED_EDGE('',*,*,#14377,.T.);
#18859=ORIENTED_EDGE('',*,*,#14376,.F.);
#18860=ORIENTED_EDGE('',*,*,#14378,.T.);
#18861=ORIENTED_EDGE('',*,*,#14365,.F.);
#18862=ORIENTED_EDGE('',*,*,#14348,.T.);
#18863=ORIENTED_EDGE('',*,*,#14371,.F.);
#18864=ORIENTED_EDGE('',*,*,#14379,.T.);
#18865=ORIENTED_EDGE('',*,*,#14380,.F.);
#18866=ORIENTED_EDGE('',*,*,#13926,.T.);
#18867=ORIENTED_EDGE('',*,*,#14370,.F.);
#18868=ORIENTED_EDGE('',*,*,#14381,.F.);
#18869=ORIENTED_EDGE('',*,*,#14382,.F.);
#18870=ORIENTED_EDGE('',*,*,#14379,.F.);
#18871=ORIENTED_EDGE('',*,*,#14367,.F.);
#18872=ORIENTED_EDGE('',*,*,#14383,.T.);
#18873=ORIENTED_EDGE('',*,*,#14384,.F.);
#18874=ORIENTED_EDGE('',*,*,#14385,.F.);
#18875=ORIENTED_EDGE('',*,*,#14386,.F.);
#18876=ORIENTED_EDGE('',*,*,#14387,.F.);
#18877=ORIENTED_EDGE('',*,*,#14388,.F.);
#18878=ORIENTED_EDGE('',*,*,#14389,.T.);
#18879=ORIENTED_EDGE('',*,*,#14390,.F.);
#18880=ORIENTED_EDGE('',*,*,#14391,.F.);
#18881=ORIENTED_EDGE('',*,*,#14392,.F.);
#18882=ORIENTED_EDGE('',*,*,#14393,.F.);
#18883=ORIENTED_EDGE('',*,*,#14394,.F.);
#18884=ORIENTED_EDGE('',*,*,#14395,.F.);
#18885=ORIENTED_EDGE('',*,*,#14396,.T.);
#18886=ORIENTED_EDGE('',*,*,#14397,.F.);
#18887=ORIENTED_EDGE('',*,*,#14381,.T.);
#18888=ORIENTED_EDGE('',*,*,#14366,.F.);
#18889=ORIENTED_EDGE('',*,*,#14398,.F.);
#18890=ORIENTED_EDGE('',*,*,#14399,.F.);
#18891=ORIENTED_EDGE('',*,*,#14400,.F.);
#18892=ORIENTED_EDGE('',*,*,#14401,.F.);
#18893=ORIENTED_EDGE('',*,*,#14402,.F.);
#18894=ORIENTED_EDGE('',*,*,#14403,.F.);
#18895=ORIENTED_EDGE('',*,*,#14396,.F.);
#18896=ORIENTED_EDGE('',*,*,#14404,.F.);
#18897=ORIENTED_EDGE('',*,*,#14389,.F.);
#18898=ORIENTED_EDGE('',*,*,#14405,.F.);
#18899=ORIENTED_EDGE('',*,*,#14383,.F.);
#18900=ORIENTED_EDGE('',*,*,#14406,.T.);
#18901=ORIENTED_EDGE('',*,*,#14403,.T.);
#18902=ORIENTED_EDGE('',*,*,#14407,.T.);
#18903=ORIENTED_EDGE('',*,*,#14297,.T.);
#18904=ORIENTED_EDGE('',*,*,#14408,.T.);
#18905=ORIENTED_EDGE('',*,*,#14397,.T.);
#18906=ORIENTED_EDGE('',*,*,#14406,.F.);
#18907=ORIENTED_EDGE('',*,*,#14304,.T.);
#18908=ORIENTED_EDGE('',*,*,#14409,.T.);
#18909=ORIENTED_EDGE('',*,*,#14382,.T.);
#18910=ORIENTED_EDGE('',*,*,#14408,.F.);
#18911=ORIENTED_EDGE('',*,*,#14303,.T.);
#18912=ORIENTED_EDGE('',*,*,#14410,.T.);
#18913=ORIENTED_EDGE('',*,*,#14380,.T.);
#18914=ORIENTED_EDGE('',*,*,#14409,.F.);
#18915=ORIENTED_EDGE('',*,*,#14302,.T.);
#18916=ORIENTED_EDGE('',*,*,#14411,.T.);
#18917=ORIENTED_EDGE('',*,*,#13927,.T.);
#18918=ORIENTED_EDGE('',*,*,#14410,.F.);
#18919=ORIENTED_EDGE('',*,*,#14301,.T.);
#18920=ORIENTED_EDGE('',*,*,#14412,.T.);
#18921=ORIENTED_EDGE('',*,*,#14413,.T.);
#18922=ORIENTED_EDGE('',*,*,#14411,.F.);
#18923=ORIENTED_EDGE('',*,*,#14300,.T.);
#18924=ORIENTED_EDGE('',*,*,#14414,.T.);
#18925=ORIENTED_EDGE('',*,*,#14415,.T.);
#18926=ORIENTED_EDGE('',*,*,#14412,.F.);
#18927=ORIENTED_EDGE('',*,*,#14299,.T.);
#18928=ORIENTED_EDGE('',*,*,#14407,.F.);
#18929=ORIENTED_EDGE('',*,*,#14416,.T.);
#18930=ORIENTED_EDGE('',*,*,#14414,.F.);
#18931=ORIENTED_EDGE('',*,*,#14298,.T.);
#18932=ORIENTED_EDGE('',*,*,#14374,.F.);
#18933=ORIENTED_EDGE('',*,*,#13928,.T.);
#18934=ORIENTED_EDGE('',*,*,#14413,.F.);
#18935=ORIENTED_EDGE('',*,*,#14417,.T.);
#18936=ORIENTED_EDGE('',*,*,#14377,.F.);
#18937=ORIENTED_EDGE('',*,*,#14417,.F.);
#18938=ORIENTED_EDGE('',*,*,#14415,.F.);
#18939=ORIENTED_EDGE('',*,*,#14418,.F.);
#18940=ORIENTED_EDGE('',*,*,#14378,.F.);
#18941=ORIENTED_EDGE('',*,*,#14418,.T.);
#18942=ORIENTED_EDGE('',*,*,#14416,.F.);
#18943=ORIENTED_EDGE('',*,*,#14402,.T.);
#18944=ORIENTED_EDGE('',*,*,#14419,.F.);
#18945=ORIENTED_EDGE('',*,*,#14420,.F.);
#18946=ORIENTED_EDGE('',*,*,#14421,.F.);
#18947=ORIENTED_EDGE('',*,*,#14422,.F.);
#18948=ORIENTED_EDGE('',*,*,#14423,.F.);
#18949=ORIENTED_EDGE('',*,*,#14400,.T.);
#18950=ORIENTED_EDGE('',*,*,#14424,.F.);
#18951=ORIENTED_EDGE('',*,*,#14425,.F.);
#18952=ORIENTED_EDGE('',*,*,#14426,.F.);
#18953=ORIENTED_EDGE('',*,*,#14427,.F.);
#18954=ORIENTED_EDGE('',*,*,#14428,.F.);
#18955=ORIENTED_EDGE('',*,*,#14429,.F.);
#18956=ORIENTED_EDGE('',*,*,#14398,.T.);
#18957=ORIENTED_EDGE('',*,*,#14430,.T.);
#18958=ORIENTED_EDGE('',*,*,#14361,.T.);
#18959=ORIENTED_EDGE('',*,*,#14431,.F.);
#18960=ORIENTED_EDGE('',*,*,#14427,.T.);
#18961=ORIENTED_EDGE('',*,*,#14426,.T.);
#18962=ORIENTED_EDGE('',*,*,#14425,.T.);
#18963=ORIENTED_EDGE('',*,*,#14432,.T.);
#18964=ORIENTED_EDGE('',*,*,#14359,.T.);
#18965=ORIENTED_EDGE('',*,*,#14363,.T.);
#18966=ORIENTED_EDGE('',*,*,#14433,.T.);
#18967=ORIENTED_EDGE('',*,*,#14399,.T.);
#18968=ORIENTED_EDGE('',*,*,#14432,.F.);
#18969=ORIENTED_EDGE('',*,*,#14429,.T.);
#18970=ORIENTED_EDGE('',*,*,#14428,.T.);
#18971=ORIENTED_EDGE('',*,*,#14431,.T.);
#18972=ORIENTED_EDGE('',*,*,#14360,.T.);
#18973=ORIENTED_EDGE('',*,*,#14430,.F.);
#18974=ORIENTED_EDGE('',*,*,#14424,.T.);
#18975=ORIENTED_EDGE('',*,*,#14433,.F.);
#18976=ORIENTED_EDGE('',*,*,#14362,.T.);
#18977=ORIENTED_EDGE('',*,*,#14434,.T.);
#18978=ORIENTED_EDGE('',*,*,#14435,.T.);
#18979=ORIENTED_EDGE('',*,*,#14436,.T.);
#18980=ORIENTED_EDGE('',*,*,#14437,.T.);
#18981=ORIENTED_EDGE('',*,*,#14340,.T.);
#18982=ORIENTED_EDGE('',*,*,#14438,.T.);
#18983=ORIENTED_EDGE('',*,*,#14287,.T.);
#18984=ORIENTED_EDGE('',*,*,#14439,.T.);
#18985=ORIENTED_EDGE('',*,*,#14440,.T.);
#18986=ORIENTED_EDGE('',*,*,#14439,.F.);
#18987=ORIENTED_EDGE('',*,*,#14286,.T.);
#18988=ORIENTED_EDGE('',*,*,#14437,.F.);
#18989=ORIENTED_EDGE('',*,*,#14441,.T.);
#18990=ORIENTED_EDGE('',*,*,#14434,.F.);
#18991=ORIENTED_EDGE('',*,*,#14288,.T.);
#18992=ORIENTED_EDGE('',*,*,#14438,.F.);
#18993=ORIENTED_EDGE('',*,*,#14442,.T.);
#18994=ORIENTED_EDGE('',*,*,#14440,.F.);
#18995=ORIENTED_EDGE('',*,*,#14441,.F.);
#18996=ORIENTED_EDGE('',*,*,#14436,.F.);
#18997=ORIENTED_EDGE('',*,*,#14443,.T.);
#18998=ORIENTED_EDGE('',*,*,#14444,.F.);
#18999=ORIENTED_EDGE('',*,*,#14445,.F.);
#19000=ORIENTED_EDGE('',*,*,#14446,.F.);
#19001=ORIENTED_EDGE('',*,*,#14447,.F.);
#19002=ORIENTED_EDGE('',*,*,#14448,.F.);
#19003=ORIENTED_EDGE('',*,*,#14443,.F.);
#19004=ORIENTED_EDGE('',*,*,#14435,.F.);
#19005=ORIENTED_EDGE('',*,*,#14442,.F.);
#19006=ORIENTED_EDGE('',*,*,#14449,.T.);
#19007=ORIENTED_EDGE('',*,*,#14446,.T.);
#19008=ORIENTED_EDGE('',*,*,#14450,.F.);
#19009=ORIENTED_EDGE('',*,*,#14393,.T.);
#19010=ORIENTED_EDGE('',*,*,#14392,.T.);
#19011=ORIENTED_EDGE('',*,*,#14391,.T.);
#19012=ORIENTED_EDGE('',*,*,#14451,.T.);
#19013=ORIENTED_EDGE('',*,*,#14444,.T.);
#19014=ORIENTED_EDGE('',*,*,#14448,.T.);
#19015=ORIENTED_EDGE('',*,*,#14452,.T.);
#19016=ORIENTED_EDGE('',*,*,#14404,.T.);
#19017=ORIENTED_EDGE('',*,*,#14451,.F.);
#19018=ORIENTED_EDGE('',*,*,#14395,.T.);
#19019=ORIENTED_EDGE('',*,*,#14394,.T.);
#19020=ORIENTED_EDGE('',*,*,#14450,.T.);
#19021=ORIENTED_EDGE('',*,*,#14445,.T.);
#19022=ORIENTED_EDGE('',*,*,#14449,.F.);
#19023=ORIENTED_EDGE('',*,*,#14390,.T.);
#19024=ORIENTED_EDGE('',*,*,#14452,.F.);
#19025=ORIENTED_EDGE('',*,*,#14447,.T.);
#19026=ORIENTED_EDGE('',*,*,#14453,.T.);
#19027=ORIENTED_EDGE('',*,*,#14334,.T.);
#19028=ORIENTED_EDGE('',*,*,#14454,.T.);
#19029=ORIENTED_EDGE('',*,*,#14455,.T.);
#19030=ORIENTED_EDGE('',*,*,#14456,.T.);
#19031=ORIENTED_EDGE('',*,*,#14457,.T.);
#19032=ORIENTED_EDGE('',*,*,#14458,.T.);
#19033=ORIENTED_EDGE('',*,*,#14459,.T.);
#19034=ORIENTED_EDGE('',*,*,#14337,.T.);
#19035=ORIENTED_EDGE('',*,*,#14456,.F.);
#19036=ORIENTED_EDGE('',*,*,#14335,.T.);
#19037=ORIENTED_EDGE('',*,*,#14453,.F.);
#19038=ORIENTED_EDGE('',*,*,#14460,.T.);
#19039=ORIENTED_EDGE('',*,*,#14454,.F.);
#19040=ORIENTED_EDGE('',*,*,#14333,.T.);
#19041=ORIENTED_EDGE('',*,*,#14459,.F.);
#19042=ORIENTED_EDGE('',*,*,#14461,.T.);
#19043=ORIENTED_EDGE('',*,*,#14457,.F.);
#19044=ORIENTED_EDGE('',*,*,#14460,.F.);
#19045=ORIENTED_EDGE('',*,*,#14455,.F.);
#19046=ORIENTED_EDGE('',*,*,#14461,.F.);
#19047=ORIENTED_EDGE('',*,*,#14458,.F.);
#19048=ORIENTED_EDGE('',*,*,#14462,.T.);
#19049=ORIENTED_EDGE('',*,*,#14463,.F.);
#19050=ORIENTED_EDGE('',*,*,#14464,.F.);
#19051=ORIENTED_EDGE('',*,*,#14465,.F.);
#19052=ORIENTED_EDGE('',*,*,#14466,.F.);
#19053=ORIENTED_EDGE('',*,*,#14467,.F.);
#19054=ORIENTED_EDGE('',*,*,#14462,.F.);
#19055=ORIENTED_EDGE('',*,*,#14468,.T.);
#19056=ORIENTED_EDGE('',*,*,#14465,.T.);
#19057=ORIENTED_EDGE('',*,*,#14469,.F.);
#19058=ORIENTED_EDGE('',*,*,#14422,.T.);
#19059=ORIENTED_EDGE('',*,*,#14421,.T.);
#19060=ORIENTED_EDGE('',*,*,#14420,.T.);
#19061=ORIENTED_EDGE('',*,*,#14470,.T.);
#19062=ORIENTED_EDGE('',*,*,#14463,.T.);
#19063=ORIENTED_EDGE('',*,*,#14467,.T.);
#19064=ORIENTED_EDGE('',*,*,#14471,.T.);
#19065=ORIENTED_EDGE('',*,*,#14401,.T.);
#19066=ORIENTED_EDGE('',*,*,#14470,.F.);
#19067=ORIENTED_EDGE('',*,*,#14423,.T.);
#19068=ORIENTED_EDGE('',*,*,#14469,.T.);
#19069=ORIENTED_EDGE('',*,*,#14464,.T.);
#19070=ORIENTED_EDGE('',*,*,#14468,.F.);
#19071=ORIENTED_EDGE('',*,*,#14419,.T.);
#19072=ORIENTED_EDGE('',*,*,#14471,.F.);
#19073=ORIENTED_EDGE('',*,*,#14466,.T.);
#19074=ORIENTED_EDGE('',*,*,#14472,.T.);
#19075=ORIENTED_EDGE('',*,*,#14473,.T.);
#19076=ORIENTED_EDGE('',*,*,#14474,.T.);
#19077=ORIENTED_EDGE('',*,*,#14475,.T.);
#19078=ORIENTED_EDGE('',*,*,#14339,.T.);
#19079=ORIENTED_EDGE('',*,*,#14476,.T.);
#19080=ORIENTED_EDGE('',*,*,#14291,.T.);
#19081=ORIENTED_EDGE('',*,*,#14477,.T.);
#19082=ORIENTED_EDGE('',*,*,#14478,.T.);
#19083=ORIENTED_EDGE('',*,*,#14477,.F.);
#19084=ORIENTED_EDGE('',*,*,#14290,.T.);
#19085=ORIENTED_EDGE('',*,*,#14475,.F.);
#19086=ORIENTED_EDGE('',*,*,#14479,.T.);
#19087=ORIENTED_EDGE('',*,*,#14472,.F.);
#19088=ORIENTED_EDGE('',*,*,#14292,.T.);
#19089=ORIENTED_EDGE('',*,*,#14476,.F.);
#19090=ORIENTED_EDGE('',*,*,#14480,.T.);
#19091=ORIENTED_EDGE('',*,*,#14478,.F.);
#19092=ORIENTED_EDGE('',*,*,#14479,.F.);
#19093=ORIENTED_EDGE('',*,*,#14474,.F.);
#19094=ORIENTED_EDGE('',*,*,#14481,.T.);
#19095=ORIENTED_EDGE('',*,*,#14482,.F.);
#19096=ORIENTED_EDGE('',*,*,#14483,.F.);
#19097=ORIENTED_EDGE('',*,*,#14484,.F.);
#19098=ORIENTED_EDGE('',*,*,#14485,.F.);
#19099=ORIENTED_EDGE('',*,*,#14486,.F.);
#19100=ORIENTED_EDGE('',*,*,#14481,.F.);
#19101=ORIENTED_EDGE('',*,*,#14473,.F.);
#19102=ORIENTED_EDGE('',*,*,#14480,.F.);
#19103=ORIENTED_EDGE('',*,*,#14487,.T.);
#19104=ORIENTED_EDGE('',*,*,#14484,.T.);
#19105=ORIENTED_EDGE('',*,*,#14488,.F.);
#19106=ORIENTED_EDGE('',*,*,#14387,.T.);
#19107=ORIENTED_EDGE('',*,*,#14386,.T.);
#19108=ORIENTED_EDGE('',*,*,#14385,.T.);
#19109=ORIENTED_EDGE('',*,*,#14489,.T.);
#19110=ORIENTED_EDGE('',*,*,#14482,.T.);
#19111=ORIENTED_EDGE('',*,*,#14486,.T.);
#19112=ORIENTED_EDGE('',*,*,#14490,.T.);
#19113=ORIENTED_EDGE('',*,*,#14405,.T.);
#19114=ORIENTED_EDGE('',*,*,#14489,.F.);
#19115=ORIENTED_EDGE('',*,*,#14388,.T.);
#19116=ORIENTED_EDGE('',*,*,#14488,.T.);
#19117=ORIENTED_EDGE('',*,*,#14483,.T.);
#19118=ORIENTED_EDGE('',*,*,#14487,.F.);
#19119=ORIENTED_EDGE('',*,*,#14384,.T.);
#19120=ORIENTED_EDGE('',*,*,#14490,.F.);
#19121=ORIENTED_EDGE('',*,*,#14485,.T.);
#19122=ORIENTED_EDGE('',*,*,#14491,.T.);
#19123=ORIENTED_EDGE('',*,*,#14492,.T.);
#19124=ORIENTED_EDGE('',*,*,#14493,.T.);
#19125=ORIENTED_EDGE('',*,*,#14492,.F.);
#19126=ORIENTED_EDGE('',*,*,#14493,.F.);
#19127=ORIENTED_EDGE('',*,*,#14494,.T.);
#19128=ORIENTED_EDGE('',*,*,#14495,.F.);
#19129=ORIENTED_EDGE('',*,*,#14494,.F.);
#19130=ORIENTED_EDGE('',*,*,#13862,.F.);
#19131=ORIENTED_EDGE('',*,*,#13878,.F.);
#19132=ORIENTED_EDGE('',*,*,#13880,.F.);
#19133=ORIENTED_EDGE('',*,*,#13851,.F.);
#19134=ORIENTED_EDGE('',*,*,#14496,.F.);
#19135=ORIENTED_EDGE('',*,*,#14491,.F.);
#19136=ORIENTED_EDGE('',*,*,#14497,.T.);
#19137=ORIENTED_EDGE('',*,*,#14498,.T.);
#19138=ORIENTED_EDGE('',*,*,#14495,.T.);
#19139=ORIENTED_EDGE('',*,*,#14498,.F.);
#19140=ORIENTED_EDGE('',*,*,#14009,.F.);
#19141=ORIENTED_EDGE('',*,*,#13865,.T.);
#19142=ORIENTED_EDGE('',*,*,#14280,.F.);
#19143=ORIENTED_EDGE('',*,*,#14499,.T.);
#19144=ORIENTED_EDGE('',*,*,#14500,.F.);
#19145=ORIENTED_EDGE('',*,*,#14497,.F.);
#19146=ORIENTED_EDGE('',*,*,#14496,.T.);
#19147=ORIENTED_EDGE('',*,*,#14501,.T.);
#19148=ORIENTED_EDGE('',*,*,#14502,.T.);
#19149=ORIENTED_EDGE('',*,*,#14501,.F.);
#19150=ORIENTED_EDGE('',*,*,#14502,.F.);
#19151=ORIENTED_EDGE('',*,*,#14503,.T.);
#19152=ORIENTED_EDGE('',*,*,#14504,.F.);
#19153=ORIENTED_EDGE('',*,*,#14503,.F.);
#19154=ORIENTED_EDGE('',*,*,#14500,.T.);
#19155=ORIENTED_EDGE('',*,*,#14505,.T.);
#19156=ORIENTED_EDGE('',*,*,#14504,.T.);
#19157=ORIENTED_EDGE('',*,*,#14505,.F.);
#19158=ORIENTED_EDGE('',*,*,#14506,.F.);
#19159=ORIENTED_EDGE('',*,*,#14507,.T.);
#19160=ORIENTED_EDGE('',*,*,#14508,.T.);
#19161=ORIENTED_EDGE('',*,*,#14509,.F.);
#19162=ORIENTED_EDGE('',*,*,#14510,.F.);
#19163=ORIENTED_EDGE('',*,*,#14511,.T.);
#19164=ORIENTED_EDGE('',*,*,#14512,.T.);
#19165=ORIENTED_EDGE('',*,*,#14507,.F.);
#19166=ORIENTED_EDGE('',*,*,#14513,.F.);
#19167=ORIENTED_EDGE('',*,*,#14514,.T.);
#19168=ORIENTED_EDGE('',*,*,#14515,.T.);
#19169=ORIENTED_EDGE('',*,*,#14511,.F.);
#19170=ORIENTED_EDGE('',*,*,#14516,.F.);
#19171=ORIENTED_EDGE('',*,*,#14517,.T.);
#19172=ORIENTED_EDGE('',*,*,#14518,.T.);
#19173=ORIENTED_EDGE('',*,*,#14514,.F.);
#19174=ORIENTED_EDGE('',*,*,#14519,.F.);
#19175=ORIENTED_EDGE('',*,*,#14520,.T.);
#19176=ORIENTED_EDGE('',*,*,#14521,.T.);
#19177=ORIENTED_EDGE('',*,*,#14517,.F.);
#19178=ORIENTED_EDGE('',*,*,#14522,.F.);
#19179=ORIENTED_EDGE('',*,*,#14523,.T.);
#19180=ORIENTED_EDGE('',*,*,#14524,.T.);
#19181=ORIENTED_EDGE('',*,*,#14520,.F.);
#19182=ORIENTED_EDGE('',*,*,#14525,.F.);
#19183=ORIENTED_EDGE('',*,*,#14526,.T.);
#19184=ORIENTED_EDGE('',*,*,#14527,.T.);
#19185=ORIENTED_EDGE('',*,*,#14523,.F.);
#19186=ORIENTED_EDGE('',*,*,#14528,.F.);
#19187=ORIENTED_EDGE('',*,*,#14509,.T.);
#19188=ORIENTED_EDGE('',*,*,#14529,.T.);
#19189=ORIENTED_EDGE('',*,*,#14526,.F.);
#19190=ORIENTED_EDGE('',*,*,#14056,.F.);
#19191=ORIENTED_EDGE('',*,*,#14530,.T.);
#19192=ORIENTED_EDGE('',*,*,#14531,.T.);
#19193=ORIENTED_EDGE('',*,*,#14532,.F.);
#19194=ORIENTED_EDGE('',*,*,#14065,.F.);
#19195=ORIENTED_EDGE('',*,*,#14533,.T.);
#19196=ORIENTED_EDGE('',*,*,#14534,.T.);
#19197=ORIENTED_EDGE('',*,*,#14530,.F.);
#19198=ORIENTED_EDGE('',*,*,#14064,.F.);
#19199=ORIENTED_EDGE('',*,*,#14535,.T.);
#19200=ORIENTED_EDGE('',*,*,#14536,.T.);
#19201=ORIENTED_EDGE('',*,*,#14533,.F.);
#19202=ORIENTED_EDGE('',*,*,#14063,.F.);
#19203=ORIENTED_EDGE('',*,*,#14537,.T.);
#19204=ORIENTED_EDGE('',*,*,#14538,.T.);
#19205=ORIENTED_EDGE('',*,*,#14535,.F.);
#19206=ORIENTED_EDGE('',*,*,#14062,.F.);
#19207=ORIENTED_EDGE('',*,*,#14539,.T.);
#19208=ORIENTED_EDGE('',*,*,#14540,.T.);
#19209=ORIENTED_EDGE('',*,*,#14537,.F.);
#19210=ORIENTED_EDGE('',*,*,#14061,.F.);
#19211=ORIENTED_EDGE('',*,*,#14541,.T.);
#19212=ORIENTED_EDGE('',*,*,#14542,.T.);
#19213=ORIENTED_EDGE('',*,*,#14539,.F.);
#19214=ORIENTED_EDGE('',*,*,#14060,.F.);
#19215=ORIENTED_EDGE('',*,*,#14543,.T.);
#19216=ORIENTED_EDGE('',*,*,#14544,.T.);
#19217=ORIENTED_EDGE('',*,*,#14541,.F.);
#19218=ORIENTED_EDGE('',*,*,#14059,.F.);
#19219=ORIENTED_EDGE('',*,*,#14545,.T.);
#19220=ORIENTED_EDGE('',*,*,#14546,.T.);
#19221=ORIENTED_EDGE('',*,*,#14543,.F.);
#19222=ORIENTED_EDGE('',*,*,#14058,.F.);
#19223=ORIENTED_EDGE('',*,*,#14547,.T.);
#19224=ORIENTED_EDGE('',*,*,#14548,.T.);
#19225=ORIENTED_EDGE('',*,*,#14545,.F.);
#19226=ORIENTED_EDGE('',*,*,#14057,.F.);
#19227=ORIENTED_EDGE('',*,*,#14532,.T.);
#19228=ORIENTED_EDGE('',*,*,#14549,.T.);
#19229=ORIENTED_EDGE('',*,*,#14547,.F.);
#19230=ORIENTED_EDGE('',*,*,#14549,.F.);
#19231=ORIENTED_EDGE('',*,*,#14531,.F.);
#19232=ORIENTED_EDGE('',*,*,#14534,.F.);
#19233=ORIENTED_EDGE('',*,*,#14536,.F.);
#19234=ORIENTED_EDGE('',*,*,#14538,.F.);
#19235=ORIENTED_EDGE('',*,*,#14540,.F.);
#19236=ORIENTED_EDGE('',*,*,#14542,.F.);
#19237=ORIENTED_EDGE('',*,*,#14544,.F.);
#19238=ORIENTED_EDGE('',*,*,#14546,.F.);
#19239=ORIENTED_EDGE('',*,*,#14548,.F.);
#19240=ORIENTED_EDGE('',*,*,#14529,.F.);
#19241=ORIENTED_EDGE('',*,*,#14508,.F.);
#19242=ORIENTED_EDGE('',*,*,#14512,.F.);
#19243=ORIENTED_EDGE('',*,*,#14515,.F.);
#19244=ORIENTED_EDGE('',*,*,#14518,.F.);
#19245=ORIENTED_EDGE('',*,*,#14521,.F.);
#19246=ORIENTED_EDGE('',*,*,#14524,.F.);
#19247=ORIENTED_EDGE('',*,*,#14527,.F.);
#19248=ORIENTED_EDGE('',*,*,#14066,.F.);
#19249=ORIENTED_EDGE('',*,*,#14550,.T.);
#19250=ORIENTED_EDGE('',*,*,#14551,.T.);
#19251=ORIENTED_EDGE('',*,*,#14552,.F.);
#19252=ORIENTED_EDGE('',*,*,#14073,.F.);
#19253=ORIENTED_EDGE('',*,*,#14553,.T.);
#19254=ORIENTED_EDGE('',*,*,#14554,.T.);
#19255=ORIENTED_EDGE('',*,*,#14550,.F.);
#19256=ORIENTED_EDGE('',*,*,#14072,.F.);
#19257=ORIENTED_EDGE('',*,*,#14555,.T.);
#19258=ORIENTED_EDGE('',*,*,#14556,.T.);
#19259=ORIENTED_EDGE('',*,*,#14553,.F.);
#19260=ORIENTED_EDGE('',*,*,#14071,.F.);
#19261=ORIENTED_EDGE('',*,*,#14557,.T.);
#19262=ORIENTED_EDGE('',*,*,#14558,.T.);
#19263=ORIENTED_EDGE('',*,*,#14555,.F.);
#19264=ORIENTED_EDGE('',*,*,#14070,.F.);
#19265=ORIENTED_EDGE('',*,*,#14559,.T.);
#19266=ORIENTED_EDGE('',*,*,#14560,.T.);
#19267=ORIENTED_EDGE('',*,*,#14557,.F.);
#19268=ORIENTED_EDGE('',*,*,#14069,.F.);
#19269=ORIENTED_EDGE('',*,*,#14561,.T.);
#19270=ORIENTED_EDGE('',*,*,#14562,.T.);
#19271=ORIENTED_EDGE('',*,*,#14559,.F.);
#19272=ORIENTED_EDGE('',*,*,#14068,.F.);
#19273=ORIENTED_EDGE('',*,*,#14563,.T.);
#19274=ORIENTED_EDGE('',*,*,#14564,.T.);
#19275=ORIENTED_EDGE('',*,*,#14561,.F.);
#19276=ORIENTED_EDGE('',*,*,#14067,.F.);
#19277=ORIENTED_EDGE('',*,*,#14552,.T.);
#19278=ORIENTED_EDGE('',*,*,#14565,.T.);
#19279=ORIENTED_EDGE('',*,*,#14563,.F.);
#19280=ORIENTED_EDGE('',*,*,#14565,.F.);
#19281=ORIENTED_EDGE('',*,*,#14551,.F.);
#19282=ORIENTED_EDGE('',*,*,#14554,.F.);
#19283=ORIENTED_EDGE('',*,*,#14556,.F.);
#19284=ORIENTED_EDGE('',*,*,#14558,.F.);
#19285=ORIENTED_EDGE('',*,*,#14560,.F.);
#19286=ORIENTED_EDGE('',*,*,#14562,.F.);
#19287=ORIENTED_EDGE('',*,*,#14564,.F.);
#19288=ORIENTED_EDGE('',*,*,#14566,.F.);
#19289=ORIENTED_EDGE('',*,*,#14567,.T.);
#19290=ORIENTED_EDGE('',*,*,#14568,.T.);
#19291=ORIENTED_EDGE('',*,*,#14569,.F.);
#19292=ORIENTED_EDGE('',*,*,#14570,.F.);
#19293=ORIENTED_EDGE('',*,*,#14571,.T.);
#19294=ORIENTED_EDGE('',*,*,#14572,.T.);
#19295=ORIENTED_EDGE('',*,*,#14567,.F.);
#19296=ORIENTED_EDGE('',*,*,#14573,.F.);
#19297=ORIENTED_EDGE('',*,*,#14574,.T.);
#19298=ORIENTED_EDGE('',*,*,#14575,.T.);
#19299=ORIENTED_EDGE('',*,*,#14571,.F.);
#19300=ORIENTED_EDGE('',*,*,#14576,.F.);
#19301=ORIENTED_EDGE('',*,*,#14577,.T.);
#19302=ORIENTED_EDGE('',*,*,#14578,.T.);
#19303=ORIENTED_EDGE('',*,*,#14574,.F.);
#19304=ORIENTED_EDGE('',*,*,#14579,.F.);
#19305=ORIENTED_EDGE('',*,*,#14580,.T.);
#19306=ORIENTED_EDGE('',*,*,#14581,.T.);
#19307=ORIENTED_EDGE('',*,*,#14577,.F.);
#19308=ORIENTED_EDGE('',*,*,#14582,.F.);
#19309=ORIENTED_EDGE('',*,*,#14583,.T.);
#19310=ORIENTED_EDGE('',*,*,#14584,.T.);
#19311=ORIENTED_EDGE('',*,*,#14580,.F.);
#19312=ORIENTED_EDGE('',*,*,#14585,.F.);
#19313=ORIENTED_EDGE('',*,*,#14586,.T.);
#19314=ORIENTED_EDGE('',*,*,#14587,.T.);
#19315=ORIENTED_EDGE('',*,*,#14583,.F.);
#19316=ORIENTED_EDGE('',*,*,#14588,.F.);
#19317=ORIENTED_EDGE('',*,*,#14589,.T.);
#19318=ORIENTED_EDGE('',*,*,#14590,.T.);
#19319=ORIENTED_EDGE('',*,*,#14586,.F.);
#19320=ORIENTED_EDGE('',*,*,#14591,.F.);
#19321=ORIENTED_EDGE('',*,*,#14569,.T.);
#19322=ORIENTED_EDGE('',*,*,#14592,.T.);
#19323=ORIENTED_EDGE('',*,*,#14589,.F.);
#19324=ORIENTED_EDGE('',*,*,#14074,.F.);
#19325=ORIENTED_EDGE('',*,*,#14593,.T.);
#19326=ORIENTED_EDGE('',*,*,#14594,.T.);
#19327=ORIENTED_EDGE('',*,*,#14595,.F.);
#19328=ORIENTED_EDGE('',*,*,#14086,.F.);
#19329=ORIENTED_EDGE('',*,*,#14596,.T.);
#19330=ORIENTED_EDGE('',*,*,#14597,.T.);
#19331=ORIENTED_EDGE('',*,*,#14593,.F.);
#19332=ORIENTED_EDGE('',*,*,#14085,.F.);
#19333=ORIENTED_EDGE('',*,*,#14598,.T.);
#19334=ORIENTED_EDGE('',*,*,#14599,.T.);
#19335=ORIENTED_EDGE('',*,*,#14596,.F.);
#19336=ORIENTED_EDGE('',*,*,#14084,.F.);
#19337=ORIENTED_EDGE('',*,*,#14600,.T.);
#19338=ORIENTED_EDGE('',*,*,#14601,.T.);
#19339=ORIENTED_EDGE('',*,*,#14598,.F.);
#19340=ORIENTED_EDGE('',*,*,#14083,.F.);
#19341=ORIENTED_EDGE('',*,*,#14602,.T.);
#19342=ORIENTED_EDGE('',*,*,#14603,.T.);
#19343=ORIENTED_EDGE('',*,*,#14600,.F.);
#19344=ORIENTED_EDGE('',*,*,#14082,.F.);
#19345=ORIENTED_EDGE('',*,*,#14604,.T.);
#19346=ORIENTED_EDGE('',*,*,#14605,.T.);
#19347=ORIENTED_EDGE('',*,*,#14602,.F.);
#19348=ORIENTED_EDGE('',*,*,#14081,.F.);
#19349=ORIENTED_EDGE('',*,*,#14606,.T.);
#19350=ORIENTED_EDGE('',*,*,#14607,.T.);
#19351=ORIENTED_EDGE('',*,*,#14604,.F.);
#19352=ORIENTED_EDGE('',*,*,#14080,.F.);
#19353=ORIENTED_EDGE('',*,*,#14608,.T.);
#19354=ORIENTED_EDGE('',*,*,#14609,.T.);
#19355=ORIENTED_EDGE('',*,*,#14606,.F.);
#19356=ORIENTED_EDGE('',*,*,#14079,.F.);
#19357=ORIENTED_EDGE('',*,*,#14610,.T.);
#19358=ORIENTED_EDGE('',*,*,#14611,.T.);
#19359=ORIENTED_EDGE('',*,*,#14608,.F.);
#19360=ORIENTED_EDGE('',*,*,#14078,.F.);
#19361=ORIENTED_EDGE('',*,*,#14612,.T.);
#19362=ORIENTED_EDGE('',*,*,#14613,.T.);
#19363=ORIENTED_EDGE('',*,*,#14610,.F.);
#19364=ORIENTED_EDGE('',*,*,#14077,.F.);
#19365=ORIENTED_EDGE('',*,*,#14614,.T.);
#19366=ORIENTED_EDGE('',*,*,#14615,.T.);
#19367=ORIENTED_EDGE('',*,*,#14612,.F.);
#19368=ORIENTED_EDGE('',*,*,#14076,.F.);
#19369=ORIENTED_EDGE('',*,*,#14616,.T.);
#19370=ORIENTED_EDGE('',*,*,#14617,.T.);
#19371=ORIENTED_EDGE('',*,*,#14614,.F.);
#19372=ORIENTED_EDGE('',*,*,#14075,.F.);
#19373=ORIENTED_EDGE('',*,*,#14595,.T.);
#19374=ORIENTED_EDGE('',*,*,#14618,.T.);
#19375=ORIENTED_EDGE('',*,*,#14616,.F.);
#19376=ORIENTED_EDGE('',*,*,#14618,.F.);
#19377=ORIENTED_EDGE('',*,*,#14594,.F.);
#19378=ORIENTED_EDGE('',*,*,#14597,.F.);
#19379=ORIENTED_EDGE('',*,*,#14599,.F.);
#19380=ORIENTED_EDGE('',*,*,#14601,.F.);
#19381=ORIENTED_EDGE('',*,*,#14603,.F.);
#19382=ORIENTED_EDGE('',*,*,#14605,.F.);
#19383=ORIENTED_EDGE('',*,*,#14607,.F.);
#19384=ORIENTED_EDGE('',*,*,#14609,.F.);
#19385=ORIENTED_EDGE('',*,*,#14611,.F.);
#19386=ORIENTED_EDGE('',*,*,#14613,.F.);
#19387=ORIENTED_EDGE('',*,*,#14615,.F.);
#19388=ORIENTED_EDGE('',*,*,#14617,.F.);
#19389=ORIENTED_EDGE('',*,*,#14592,.F.);
#19390=ORIENTED_EDGE('',*,*,#14568,.F.);
#19391=ORIENTED_EDGE('',*,*,#14572,.F.);
#19392=ORIENTED_EDGE('',*,*,#14575,.F.);
#19393=ORIENTED_EDGE('',*,*,#14578,.F.);
#19394=ORIENTED_EDGE('',*,*,#14581,.F.);
#19395=ORIENTED_EDGE('',*,*,#14584,.F.);
#19396=ORIENTED_EDGE('',*,*,#14587,.F.);
#19397=ORIENTED_EDGE('',*,*,#14590,.F.);
#19398=ORIENTED_EDGE('',*,*,#14087,.F.);
#19399=ORIENTED_EDGE('',*,*,#14619,.T.);
#19400=ORIENTED_EDGE('',*,*,#14620,.T.);
#19401=ORIENTED_EDGE('',*,*,#14621,.F.);
#19402=ORIENTED_EDGE('',*,*,#14108,.F.);
#19403=ORIENTED_EDGE('',*,*,#14622,.T.);
#19404=ORIENTED_EDGE('',*,*,#14623,.T.);
#19405=ORIENTED_EDGE('',*,*,#14619,.F.);
#19406=ORIENTED_EDGE('',*,*,#14107,.F.);
#19407=ORIENTED_EDGE('',*,*,#14624,.T.);
#19408=ORIENTED_EDGE('',*,*,#14625,.T.);
#19409=ORIENTED_EDGE('',*,*,#14622,.F.);
#19410=ORIENTED_EDGE('',*,*,#14106,.F.);
#19411=ORIENTED_EDGE('',*,*,#14626,.T.);
#19412=ORIENTED_EDGE('',*,*,#14627,.T.);
#19413=ORIENTED_EDGE('',*,*,#14624,.F.);
#19414=ORIENTED_EDGE('',*,*,#14105,.F.);
#19415=ORIENTED_EDGE('',*,*,#14628,.T.);
#19416=ORIENTED_EDGE('',*,*,#14629,.T.);
#19417=ORIENTED_EDGE('',*,*,#14626,.F.);
#19418=ORIENTED_EDGE('',*,*,#14104,.F.);
#19419=ORIENTED_EDGE('',*,*,#14630,.T.);
#19420=ORIENTED_EDGE('',*,*,#14631,.T.);
#19421=ORIENTED_EDGE('',*,*,#14628,.F.);
#19422=ORIENTED_EDGE('',*,*,#14103,.F.);
#19423=ORIENTED_EDGE('',*,*,#14632,.T.);
#19424=ORIENTED_EDGE('',*,*,#14633,.T.);
#19425=ORIENTED_EDGE('',*,*,#14630,.F.);
#19426=ORIENTED_EDGE('',*,*,#14102,.F.);
#19427=ORIENTED_EDGE('',*,*,#14634,.T.);
#19428=ORIENTED_EDGE('',*,*,#14635,.T.);
#19429=ORIENTED_EDGE('',*,*,#14632,.F.);
#19430=ORIENTED_EDGE('',*,*,#14101,.F.);
#19431=ORIENTED_EDGE('',*,*,#14636,.T.);
#19432=ORIENTED_EDGE('',*,*,#14637,.T.);
#19433=ORIENTED_EDGE('',*,*,#14634,.F.);
#19434=ORIENTED_EDGE('',*,*,#14100,.F.);
#19435=ORIENTED_EDGE('',*,*,#14638,.T.);
#19436=ORIENTED_EDGE('',*,*,#14639,.T.);
#19437=ORIENTED_EDGE('',*,*,#14636,.F.);
#19438=ORIENTED_EDGE('',*,*,#14099,.F.);
#19439=ORIENTED_EDGE('',*,*,#14640,.T.);
#19440=ORIENTED_EDGE('',*,*,#14641,.T.);
#19441=ORIENTED_EDGE('',*,*,#14638,.F.);
#19442=ORIENTED_EDGE('',*,*,#14098,.F.);
#19443=ORIENTED_EDGE('',*,*,#14642,.T.);
#19444=ORIENTED_EDGE('',*,*,#14643,.T.);
#19445=ORIENTED_EDGE('',*,*,#14640,.F.);
#19446=ORIENTED_EDGE('',*,*,#14097,.F.);
#19447=ORIENTED_EDGE('',*,*,#14644,.T.);
#19448=ORIENTED_EDGE('',*,*,#14645,.T.);
#19449=ORIENTED_EDGE('',*,*,#14642,.F.);
#19450=ORIENTED_EDGE('',*,*,#14096,.F.);
#19451=ORIENTED_EDGE('',*,*,#14646,.T.);
#19452=ORIENTED_EDGE('',*,*,#14647,.T.);
#19453=ORIENTED_EDGE('',*,*,#14644,.F.);
#19454=ORIENTED_EDGE('',*,*,#14095,.F.);
#19455=ORIENTED_EDGE('',*,*,#14648,.T.);
#19456=ORIENTED_EDGE('',*,*,#14649,.T.);
#19457=ORIENTED_EDGE('',*,*,#14646,.F.);
#19458=ORIENTED_EDGE('',*,*,#14094,.F.);
#19459=ORIENTED_EDGE('',*,*,#14650,.T.);
#19460=ORIENTED_EDGE('',*,*,#14651,.T.);
#19461=ORIENTED_EDGE('',*,*,#14648,.F.);
#19462=ORIENTED_EDGE('',*,*,#14093,.F.);
#19463=ORIENTED_EDGE('',*,*,#14652,.T.);
#19464=ORIENTED_EDGE('',*,*,#14653,.T.);
#19465=ORIENTED_EDGE('',*,*,#14650,.F.);
#19466=ORIENTED_EDGE('',*,*,#14092,.F.);
#19467=ORIENTED_EDGE('',*,*,#14654,.T.);
#19468=ORIENTED_EDGE('',*,*,#14655,.T.);
#19469=ORIENTED_EDGE('',*,*,#14652,.F.);
#19470=ORIENTED_EDGE('',*,*,#14091,.F.);
#19471=ORIENTED_EDGE('',*,*,#14656,.T.);
#19472=ORIENTED_EDGE('',*,*,#14657,.T.);
#19473=ORIENTED_EDGE('',*,*,#14654,.F.);
#19474=ORIENTED_EDGE('',*,*,#14090,.F.);
#19475=ORIENTED_EDGE('',*,*,#14658,.T.);
#19476=ORIENTED_EDGE('',*,*,#14659,.T.);
#19477=ORIENTED_EDGE('',*,*,#14656,.F.);
#19478=ORIENTED_EDGE('',*,*,#14089,.F.);
#19479=ORIENTED_EDGE('',*,*,#14660,.T.);
#19480=ORIENTED_EDGE('',*,*,#14661,.T.);
#19481=ORIENTED_EDGE('',*,*,#14658,.F.);
#19482=ORIENTED_EDGE('',*,*,#14088,.F.);
#19483=ORIENTED_EDGE('',*,*,#14621,.T.);
#19484=ORIENTED_EDGE('',*,*,#14662,.T.);
#19485=ORIENTED_EDGE('',*,*,#14660,.F.);
#19486=ORIENTED_EDGE('',*,*,#14662,.F.);
#19487=ORIENTED_EDGE('',*,*,#14620,.F.);
#19488=ORIENTED_EDGE('',*,*,#14623,.F.);
#19489=ORIENTED_EDGE('',*,*,#14625,.F.);
#19490=ORIENTED_EDGE('',*,*,#14627,.F.);
#19491=ORIENTED_EDGE('',*,*,#14629,.F.);
#19492=ORIENTED_EDGE('',*,*,#14631,.F.);
#19493=ORIENTED_EDGE('',*,*,#14633,.F.);
#19494=ORIENTED_EDGE('',*,*,#14635,.F.);
#19495=ORIENTED_EDGE('',*,*,#14637,.F.);
#19496=ORIENTED_EDGE('',*,*,#14639,.F.);
#19497=ORIENTED_EDGE('',*,*,#14641,.F.);
#19498=ORIENTED_EDGE('',*,*,#14643,.F.);
#19499=ORIENTED_EDGE('',*,*,#14645,.F.);
#19500=ORIENTED_EDGE('',*,*,#14647,.F.);
#19501=ORIENTED_EDGE('',*,*,#14649,.F.);
#19502=ORIENTED_EDGE('',*,*,#14651,.F.);
#19503=ORIENTED_EDGE('',*,*,#14653,.F.);
#19504=ORIENTED_EDGE('',*,*,#14655,.F.);
#19505=ORIENTED_EDGE('',*,*,#14657,.F.);
#19506=ORIENTED_EDGE('',*,*,#14659,.F.);
#19507=ORIENTED_EDGE('',*,*,#14661,.F.);
#19508=ORIENTED_EDGE('',*,*,#14109,.F.);
#19509=ORIENTED_EDGE('',*,*,#14663,.T.);
#19510=ORIENTED_EDGE('',*,*,#14664,.T.);
#19511=ORIENTED_EDGE('',*,*,#14665,.F.);
#19512=ORIENTED_EDGE('',*,*,#14118,.F.);
#19513=ORIENTED_EDGE('',*,*,#14666,.T.);
#19514=ORIENTED_EDGE('',*,*,#14667,.T.);
#19515=ORIENTED_EDGE('',*,*,#14663,.F.);
#19516=ORIENTED_EDGE('',*,*,#14117,.F.);
#19517=ORIENTED_EDGE('',*,*,#14668,.T.);
#19518=ORIENTED_EDGE('',*,*,#14669,.T.);
#19519=ORIENTED_EDGE('',*,*,#14666,.F.);
#19520=ORIENTED_EDGE('',*,*,#14116,.F.);
#19521=ORIENTED_EDGE('',*,*,#14670,.T.);
#19522=ORIENTED_EDGE('',*,*,#14671,.T.);
#19523=ORIENTED_EDGE('',*,*,#14668,.F.);
#19524=ORIENTED_EDGE('',*,*,#14115,.F.);
#19525=ORIENTED_EDGE('',*,*,#14672,.T.);
#19526=ORIENTED_EDGE('',*,*,#14673,.T.);
#19527=ORIENTED_EDGE('',*,*,#14670,.F.);
#19528=ORIENTED_EDGE('',*,*,#14114,.F.);
#19529=ORIENTED_EDGE('',*,*,#14674,.T.);
#19530=ORIENTED_EDGE('',*,*,#14675,.T.);
#19531=ORIENTED_EDGE('',*,*,#14672,.F.);
#19532=ORIENTED_EDGE('',*,*,#14113,.F.);
#19533=ORIENTED_EDGE('',*,*,#14676,.T.);
#19534=ORIENTED_EDGE('',*,*,#14677,.T.);
#19535=ORIENTED_EDGE('',*,*,#14674,.F.);
#19536=ORIENTED_EDGE('',*,*,#14112,.F.);
#19537=ORIENTED_EDGE('',*,*,#14678,.T.);
#19538=ORIENTED_EDGE('',*,*,#14679,.T.);
#19539=ORIENTED_EDGE('',*,*,#14676,.F.);
#19540=ORIENTED_EDGE('',*,*,#14111,.F.);
#19541=ORIENTED_EDGE('',*,*,#14680,.T.);
#19542=ORIENTED_EDGE('',*,*,#14681,.T.);
#19543=ORIENTED_EDGE('',*,*,#14678,.F.);
#19544=ORIENTED_EDGE('',*,*,#14110,.F.);
#19545=ORIENTED_EDGE('',*,*,#14665,.T.);
#19546=ORIENTED_EDGE('',*,*,#14682,.T.);
#19547=ORIENTED_EDGE('',*,*,#14680,.F.);
#19548=ORIENTED_EDGE('',*,*,#14682,.F.);
#19549=ORIENTED_EDGE('',*,*,#14664,.F.);
#19550=ORIENTED_EDGE('',*,*,#14667,.F.);
#19551=ORIENTED_EDGE('',*,*,#14669,.F.);
#19552=ORIENTED_EDGE('',*,*,#14671,.F.);
#19553=ORIENTED_EDGE('',*,*,#14673,.F.);
#19554=ORIENTED_EDGE('',*,*,#14675,.F.);
#19555=ORIENTED_EDGE('',*,*,#14677,.F.);
#19556=ORIENTED_EDGE('',*,*,#14679,.F.);
#19557=ORIENTED_EDGE('',*,*,#14681,.F.);
#19558=ORIENTED_EDGE('',*,*,#14566,.T.);
#19559=ORIENTED_EDGE('',*,*,#14591,.T.);
#19560=ORIENTED_EDGE('',*,*,#14588,.T.);
#19561=ORIENTED_EDGE('',*,*,#14585,.T.);
#19562=ORIENTED_EDGE('',*,*,#14582,.T.);
#19563=ORIENTED_EDGE('',*,*,#14579,.T.);
#19564=ORIENTED_EDGE('',*,*,#14576,.T.);
#19565=ORIENTED_EDGE('',*,*,#14573,.T.);
#19566=ORIENTED_EDGE('',*,*,#14570,.T.);
#19567=ORIENTED_EDGE('',*,*,#14506,.T.);
#19568=ORIENTED_EDGE('',*,*,#14528,.T.);
#19569=ORIENTED_EDGE('',*,*,#14525,.T.);
#19570=ORIENTED_EDGE('',*,*,#14522,.T.);
#19571=ORIENTED_EDGE('',*,*,#14519,.T.);
#19572=ORIENTED_EDGE('',*,*,#14516,.T.);
#19573=ORIENTED_EDGE('',*,*,#14513,.T.);
#19574=ORIENTED_EDGE('',*,*,#14510,.T.);
#19575=ORIENTED_EDGE('',*,*,#13855,.F.);
#19576=ORIENTED_EDGE('',*,*,#14683,.T.);
#19577=ORIENTED_EDGE('',*,*,#14296,.F.);
#19578=ORIENTED_EDGE('',*,*,#13863,.T.);
#19579=ORIENTED_EDGE('',*,*,#13847,.F.);
#19580=ORIENTED_EDGE('',*,*,#13881,.F.);
#19581=ORIENTED_EDGE('',*,*,#13870,.F.);
#19582=ORIENTED_EDGE('',*,*,#13885,.F.);
#19583=ORIENTED_EDGE('',*,*,#14684,.F.);
#19584=ORIENTED_EDGE('',*,*,#14499,.F.);
#19585=ORIENTED_EDGE('',*,*,#14284,.F.);
#19586=ORIENTED_EDGE('',*,*,#14683,.F.);
#19587=ORIENTED_EDGE('',*,*,#14310,.F.);
#19588=ORIENTED_EDGE('',*,*,#14281,.F.);
#19589=ORIENTED_EDGE('',*,*,#13864,.T.);
#19590=ORIENTED_EDGE('',*,*,#14295,.F.);
#19591=ORIENTED_EDGE('',*,*,#14270,.F.);
#19592=ORIENTED_EDGE('',*,*,#13979,.T.);
#19593=ORIENTED_EDGE('',*,*,#14316,.F.);
#19594=ORIENTED_EDGE('',*,*,#14326,.T.);
#19595=ORIENTED_EDGE('',*,*,#14037,.F.);
#19596=ORIENTED_EDGE('',*,*,#14010,.F.);
#19597=ORIENTED_EDGE('',*,*,#14684,.T.);
#19598=ORIENTED_EDGE('',*,*,#14023,.F.);
#19599=ORIENTED_EDGE('',*,*,#13999,.F.);
#19600=ORIENTED_EDGE('',*,*,#13915,.T.);
#19601=ORIENTED_EDGE('',*,*,#14043,.F.);
#19602=ORIENTED_EDGE('',*,*,#14052,.T.);
#26071=PLANE('',#28690);
#26072=PLANE('',#28691);
#26073=PLANE('',#28692);
#26074=PLANE('',#28693);
#26075=PLANE('',#28694);
#26076=PLANE('',#28695);
#26077=PLANE('',#28696);
#26078=PLANE('',#28697);
#26079=PLANE('',#28698);
#26080=PLANE('',#28699);
#26081=PLANE('',#28700);
#26082=PLANE('',#28701);
#26083=PLANE('',#28702);
#26084=PLANE('',#28703);
#26085=PLANE('',#28707);
#26086=PLANE('',#28727);
#26087=PLANE('',#28737);
#26088=PLANE('',#28767);
#26089=PLANE('',#28777);
#26090=PLANE('',#28780);
#26091=PLANE('',#28784);
#26092=PLANE('',#28788);
#26093=PLANE('',#28791);
#26094=PLANE('',#28794);
#26095=PLANE('',#28801);
#26096=PLANE('',#28804);
#26097=PLANE('',#28808);
#26098=PLANE('',#28811);
#26099=PLANE('',#28812);
#26100=PLANE('',#28813);
#26101=PLANE('',#28817);
#26102=PLANE('',#28834);
#26103=PLANE('',#28837);
#26104=PLANE('',#28840);
#26105=PLANE('',#28843);
#26106=PLANE('',#28848);
#26107=PLANE('',#28851);
#26108=PLANE('',#28857);
#26109=PLANE('',#28860);
#26110=PLANE('',#28863);
#26111=PLANE('',#28865);
#26112=PLANE('',#28868);
#26113=PLANE('',#28882);
#26114=PLANE('',#28886);
#26115=PLANE('',#28890);
#26116=PLANE('',#28894);
#26117=PLANE('',#28897);
#26118=PLANE('',#28900);
#26119=PLANE('',#28907);
#26120=PLANE('',#28910);
#26121=PLANE('',#28914);
#26122=PLANE('',#28918);
#26123=PLANE('',#28919);
#26124=PLANE('',#28921);
#26125=PLANE('',#28926);
#26126=PLANE('',#28937);
#26127=PLANE('',#28940);
#26128=PLANE('',#28943);
#26129=PLANE('',#28946);
#26130=PLANE('',#28951);
#26131=PLANE('',#28954);
#26132=PLANE('',#28959);
#26133=PLANE('',#28961);
#26134=PLANE('',#28963);
#26135=PLANE('',#28966);
#26136=PLANE('',#28970);
#26137=PLANE('',#28999);
#26138=PLANE('',#29003);
#26139=PLANE('',#29010);
#26140=PLANE('',#29011);
#26141=PLANE('',#29012);
#26142=PLANE('',#29013);
#26143=PLANE('',#29014);
#26144=PLANE('',#29015);
#26145=PLANE('',#29016);
#26146=PLANE('',#29017);
#26147=PLANE('',#29018);
#26148=PLANE('',#29019);
#26149=PLANE('',#29020);
#26150=PLANE('',#29021);
#26151=PLANE('',#29022);
#26152=PLANE('',#29023);
#26153=PLANE('',#29024);
#26154=PLANE('',#29025);
#26155=PLANE('',#29026);
#26156=PLANE('',#29027);
#26157=PLANE('',#29028);
#26158=PLANE('',#29029);
#26159=PLANE('',#29030);
#26160=PLANE('',#29031);
#26161=PLANE('',#29032);
#26162=PLANE('',#29033);
#26163=PLANE('',#29034);
#26164=PLANE('',#29035);
#26165=PLANE('',#29036);
#26166=PLANE('',#29037);
#26167=PLANE('',#29038);
#26168=PLANE('',#29039);
#26169=PLANE('',#29040);
#26170=PLANE('',#29041);
#26171=PLANE('',#29043);
#26879=ADVANCED_FACE('',(#2971),#26071,.T.);
#26880=ADVANCED_FACE('',(#2972),#26072,.T.);
#26881=ADVANCED_FACE('',(#2973),#26073,.T.);
#26882=ADVANCED_FACE('',(#2974),#26074,.T.);
#26883=ADVANCED_FACE('',(#2975),#26075,.T.);
#26884=ADVANCED_FACE('',(#2976),#26076,.T.);
#26885=ADVANCED_FACE('',(#2977),#26077,.T.);
#26886=ADVANCED_FACE('',(#2978),#26078,.T.);
#26887=ADVANCED_FACE('',(#2979),#26079,.T.);
#26888=ADVANCED_FACE('',(#2980),#26080,.T.);
#26889=ADVANCED_FACE('',(#2981),#26081,.T.);
#26890=ADVANCED_FACE('',(#2982),#26082,.T.);
#26891=ADVANCED_FACE('',(#2983),#26083,.T.);
#26892=ADVANCED_FACE('',(#2984),#26084,.T.);
#26893=ADVANCED_FACE('',(#2985),#2731,.F.);
#26894=ADVANCED_FACE('',(#2986,#1874,#1875,#1876,#1877),#26085,.T.);
#26895=ADVANCED_FACE('',(#2987),#1532,.F.);
#26896=ADVANCED_FACE('',(#2988),#2732,.F.);
#26897=ADVANCED_FACE('',(#2989),#1533,.F.);
#26898=ADVANCED_FACE('',(#2990),#2733,.F.);
#26899=ADVANCED_FACE('',(#2991),#1534,.F.);
#26900=ADVANCED_FACE('',(#2992),#2734,.F.);
#26901=ADVANCED_FACE('',(#2993),#1535,.F.);
#26902=ADVANCED_FACE('',(#2994),#2735,.F.);
#26903=ADVANCED_FACE('',(#2995,#1878,#1879,#1880,#1881),#26086,.T.);
#26904=ADVANCED_FACE('',(#2996),#2736,.F.);
#26905=ADVANCED_FACE('',(#2997),#2737,.F.);
#26906=ADVANCED_FACE('',(#2998),#2738,.F.);
#26907=ADVANCED_FACE('',(#2999),#2739,.F.);
#26908=ADVANCED_FACE('',(#3000,#1882,#1883,#1884,#1885),#26087,.T.);
#26909=ADVANCED_FACE('',(#3001),#1536,.F.);
#26910=ADVANCED_FACE('',(#3002),#2740,.F.);
#26911=ADVANCED_FACE('',(#3003),#1537,.F.);
#26912=ADVANCED_FACE('',(#3004),#2741,.F.);
#26913=ADVANCED_FACE('',(#3005),#1538,.F.);
#26914=ADVANCED_FACE('',(#3006),#2742,.F.);
#26915=ADVANCED_FACE('',(#3007),#1539,.F.);
#26916=ADVANCED_FACE('',(#3008),#2743,.F.);
#26917=ADVANCED_FACE('',(#3009),#1348,.T.);
#26918=ADVANCED_FACE('',(#3010),#1349,.T.);
#26919=ADVANCED_FACE('',(#3011),#1350,.T.);
#26920=ADVANCED_FACE('',(#3012),#1540,.T.);
#26921=ADVANCED_FACE('',(#3013),#1541,.F.);
#26922=ADVANCED_FACE('',(#3014),#2744,.F.);
#26923=ADVANCED_FACE('',(#3015,#1886,#1887,#1888,#1889),#26088,.T.);
#26924=ADVANCED_FACE('',(#3016),#2745,.F.);
#26925=ADVANCED_FACE('',(#3017),#2746,.F.);
#26926=ADVANCED_FACE('',(#3018),#2747,.F.);
#26927=ADVANCED_FACE('',(#3019),#2748,.T.);
#26928=ADVANCED_FACE('',(#3020),#26089,.T.);
#26929=ADVANCED_FACE('',(#3021),#2749,.T.);
#26930=ADVANCED_FACE('',(#3022),#26090,.T.);
#26931=ADVANCED_FACE('',(#3023),#2750,.T.);
#26932=ADVANCED_FACE('',(#3024),#26091,.T.);
#26933=ADVANCED_FACE('',(#3025),#2751,.T.);
#26934=ADVANCED_FACE('',(#3026),#26092,.T.);
#26935=ADVANCED_FACE('',(#3027),#1542,.T.);
#26936=ADVANCED_FACE('',(#3028),#26093,.T.);
#26937=ADVANCED_FACE('',(#3029),#1543,.T.);
#26938=ADVANCED_FACE('',(#3030,#1890),#26094,.T.);
#26939=ADVANCED_FACE('',(#3031),#2752,.T.);
#26940=ADVANCED_FACE('',(#3032),#26095,.T.);
#26941=ADVANCED_FACE('',(#3033),#2753,.T.);
#26942=ADVANCED_FACE('',(#3034),#26096,.T.);
#26943=ADVANCED_FACE('',(#3035),#2754,.T.);
#26944=ADVANCED_FACE('',(#3036),#26097,.T.);
#26945=ADVANCED_FACE('',(#3037),#2755,.T.);
#26946=ADVANCED_FACE('',(#3038),#26098,.T.);
#26947=ADVANCED_FACE('',(#3039),#26099,.T.);
#26948=ADVANCED_FACE('',(#3040,#1891,#1892,#1893,#1894,#1895),#26100,.T.);
#26949=ADVANCED_FACE('',(#3041,#1896),#26101,.F.);
#26950=ADVANCED_FACE('',(#3042),#2756,.F.);
#26951=ADVANCED_FACE('',(#3043),#1351,.T.);
#26952=ADVANCED_FACE('',(#3044),#1352,.T.);
#26953=ADVANCED_FACE('',(#3045),#1353,.T.);
#26954=ADVANCED_FACE('',(#3046),#1544,.F.);
#26955=ADVANCED_FACE('',(#3047),#2757,.F.);
#26956=ADVANCED_FACE('',(#3048),#1354,.T.);
#26957=ADVANCED_FACE('',(#3049),#1355,.T.);
#26958=ADVANCED_FACE('',(#3050),#1356,.T.);
#26959=ADVANCED_FACE('',(#3051),#1545,.F.);
#26960=ADVANCED_FACE('',(#3052),#26102,.T.);
#26961=ADVANCED_FACE('',(#3053),#2758,.F.);
#26962=ADVANCED_FACE('',(#3054),#26103,.T.);
#26963=ADVANCED_FACE('',(#3055),#2759,.F.);
#26964=ADVANCED_FACE('',(#3056),#26104,.T.);
#26965=ADVANCED_FACE('',(#3057),#2760,.F.);
#26966=ADVANCED_FACE('',(#3058),#26105,.T.);
#26967=ADVANCED_FACE('',(#3059),#2761,.F.);
#26968=ADVANCED_FACE('',(#3060),#1546,.F.);
#26969=ADVANCED_FACE('',(#3061),#26106,.T.);
#26970=ADVANCED_FACE('',(#3062),#1547,.F.);
#26971=ADVANCED_FACE('',(#3063),#26107,.T.);
#26972=ADVANCED_FACE('',(#3064),#1357,.T.);
#26973=ADVANCED_FACE('',(#3065),#2762,.F.);
#26974=ADVANCED_FACE('',(#3066),#1358,.T.);
#26975=ADVANCED_FACE('',(#3067),#1359,.T.);
#26976=ADVANCED_FACE('',(#3068),#26108,.T.);
#26977=ADVANCED_FACE('',(#3069),#2763,.F.);
#26978=ADVANCED_FACE('',(#3070),#26109,.T.);
#26979=ADVANCED_FACE('',(#3071),#2764,.F.);
#26980=ADVANCED_FACE('',(#3072),#26110,.T.);
#26981=ADVANCED_FACE('',(#3073),#2765,.F.);
#26982=ADVANCED_FACE('',(#3074),#26111,.T.);
#26983=ADVANCED_FACE('',(#3075),#2766,.F.);
#26984=ADVANCED_FACE('',(#3076),#1548,.F.);
#26985=ADVANCED_FACE('',(#3077),#26112,.T.);
#26986=ADVANCED_FACE('',(#3078),#1549,.F.);
#26987=ADVANCED_FACE('',(#3079),#1360,.T.);
#26988=ADVANCED_FACE('',(#3080),#2767,.F.);
#26989=ADVANCED_FACE('',(#3081),#1361,.T.);
#26990=ADVANCED_FACE('',(#3082),#1362,.T.);
#26991=ADVANCED_FACE('',(#3083),#1363,.T.);
#26992=ADVANCED_FACE('',(#3084),#2768,.F.);
#26993=ADVANCED_FACE('',(#3085),#1364,.T.);
#26994=ADVANCED_FACE('',(#3086),#1365,.T.);
#26995=ADVANCED_FACE('',(#3087),#2769,.F.);
#26996=ADVANCED_FACE('',(#3088),#1366,.T.);
#26997=ADVANCED_FACE('',(#3089),#1367,.T.);
#26998=ADVANCED_FACE('',(#3090),#1368,.T.);
#26999=ADVANCED_FACE('',(#3091),#1550,.F.);
#27000=ADVANCED_FACE('',(#3092),#1369,.T.);
#27001=ADVANCED_FACE('',(#3093),#2770,.F.);
#27002=ADVANCED_FACE('',(#3094),#1370,.T.);
#27003=ADVANCED_FACE('',(#3095),#1371,.T.);
#27004=ADVANCED_FACE('',(#3096),#2771,.T.);
#27005=ADVANCED_FACE('',(#3097),#26113,.T.);
#27006=ADVANCED_FACE('',(#3098),#2772,.T.);
#27007=ADVANCED_FACE('',(#3099),#26114,.T.);
#27008=ADVANCED_FACE('',(#3100),#2773,.T.);
#27009=ADVANCED_FACE('',(#3101),#26115,.T.);
#27010=ADVANCED_FACE('',(#3102),#2774,.T.);
#27011=ADVANCED_FACE('',(#3103),#26116,.T.);
#27012=ADVANCED_FACE('',(#3104),#1551,.T.);
#27013=ADVANCED_FACE('',(#3105),#26117,.T.);
#27014=ADVANCED_FACE('',(#3106),#1552,.T.);
#27015=ADVANCED_FACE('',(#3107,#1897),#26118,.F.);
#27016=ADVANCED_FACE('',(#3108),#2775,.T.);
#27017=ADVANCED_FACE('',(#3109),#26119,.T.);
#27018=ADVANCED_FACE('',(#3110),#2776,.T.);
#27019=ADVANCED_FACE('',(#3111),#26120,.T.);
#27020=ADVANCED_FACE('',(#3112),#2777,.T.);
#27021=ADVANCED_FACE('',(#3113),#26121,.T.);
#27022=ADVANCED_FACE('',(#3114),#2778,.T.);
#27023=ADVANCED_FACE('',(#3115),#26122,.T.);
#27024=ADVANCED_FACE('',(#3116),#26123,.T.);
#27025=ADVANCED_FACE('',(#3117),#1553,.T.);
#27026=ADVANCED_FACE('',(#3118),#26124,.T.);
#27027=ADVANCED_FACE('',(#3119,#1898),#26125,.T.);
#27028=ADVANCED_FACE('',(#3120),#1372,.T.);
#27029=ADVANCED_FACE('',(#3121),#2779,.F.);
#27030=ADVANCED_FACE('',(#3122),#1373,.T.);
#27031=ADVANCED_FACE('',(#3123),#1374,.T.);
#27032=ADVANCED_FACE('',(#3124),#1554,.F.);
#27033=ADVANCED_FACE('',(#3125),#26126,.T.);
#27034=ADVANCED_FACE('',(#3126),#2780,.F.);
#27035=ADVANCED_FACE('',(#3127),#26127,.T.);
#27036=ADVANCED_FACE('',(#3128),#2781,.F.);
#27037=ADVANCED_FACE('',(#3129),#26128,.T.);
#27038=ADVANCED_FACE('',(#3130),#2782,.F.);
#27039=ADVANCED_FACE('',(#3131),#26129,.T.);
#27040=ADVANCED_FACE('',(#3132),#2783,.F.);
#27041=ADVANCED_FACE('',(#3133),#1555,.F.);
#27042=ADVANCED_FACE('',(#3134),#26130,.T.);
#27043=ADVANCED_FACE('',(#3135),#1556,.F.);
#27044=ADVANCED_FACE('',(#3136),#26131,.T.);
#27045=ADVANCED_FACE('',(#3137),#26132,.T.);
#27046=ADVANCED_FACE('',(#3138),#2784,.F.);
#27047=ADVANCED_FACE('',(#3139),#26133,.T.);
#27048=ADVANCED_FACE('',(#3140),#2785,.F.);
#27049=ADVANCED_FACE('',(#3141),#26134,.T.);
#27050=ADVANCED_FACE('',(#3142),#2786,.F.);
#27051=ADVANCED_FACE('',(#3143),#26135,.T.);
#27052=ADVANCED_FACE('',(#3144),#2787,.F.);
#27053=ADVANCED_FACE('',(#3145),#1557,.F.);
#27054=ADVANCED_FACE('',(#3146),#26136,.T.);
#27055=ADVANCED_FACE('',(#3147),#1558,.F.);
#27056=ADVANCED_FACE('',(#3148),#1375,.T.);
#27057=ADVANCED_FACE('',(#3149),#2788,.F.);
#27058=ADVANCED_FACE('',(#3150),#1376,.T.);
#27059=ADVANCED_FACE('',(#3151),#1377,.T.);
#27060=ADVANCED_FACE('',(#3152),#2789,.F.);
#27061=ADVANCED_FACE('',(#3153),#1378,.T.);
#27062=ADVANCED_FACE('',(#3154),#1379,.T.);
#27063=ADVANCED_FACE('',(#3155),#1380,.T.);
#27064=ADVANCED_FACE('',(#3156),#1559,.F.);
#27065=ADVANCED_FACE('',(#3157),#1381,.T.);
#27066=ADVANCED_FACE('',(#3158),#2790,.F.);
#27067=ADVANCED_FACE('',(#3159),#1382,.T.);
#27068=ADVANCED_FACE('',(#3160),#1383,.T.);
#27069=ADVANCED_FACE('',(#3161),#1384,.T.);
#27070=ADVANCED_FACE('',(#3162),#2791,.F.);
#27071=ADVANCED_FACE('',(#3163),#1385,.T.);
#27072=ADVANCED_FACE('',(#3164),#1386,.T.);
#27073=ADVANCED_FACE('',(#3165),#1560,.F.);
#27074=ADVANCED_FACE('',(#3166),#1387,.T.);
#27075=ADVANCED_FACE('',(#3167),#2792,.F.);
#27076=ADVANCED_FACE('',(#3168),#1388,.T.);
#27077=ADVANCED_FACE('',(#3169),#1389,.T.);
#27078=ADVANCED_FACE('',(#3170),#2793,.F.);
#27079=ADVANCED_FACE('',(#3171),#1390,.T.);
#27080=ADVANCED_FACE('',(#3172),#1391,.T.);
#27081=ADVANCED_FACE('',(#3173),#1392,.T.);
#27082=ADVANCED_FACE('',(#3174),#1561,.F.);
#27083=ADVANCED_FACE('',(#3175),#1393,.T.);
#27084=ADVANCED_FACE('',(#3176),#2794,.F.);
#27085=ADVANCED_FACE('',(#3177),#1394,.T.);
#27086=ADVANCED_FACE('',(#3178),#1395,.T.);
#27087=ADVANCED_FACE('',(#3179),#2795,.F.);
#27088=ADVANCED_FACE('',(#3180),#1562,.F.);
#27089=ADVANCED_FACE('',(#3181,#1899,#1900),#26137,.F.);
#27090=ADVANCED_FACE('',(#3182),#2796,.F.);
#27091=ADVANCED_FACE('',(#3183,#1901,#1902),#26138,.T.);
#27092=ADVANCED_FACE('',(#3184),#2797,.F.);
#27093=ADVANCED_FACE('',(#3185),#1563,.F.);
#27094=ADVANCED_FACE('',(#3186),#2798,.F.);
#27095=ADVANCED_FACE('',(#3187),#1396,.F.);
#27096=ADVANCED_FACE('',(#3188),#1397,.F.);
#27097=ADVANCED_FACE('',(#3189),#1398,.F.);
#27098=ADVANCED_FACE('',(#3190),#1399,.F.);
#27099=ADVANCED_FACE('',(#3191),#1400,.F.);
#27100=ADVANCED_FACE('',(#3192),#1401,.F.);
#27101=ADVANCED_FACE('',(#3193),#1402,.F.);
#27102=ADVANCED_FACE('',(#3194),#1403,.F.);
#27103=ADVANCED_FACE('',(#3195),#1404,.F.);
#27104=ADVANCED_FACE('',(#3196),#1405,.F.);
#27105=ADVANCED_FACE('',(#3197),#1406,.F.);
#27106=ADVANCED_FACE('',(#3198),#1407,.F.);
#27107=ADVANCED_FACE('',(#3199),#1408,.F.);
#27108=ADVANCED_FACE('',(#3200),#1409,.F.);
#27109=ADVANCED_FACE('',(#3201),#1410,.F.);
#27110=ADVANCED_FACE('',(#3202),#1411,.F.);
#27111=ADVANCED_FACE('',(#3203),#1412,.F.);
#27112=ADVANCED_FACE('',(#3204),#1413,.F.);
#27113=ADVANCED_FACE('',(#3205,#1903),#26139,.F.);
#27114=ADVANCED_FACE('',(#3206),#26140,.F.);
#27115=ADVANCED_FACE('',(#3207),#26141,.F.);
#27116=ADVANCED_FACE('',(#3208),#26142,.F.);
#27117=ADVANCED_FACE('',(#3209),#26143,.F.);
#27118=ADVANCED_FACE('',(#3210),#26144,.F.);
#27119=ADVANCED_FACE('',(#3211),#26145,.F.);
#27120=ADVANCED_FACE('',(#3212),#26146,.F.);
#27121=ADVANCED_FACE('',(#3213),#26147,.F.);
#27122=ADVANCED_FACE('',(#3214),#26148,.F.);
#27123=ADVANCED_FACE('',(#3215),#1414,.F.);
#27124=ADVANCED_FACE('',(#3216),#1415,.F.);
#27125=ADVANCED_FACE('',(#3217),#1416,.F.);
#27126=ADVANCED_FACE('',(#3218),#1417,.F.);
#27127=ADVANCED_FACE('',(#3219),#1418,.F.);
#27128=ADVANCED_FACE('',(#3220),#1419,.F.);
#27129=ADVANCED_FACE('',(#3221),#1420,.F.);
#27130=ADVANCED_FACE('',(#3222),#1421,.F.);
#27131=ADVANCED_FACE('',(#3223),#1422,.F.);
#27132=ADVANCED_FACE('',(#3224),#1423,.F.);
#27133=ADVANCED_FACE('',(#3225),#1424,.F.);
#27134=ADVANCED_FACE('',(#3226),#1425,.F.);
#27135=ADVANCED_FACE('',(#3227),#1426,.F.);
#27136=ADVANCED_FACE('',(#3228),#1427,.F.);
#27137=ADVANCED_FACE('',(#3229),#1428,.F.);
#27138=ADVANCED_FACE('',(#3230),#1429,.F.);
#27139=ADVANCED_FACE('',(#3231),#1430,.F.);
#27140=ADVANCED_FACE('',(#3232),#1431,.F.);
#27141=ADVANCED_FACE('',(#3233),#1432,.F.);
#27142=ADVANCED_FACE('',(#3234),#1433,.F.);
#27143=ADVANCED_FACE('',(#3235),#1434,.F.);
#27144=ADVANCED_FACE('',(#3236),#1435,.F.);
#27145=ADVANCED_FACE('',(#3237,#1904),#26149,.F.);
#27146=ADVANCED_FACE('',(#3238),#26150,.F.);
#27147=ADVANCED_FACE('',(#3239),#1436,.F.);
#27148=ADVANCED_FACE('',(#3240),#1437,.F.);
#27149=ADVANCED_FACE('',(#3241),#1438,.F.);
#27150=ADVANCED_FACE('',(#3242),#1439,.F.);
#27151=ADVANCED_FACE('',(#3243),#1440,.F.);
#27152=ADVANCED_FACE('',(#3244),#1441,.F.);
#27153=ADVANCED_FACE('',(#3245),#1442,.F.);
#27154=ADVANCED_FACE('',(#3246),#1443,.F.);
#27155=ADVANCED_FACE('',(#3247),#1444,.F.);
#27156=ADVANCED_FACE('',(#3248),#1445,.F.);
#27157=ADVANCED_FACE('',(#3249),#26151,.F.);
#27158=ADVANCED_FACE('',(#3250),#1446,.F.);
#27159=ADVANCED_FACE('',(#3251),#1447,.F.);
#27160=ADVANCED_FACE('',(#3252),#1448,.F.);
#27161=ADVANCED_FACE('',(#3253),#1449,.F.);
#27162=ADVANCED_FACE('',(#3254),#1450,.F.);
#27163=ADVANCED_FACE('',(#3255),#1451,.F.);
#27164=ADVANCED_FACE('',(#3256),#1452,.F.);
#27165=ADVANCED_FACE('',(#3257),#1453,.F.);
#27166=ADVANCED_FACE('',(#3258),#26152,.F.);
#27167=ADVANCED_FACE('',(#3259),#26153,.F.);
#27168=ADVANCED_FACE('',(#3260),#26154,.F.);
#27169=ADVANCED_FACE('',(#3261),#26155,.F.);
#27170=ADVANCED_FACE('',(#3262),#26156,.F.);
#27171=ADVANCED_FACE('',(#3263),#26157,.F.);
#27172=ADVANCED_FACE('',(#3264),#26158,.F.);
#27173=ADVANCED_FACE('',(#3265),#26159,.F.);
#27174=ADVANCED_FACE('',(#3266),#26160,.F.);
#27175=ADVANCED_FACE('',(#3267),#26161,.F.);
#27176=ADVANCED_FACE('',(#3268),#26162,.F.);
#27177=ADVANCED_FACE('',(#3269),#26163,.F.);
#27178=ADVANCED_FACE('',(#3270),#26164,.F.);
#27179=ADVANCED_FACE('',(#3271),#26165,.F.);
#27180=ADVANCED_FACE('',(#3272),#26166,.T.);
#27181=ADVANCED_FACE('',(#3273),#26167,.T.);
#27182=ADVANCED_FACE('',(#3274),#26168,.T.);
#27183=ADVANCED_FACE('',(#3275),#26169,.T.);
#27184=ADVANCED_FACE('',(#3276),#26170,.T.);
#27185=ADVANCED_FACE('',(#3277),#1564,.T.);
#27186=ADVANCED_FACE('',(#3278),#26171,.T.);
#27187=ADVANCED_FACE('',(#3279),#1565,.T.);
#28459=CLOSED_SHELL('',(#26879,#26880,#26881,#26882,#26883,#26884,#26885,
#26886,#26887,#26888,#26889,#26890,#26891,#26892,#26893,#26894,#26895,#26896,
#26897,#26898,#26899,#26900,#26901,#26902,#26903,#26904,#26905,#26906,#26907,
#26908,#26909,#26910,#26911,#26912,#26913,#26914,#26915,#26916,#26917,#26918,
#26919,#26920,#26921,#26922,#26923,#26924,#26925,#26926,#26927,#26928,#26929,
#26930,#26931,#26932,#26933,#26934,#26935,#26936,#26937,#26938,#26939,#26940,
#26941,#26942,#26943,#26944,#26945,#26946,#26947,#26948,#26949,#26950,#26951,
#26952,#26953,#26954,#26955,#26956,#26957,#26958,#26959,#26960,#26961,#26962,
#26963,#26964,#26965,#26966,#26967,#26968,#26969,#26970,#26971,#26972,#26973,
#26974,#26975,#26976,#26977,#26978,#26979,#26980,#26981,#26982,#26983,#26984,
#26985,#26986,#26987,#26988,#26989,#26990,#26991,#26992,#26993,#26994,#26995,
#26996,#26997,#26998,#26999,#27000,#27001,#27002,#27003,#27004,#27005,#27006,
#27007,#27008,#27009,#27010,#27011,#27012,#27013,#27014,#27015,#27016,#27017,
#27018,#27019,#27020,#27021,#27022,#27023,#27024,#27025,#27026,#27027,#27028,
#27029,#27030,#27031,#27032,#27033,#27034,#27035,#27036,#27037,#27038,#27039,
#27040,#27041,#27042,#27043,#27044,#27045,#27046,#27047,#27048,#27049,#27050,
#27051,#27052,#27053,#27054,#27055,#27056,#27057,#27058,#27059,#27060,#27061,
#27062,#27063,#27064,#27065,#27066,#27067,#27068,#27069,#27070,#27071,#27072,
#27073,#27074,#27075,#27076,#27077,#27078,#27079,#27080,#27081,#27082,#27083,
#27084,#27085,#27086,#27087,#27088,#27089,#27090,#27091,#27092,#27093,#27094,
#27095,#27096,#27097,#27098,#27099,#27100,#27101,#27102,#27103,#27104,#27105,
#27106,#27107,#27108,#27109,#27110,#27111,#27112,#27113,#27114,#27115,#27116,
#27117,#27118,#27119,#27120,#27121,#27122,#27123,#27124,#27125,#27126,#27127,
#27128,#27129,#27130,#27131,#27132,#27133,#27134,#27135,#27136,#27137,#27138,
#27139,#27140,#27141,#27142,#27143,#27144,#27145,#27146,#27147,#27148,#27149,
#27150,#27151,#27152,#27153,#27154,#27155,#27156,#27157,#27158,#27159,#27160,
#27161,#27162,#27163,#27164,#27165,#27166,#27167,#27168,#27169,#27170,#27171,
#27172,#27173,#27174,#27175,#27176,#27177,#27178,#27179,#27180,#27181,#27182,
#27183,#27184,#27185,#27186,#27187));
#28689=AXIS2_PLACEMENT_3D('',#37678,#30857,#30858);
#28690=AXIS2_PLACEMENT_3D('',#37679,#30859,#30860);
#28691=AXIS2_PLACEMENT_3D('',#37690,#30866,#30867);
#28692=AXIS2_PLACEMENT_3D('',#37700,#30873,#30874);
#28693=AXIS2_PLACEMENT_3D('',#37704,#30877,#30878);
#28694=AXIS2_PLACEMENT_3D('',#37708,#30881,#30882);
#28695=AXIS2_PLACEMENT_3D('',#37712,#30885,#30886);
#28696=AXIS2_PLACEMENT_3D('',#37720,#30891,#30892);
#28697=AXIS2_PLACEMENT_3D('',#37732,#30899,#30900);
#28698=AXIS2_PLACEMENT_3D('',#37743,#30906,#30907);
#28699=AXIS2_PLACEMENT_3D('',#37749,#30911,#30912);
#28700=AXIS2_PLACEMENT_3D('',#37754,#30916,#30917);
#28701=AXIS2_PLACEMENT_3D('',#37757,#30920,#30921);
#28702=AXIS2_PLACEMENT_3D('',#37760,#30924,#30925);
#28703=AXIS2_PLACEMENT_3D('',#37764,#30928,#30929);
#28704=AXIS2_PLACEMENT_3D('',#37765,#30930,#30931);
#28705=AXIS2_PLACEMENT_3D('',#37767,#30932,#30933);
#28706=AXIS2_PLACEMENT_3D('',#37770,#30935,#30936);
#28707=AXIS2_PLACEMENT_3D('',#37771,#30937,#30938);
#28708=AXIS2_PLACEMENT_3D('',#37781,#30943,#30944);
#28709=AXIS2_PLACEMENT_3D('',#37783,#30945,#30946);
#28710=AXIS2_PLACEMENT_3D('',#37785,#30947,#30948);
#28711=AXIS2_PLACEMENT_3D('',#37786,#30949,#30950);
#28712=AXIS2_PLACEMENT_3D('',#37789,#30952,#30953);
#28713=AXIS2_PLACEMENT_3D('',#37790,#30954,#30955);
#28714=AXIS2_PLACEMENT_3D('',#37793,#30957,#30958);
#28715=AXIS2_PLACEMENT_3D('',#37794,#30959,#30960);
#28716=AXIS2_PLACEMENT_3D('',#37797,#30962,#30963);
#28717=AXIS2_PLACEMENT_3D('',#37798,#30964,#30965);
#28718=AXIS2_PLACEMENT_3D('',#37801,#30967,#30968);
#28719=AXIS2_PLACEMENT_3D('',#37802,#30969,#30970);
#28720=AXIS2_PLACEMENT_3D('',#37805,#30972,#30973);
#28721=AXIS2_PLACEMENT_3D('',#37806,#30974,#30975);
#28722=AXIS2_PLACEMENT_3D('',#37809,#30977,#30978);
#28723=AXIS2_PLACEMENT_3D('',#37810,#30979,#30980);
#28724=AXIS2_PLACEMENT_3D('',#37813,#30982,#30983);
#28725=AXIS2_PLACEMENT_3D('',#37814,#30984,#30985);
#28726=AXIS2_PLACEMENT_3D('',#37816,#30986,#30987);
#28727=AXIS2_PLACEMENT_3D('',#37818,#30989,#30990);
#28728=AXIS2_PLACEMENT_3D('',#37828,#30995,#30996);
#28729=AXIS2_PLACEMENT_3D('',#37830,#30997,#30998);
#28730=AXIS2_PLACEMENT_3D('',#37832,#30999,#31000);
#28731=AXIS2_PLACEMENT_3D('',#37833,#31001,#31002);
#28732=AXIS2_PLACEMENT_3D('',#37835,#31004,#31005);
#28733=AXIS2_PLACEMENT_3D('',#37837,#31007,#31008);
#28734=AXIS2_PLACEMENT_3D('',#37839,#31010,#31011);
#28735=AXIS2_PLACEMENT_3D('',#37841,#31012,#31013);
#28736=AXIS2_PLACEMENT_3D('',#37844,#31015,#31016);
#28737=AXIS2_PLACEMENT_3D('',#37845,#31017,#31018);
#28738=AXIS2_PLACEMENT_3D('',#37855,#31023,#31024);
#28739=AXIS2_PLACEMENT_3D('',#37857,#31025,#31026);
#28740=AXIS2_PLACEMENT_3D('',#37859,#31027,#31028);
#28741=AXIS2_PLACEMENT_3D('',#37860,#31029,#31030);
#28742=AXIS2_PLACEMENT_3D('',#37862,#31031,#31032);
#28743=AXIS2_PLACEMENT_3D('',#37864,#31034,#31035);
#28744=AXIS2_PLACEMENT_3D('',#37867,#31037,#31038);
#28745=AXIS2_PLACEMENT_3D('',#37868,#31039,#31040);
#28746=AXIS2_PLACEMENT_3D('',#37870,#31041,#31042);
#28747=AXIS2_PLACEMENT_3D('',#37872,#31044,#31045);
#28748=AXIS2_PLACEMENT_3D('',#37875,#31047,#31048);
#28749=AXIS2_PLACEMENT_3D('',#37876,#31049,#31050);
#28750=AXIS2_PLACEMENT_3D('',#37878,#31051,#31052);
#28751=AXIS2_PLACEMENT_3D('',#37880,#31054,#31055);
#28752=AXIS2_PLACEMENT_3D('',#37883,#31057,#31058);
#28753=AXIS2_PLACEMENT_3D('',#37884,#31059,#31060);
#28754=AXIS2_PLACEMENT_3D('',#37886,#31061,#31062);
#28755=AXIS2_PLACEMENT_3D('',#37888,#31064,#31065);
#28756=AXIS2_PLACEMENT_3D('',#37893,#31067,#31068);
#28757=AXIS2_PLACEMENT_3D('',#37895,#31069,#31070);
#28758=AXIS2_PLACEMENT_3D('',#37898,#31072,#31073);
#28759=AXIS2_PLACEMENT_3D('',#38007,#31076,#31077);
#28760=AXIS2_PLACEMENT_3D('',#38011,#31079,#31080);
#28761=AXIS2_PLACEMENT_3D('',#38015,#31082,#31083);
#28762=AXIS2_PLACEMENT_3D('',#38040,#31086,#31087);
#28763=AXIS2_PLACEMENT_3D('',#38044,#31089,#31090);
#28764=AXIS2_PLACEMENT_3D('',#38093,#31091,#31092);
#28765=AXIS2_PLACEMENT_3D('',#38094,#31093,#31094);
#28766=AXIS2_PLACEMENT_3D('',#38096,#31095,#31096);
#28767=AXIS2_PLACEMENT_3D('',#38098,#31098,#31099);
#28768=AXIS2_PLACEMENT_3D('',#38108,#31104,#31105);
#28769=AXIS2_PLACEMENT_3D('',#38110,#31106,#31107);
#28770=AXIS2_PLACEMENT_3D('',#38112,#31108,#31109);
#28771=AXIS2_PLACEMENT_3D('',#38113,#31110,#31111);
#28772=AXIS2_PLACEMENT_3D('',#38115,#31113,#31114);
#28773=AXIS2_PLACEMENT_3D('',#38117,#31116,#31117);
#28774=AXIS2_PLACEMENT_3D('',#38119,#31119,#31120);
#28775=AXIS2_PLACEMENT_3D('',#38124,#31122,#31123);
#28776=AXIS2_PLACEMENT_3D('',#38127,#31125,#31126);
#28777=AXIS2_PLACEMENT_3D('',#38128,#31127,#31128);
#28778=AXIS2_PLACEMENT_3D('',#38133,#31132,#31133);
#28779=AXIS2_PLACEMENT_3D('',#38136,#31135,#31136);
#28780=AXIS2_PLACEMENT_3D('',#38137,#31137,#31138);
#28781=AXIS2_PLACEMENT_3D('',#38143,#31142,#31143);
#28782=AXIS2_PLACEMENT_3D('',#38146,#31145,#31146);
#28783=AXIS2_PLACEMENT_3D('',#38147,#31147,#31148);
#28784=AXIS2_PLACEMENT_3D('',#38148,#31149,#31150);
#28785=AXIS2_PLACEMENT_3D('',#38152,#31153,#31154);
#28786=AXIS2_PLACEMENT_3D('',#38156,#31156,#31157);
#28787=AXIS2_PLACEMENT_3D('',#38157,#31158,#31159);
#28788=AXIS2_PLACEMENT_3D('',#38158,#31160,#31161);
#28789=AXIS2_PLACEMENT_3D('',#38161,#31164,#31165);
#28790=AXIS2_PLACEMENT_3D('',#38167,#31169,#31170);
#28791=AXIS2_PLACEMENT_3D('',#38168,#31171,#31172);
#28792=AXIS2_PLACEMENT_3D('',#38170,#31174,#31175);
#28793=AXIS2_PLACEMENT_3D('',#38221,#31179,#31180);
#28794=AXIS2_PLACEMENT_3D('',#38223,#31182,#31183);
#28795=AXIS2_PLACEMENT_3D('',#38228,#31185,#31186);
#28796=AXIS2_PLACEMENT_3D('',#38232,#31188,#31189);
#28797=AXIS2_PLACEMENT_3D('',#38236,#31191,#31192);
#28798=AXIS2_PLACEMENT_3D('',#38239,#31194,#31195);
#28799=AXIS2_PLACEMENT_3D('',#38240,#31196,#31197);
#28800=AXIS2_PLACEMENT_3D('',#38245,#31200,#31201);
#28801=AXIS2_PLACEMENT_3D('',#38246,#31202,#31203);
#28802=AXIS2_PLACEMENT_3D('',#38251,#31207,#31208);
#28803=AXIS2_PLACEMENT_3D('',#38254,#31210,#31211);
#28804=AXIS2_PLACEMENT_3D('',#38255,#31212,#31213);
#28805=AXIS2_PLACEMENT_3D('',#38259,#31216,#31217);
#28806=AXIS2_PLACEMENT_3D('',#38263,#31219,#31220);
#28807=AXIS2_PLACEMENT_3D('',#38264,#31221,#31222);
#28808=AXIS2_PLACEMENT_3D('',#38265,#31223,#31224);
#28809=AXIS2_PLACEMENT_3D('',#38270,#31228,#31229);
#28810=AXIS2_PLACEMENT_3D('',#38273,#31231,#31232);
#28811=AXIS2_PLACEMENT_3D('',#38274,#31233,#31234);
#28812=AXIS2_PLACEMENT_3D('',#38277,#31237,#31238);
#28813=AXIS2_PLACEMENT_3D('',#38279,#31240,#31241);
#28814=AXIS2_PLACEMENT_3D('',#38280,#31242,#31243);
#28815=AXIS2_PLACEMENT_3D('',#38281,#31244,#31245);
#28816=AXIS2_PLACEMENT_3D('',#38282,#31246,#31247);
#28817=AXIS2_PLACEMENT_3D('',#38491,#31270,#31271);
#28818=AXIS2_PLACEMENT_3D('',#38496,#31273,#31274);
#28819=AXIS2_PLACEMENT_3D('',#38500,#31276,#31277);
#28820=AXIS2_PLACEMENT_3D('',#38504,#31279,#31280);
#28821=AXIS2_PLACEMENT_3D('',#38507,#31282,#31283);
#28822=AXIS2_PLACEMENT_3D('',#38508,#31284,#31285);
#28823=AXIS2_PLACEMENT_3D('',#38512,#31287,#31288);
#28824=AXIS2_PLACEMENT_3D('',#38514,#31289,#31290);
#28825=AXIS2_PLACEMENT_3D('',#38615,#31294,#31295);
#28826=AXIS2_PLACEMENT_3D('',#38619,#31297,#31298);
#28827=AXIS2_PLACEMENT_3D('',#38662,#31299,#31300);
#28828=AXIS2_PLACEMENT_3D('',#38663,#31301,#31302);
#28829=AXIS2_PLACEMENT_3D('',#38667,#31304,#31305);
#28830=AXIS2_PLACEMENT_3D('',#38669,#31306,#31307);
#28831=AXIS2_PLACEMENT_3D('',#38765,#31311,#31312);
#28832=AXIS2_PLACEMENT_3D('',#38769,#31314,#31315);
#28833=AXIS2_PLACEMENT_3D('',#38818,#31316,#31317);
#28834=AXIS2_PLACEMENT_3D('',#38819,#31318,#31319);
#28835=AXIS2_PLACEMENT_3D('',#38825,#31323,#31324);
#28836=AXIS2_PLACEMENT_3D('',#38828,#31326,#31327);
#28837=AXIS2_PLACEMENT_3D('',#38829,#31328,#31329);
#28838=AXIS2_PLACEMENT_3D('',#38833,#31332,#31333);
#28839=AXIS2_PLACEMENT_3D('',#38835,#31335,#31336);
#28840=AXIS2_PLACEMENT_3D('',#38836,#31337,#31338);
#28841=AXIS2_PLACEMENT_3D('',#38838,#31340,#31341);
#28842=AXIS2_PLACEMENT_3D('',#38841,#31343,#31344);
#28843=AXIS2_PLACEMENT_3D('',#38842,#31345,#31346);
#28844=AXIS2_PLACEMENT_3D('',#38846,#31349,#31350);
#28845=AXIS2_PLACEMENT_3D('',#38847,#31351,#31352);
#28846=AXIS2_PLACEMENT_3D('',#38848,#31353,#31354);
#28847=AXIS2_PLACEMENT_3D('',#38851,#31356,#31357);
#28848=AXIS2_PLACEMENT_3D('',#38852,#31358,#31359);
#28849=AXIS2_PLACEMENT_3D('',#38856,#31362,#31363);
#28850=AXIS2_PLACEMENT_3D('',#38957,#31367,#31368);
#28851=AXIS2_PLACEMENT_3D('',#38958,#31369,#31370);
#28852=AXIS2_PLACEMENT_3D('',#38962,#31372,#31373);
#28853=AXIS2_PLACEMENT_3D('',#38966,#31375,#31376);
#28854=AXIS2_PLACEMENT_3D('',#38970,#31379,#31380);
#28855=AXIS2_PLACEMENT_3D('',#38971,#31381,#31382);
#28856=AXIS2_PLACEMENT_3D('',#39054,#31385,#31386);
#28857=AXIS2_PLACEMENT_3D('',#39089,#31389,#31390);
#28858=AXIS2_PLACEMENT_3D('',#39092,#31393,#31394);
#28859=AXIS2_PLACEMENT_3D('',#39094,#31395,#31396);
#28860=AXIS2_PLACEMENT_3D('',#39096,#31398,#31399);
#28861=AXIS2_PLACEMENT_3D('',#39100,#31402,#31403);
#28862=AXIS2_PLACEMENT_3D('',#39101,#31404,#31405);
#28863=AXIS2_PLACEMENT_3D('',#39103,#31407,#31408);
#28864=AXIS2_PLACEMENT_3D('',#39105,#31410,#31411);
#28865=AXIS2_PLACEMENT_3D('',#39107,#31413,#31414);
#28866=AXIS2_PLACEMENT_3D('',#39109,#31416,#31417);
#28867=AXIS2_PLACEMENT_3D('',#39110,#31418,#31419);
#28868=AXIS2_PLACEMENT_3D('',#39112,#31421,#31422);
#28869=AXIS2_PLACEMENT_3D('',#39114,#31424,#31425);
#28870=AXIS2_PLACEMENT_3D('',#39300,#31428,#31429);
#28871=AXIS2_PLACEMENT_3D('',#39433,#31434,#31435);
#28872=AXIS2_PLACEMENT_3D('',#39468,#31438,#31439);
#28873=AXIS2_PLACEMENT_3D('',#39472,#31441,#31442);
#28874=AXIS2_PLACEMENT_3D('',#39474,#31443,#31444);
#28875=AXIS2_PLACEMENT_3D('',#39570,#31448,#31449);
#28876=AXIS2_PLACEMENT_3D('',#39574,#31451,#31452);
#28877=AXIS2_PLACEMENT_3D('',#39617,#31453,#31454);
#28878=AXIS2_PLACEMENT_3D('',#39692,#31457,#31458);
#28879=AXIS2_PLACEMENT_3D('',#39727,#31461,#31462);
#28880=AXIS2_PLACEMENT_3D('',#39732,#31464,#31465);
#28881=AXIS2_PLACEMENT_3D('',#39735,#31467,#31468);
#28882=AXIS2_PLACEMENT_3D('',#39736,#31469,#31470);
#28883=AXIS2_PLACEMENT_3D('',#39742,#31474,#31475);
#28884=AXIS2_PLACEMENT_3D('',#39746,#31477,#31478);
#28885=AXIS2_PLACEMENT_3D('',#39747,#31479,#31480);
#28886=AXIS2_PLACEMENT_3D('',#39748,#31481,#31482);
#28887=AXIS2_PLACEMENT_3D('',#39754,#31486,#31487);
#28888=AXIS2_PLACEMENT_3D('',#39757,#31489,#31490);
#28889=AXIS2_PLACEMENT_3D('',#39758,#31491,#31492);
#28890=AXIS2_PLACEMENT_3D('',#39759,#31493,#31494);
#28891=AXIS2_PLACEMENT_3D('',#39763,#31497,#31498);
#28892=AXIS2_PLACEMENT_3D('',#39767,#31500,#31501);
#28893=AXIS2_PLACEMENT_3D('',#39768,#31502,#31503);
#28894=AXIS2_PLACEMENT_3D('',#39769,#31504,#31505);
#28895=AXIS2_PLACEMENT_3D('',#39772,#31508,#31509);
#28896=AXIS2_PLACEMENT_3D('',#39778,#31513,#31514);
#28897=AXIS2_PLACEMENT_3D('',#39779,#31515,#31516);
#28898=AXIS2_PLACEMENT_3D('',#39783,#31519,#31520);
#28899=AXIS2_PLACEMENT_3D('',#39833,#31524,#31525);
#28900=AXIS2_PLACEMENT_3D('',#39836,#31528,#31529);
#28901=AXIS2_PLACEMENT_3D('',#39841,#31531,#31532);
#28902=AXIS2_PLACEMENT_3D('',#39845,#31534,#31535);
#28903=AXIS2_PLACEMENT_3D('',#39849,#31537,#31538);
#28904=AXIS2_PLACEMENT_3D('',#39852,#31540,#31541);
#28905=AXIS2_PLACEMENT_3D('',#39853,#31542,#31543);
#28906=AXIS2_PLACEMENT_3D('',#39858,#31546,#31547);
#28907=AXIS2_PLACEMENT_3D('',#39859,#31548,#31549);
#28908=AXIS2_PLACEMENT_3D('',#39864,#31553,#31554);
#28909=AXIS2_PLACEMENT_3D('',#39867,#31556,#31557);
#28910=AXIS2_PLACEMENT_3D('',#39868,#31558,#31559);
#28911=AXIS2_PLACEMENT_3D('',#39872,#31562,#31563);
#28912=AXIS2_PLACEMENT_3D('',#39876,#31565,#31566);
#28913=AXIS2_PLACEMENT_3D('',#39877,#31567,#31568);
#28914=AXIS2_PLACEMENT_3D('',#39878,#31569,#31570);
#28915=AXIS2_PLACEMENT_3D('',#39884,#31574,#31575);
#28916=AXIS2_PLACEMENT_3D('',#39888,#31577,#31578);
#28917=AXIS2_PLACEMENT_3D('',#39889,#31579,#31580);
#28918=AXIS2_PLACEMENT_3D('',#39890,#31581,#31582);
#28919=AXIS2_PLACEMENT_3D('',#39893,#31585,#31586);
#28920=AXIS2_PLACEMENT_3D('',#39896,#31589,#31590);
#28921=AXIS2_PLACEMENT_3D('',#39945,#31594,#31595);
#28922=AXIS2_PLACEMENT_3D('',#39946,#31596,#31597);
#28923=AXIS2_PLACEMENT_3D('',#39947,#31598,#31599);
#28924=AXIS2_PLACEMENT_3D('',#39948,#31600,#31601);
#28925=AXIS2_PLACEMENT_3D('',#39949,#31602,#31603);
#28926=AXIS2_PLACEMENT_3D('',#39950,#31604,#31605);
#28927=AXIS2_PLACEMENT_3D('',#39955,#31607,#31608);
#28928=AXIS2_PLACEMENT_3D('',#39959,#31610,#31611);
#28929=AXIS2_PLACEMENT_3D('',#39963,#31613,#31614);
#28930=AXIS2_PLACEMENT_3D('',#39966,#31616,#31617);
#28931=AXIS2_PLACEMENT_3D('',#40021,#31620,#31621);
#28932=AXIS2_PLACEMENT_3D('',#40025,#31623,#31624);
#28933=AXIS2_PLACEMENT_3D('',#40027,#31625,#31626);
#28934=AXIS2_PLACEMENT_3D('',#40069,#31628,#31629);
#28935=AXIS2_PLACEMENT_3D('',#40073,#31631,#31632);
#28936=AXIS2_PLACEMENT_3D('',#40119,#31633,#31634);
#28937=AXIS2_PLACEMENT_3D('',#40120,#31635,#31636);
#28938=AXIS2_PLACEMENT_3D('',#40126,#31640,#31641);
#28939=AXIS2_PLACEMENT_3D('',#40128,#31642,#31643);
#28940=AXIS2_PLACEMENT_3D('',#40130,#31645,#31646);
#28941=AXIS2_PLACEMENT_3D('',#40134,#31649,#31650);
#28942=AXIS2_PLACEMENT_3D('',#40135,#31651,#31652);
#28943=AXIS2_PLACEMENT_3D('',#40137,#31654,#31655);
#28944=AXIS2_PLACEMENT_3D('',#40139,#31657,#31658);
#28945=AXIS2_PLACEMENT_3D('',#40141,#31659,#31660);
#28946=AXIS2_PLACEMENT_3D('',#40143,#31662,#31663);
#28947=AXIS2_PLACEMENT_3D('',#40147,#31666,#31667);
#28948=AXIS2_PLACEMENT_3D('',#40148,#31668,#31669);
#28949=AXIS2_PLACEMENT_3D('',#40149,#31670,#31671);
#28950=AXIS2_PLACEMENT_3D('',#40152,#31673,#31674);
#28951=AXIS2_PLACEMENT_3D('',#40153,#31675,#31676);
#28952=AXIS2_PLACEMENT_3D('',#40157,#31679,#31680);
#28953=AXIS2_PLACEMENT_3D('',#40255,#31684,#31685);
#28954=AXIS2_PLACEMENT_3D('',#40256,#31686,#31687);
#28955=AXIS2_PLACEMENT_3D('',#40260,#31689,#31690);
#28956=AXIS2_PLACEMENT_3D('',#40264,#31692,#31693);
#28957=AXIS2_PLACEMENT_3D('',#40268,#31696,#31697);
#28958=AXIS2_PLACEMENT_3D('',#40269,#31698,#31699);
#28959=AXIS2_PLACEMENT_3D('',#40270,#31700,#31701);
#28960=AXIS2_PLACEMENT_3D('',#40273,#31704,#31705);
#28961=AXIS2_PLACEMENT_3D('',#40275,#31707,#31708);
#28962=AXIS2_PLACEMENT_3D('',#40277,#31710,#31711);
#28963=AXIS2_PLACEMENT_3D('',#40279,#31713,#31714);
#28964=AXIS2_PLACEMENT_3D('',#40281,#31716,#31717);
#28965=AXIS2_PLACEMENT_3D('',#40284,#31719,#31720);
#28966=AXIS2_PLACEMENT_3D('',#40285,#31721,#31722);
#28967=AXIS2_PLACEMENT_3D('',#40289,#31725,#31726);
#28968=AXIS2_PLACEMENT_3D('',#40290,#31727,#31728);
#28969=AXIS2_PLACEMENT_3D('',#40291,#31729,#31730);
#28970=AXIS2_PLACEMENT_3D('',#40293,#31732,#31733);
#28971=AXIS2_PLACEMENT_3D('',#40295,#31735,#31736);
#28972=AXIS2_PLACEMENT_3D('',#40468,#31739,#31740);
#28973=AXIS2_PLACEMENT_3D('',#40503,#31743,#31744);
#28974=AXIS2_PLACEMENT_3D('',#40507,#31746,#31747);
#28975=AXIS2_PLACEMENT_3D('',#40509,#31748,#31749);
#28976=AXIS2_PLACEMENT_3D('',#40605,#31753,#31754);
#28977=AXIS2_PLACEMENT_3D('',#40609,#31756,#31757);
#28978=AXIS2_PLACEMENT_3D('',#40652,#31758,#31759);
#28979=AXIS2_PLACEMENT_3D('',#40735,#31762,#31763);
#28980=AXIS2_PLACEMENT_3D('',#40829,#31768,#31769);
#28981=AXIS2_PLACEMENT_3D('',#40833,#31771,#31772);
#28982=AXIS2_PLACEMENT_3D('',#40835,#31773,#31774);
#28983=AXIS2_PLACEMENT_3D('',#40877,#31776,#31777);
#28984=AXIS2_PLACEMENT_3D('',#40881,#31779,#31780);
#28985=AXIS2_PLACEMENT_3D('',#40924,#31781,#31782);
#28986=AXIS2_PLACEMENT_3D('',#41011,#31785,#31786);
#28987=AXIS2_PLACEMENT_3D('',#41046,#31789,#31790);
#28988=AXIS2_PLACEMENT_3D('',#41050,#31792,#31793);
#28989=AXIS2_PLACEMENT_3D('',#41052,#31794,#31795);
#28990=AXIS2_PLACEMENT_3D('',#41148,#31799,#31800);
#28991=AXIS2_PLACEMENT_3D('',#41152,#31802,#31803);
#28992=AXIS2_PLACEMENT_3D('',#41195,#31804,#31805);
#28993=AXIS2_PLACEMENT_3D('',#41278,#31808,#31809);
#28994=AXIS2_PLACEMENT_3D('',#41313,#31812,#31813);
#28995=AXIS2_PLACEMENT_3D('',#41315,#31814,#31815);
#28996=AXIS2_PLACEMENT_3D('',#41318,#31817,#31818);
#28997=AXIS2_PLACEMENT_3D('',#41319,#31819,#31820);
#28998=AXIS2_PLACEMENT_3D('',#41322,#31822,#31823);
#28999=AXIS2_PLACEMENT_3D('',#41323,#31824,#31825);
#29000=AXIS2_PLACEMENT_3D('',#41325,#31826,#31827);
#29001=AXIS2_PLACEMENT_3D('',#41326,#31828,#31829);
#29002=AXIS2_PLACEMENT_3D('',#41328,#31830,#31831);
#29003=AXIS2_PLACEMENT_3D('',#41330,#31833,#31834);
#29004=AXIS2_PLACEMENT_3D('',#41333,#31836,#31837);
#29005=AXIS2_PLACEMENT_3D('',#41334,#31838,#31839);
#29006=AXIS2_PLACEMENT_3D('',#41337,#31841,#31842);
#29007=AXIS2_PLACEMENT_3D('',#41338,#31843,#31844);
#29008=AXIS2_PLACEMENT_3D('',#41341,#31846,#31847);
#29009=AXIS2_PLACEMENT_3D('',#41342,#31848,#31849);
#29010=AXIS2_PLACEMENT_3D('',#41574,#31869,#31870);
#29011=AXIS2_PLACEMENT_3D('',#41575,#31871,#31872);
#29012=AXIS2_PLACEMENT_3D('',#41581,#31876,#31877);
#29013=AXIS2_PLACEMENT_3D('',#41585,#31880,#31881);
#29014=AXIS2_PLACEMENT_3D('',#41589,#31884,#31885);
#29015=AXIS2_PLACEMENT_3D('',#41593,#31888,#31889);
#29016=AXIS2_PLACEMENT_3D('',#41597,#31892,#31893);
#29017=AXIS2_PLACEMENT_3D('',#41601,#31896,#31897);
#29018=AXIS2_PLACEMENT_3D('',#41605,#31900,#31901);
#29019=AXIS2_PLACEMENT_3D('',#41607,#31903,#31904);
#29020=AXIS2_PLACEMENT_3D('',#41886,#31927,#31928);
#29021=AXIS2_PLACEMENT_3D('',#41887,#31929,#31930);
#29022=AXIS2_PLACEMENT_3D('',#42003,#31944,#31945);
#29023=AXIS2_PLACEMENT_3D('',#42095,#31956,#31957);
#29024=AXIS2_PLACEMENT_3D('',#42099,#31960,#31961);
#29025=AXIS2_PLACEMENT_3D('',#42101,#31963,#31964);
#29026=AXIS2_PLACEMENT_3D('',#42102,#31965,#31966);
#29027=AXIS2_PLACEMENT_3D('',#42108,#31970,#31971);
#29028=AXIS2_PLACEMENT_3D('',#42112,#31974,#31975);
#29029=AXIS2_PLACEMENT_3D('',#42116,#31978,#31979);
#29030=AXIS2_PLACEMENT_3D('',#42120,#31982,#31983);
#29031=AXIS2_PLACEMENT_3D('',#42124,#31986,#31987);
#29032=AXIS2_PLACEMENT_3D('',#42128,#31990,#31991);
#29033=AXIS2_PLACEMENT_3D('',#42132,#31994,#31995);
#29034=AXIS2_PLACEMENT_3D('',#42136,#31998,#31999);
#29035=AXIS2_PLACEMENT_3D('',#42140,#32002,#32003);
#29036=AXIS2_PLACEMENT_3D('',#42142,#32005,#32006);
#29037=AXIS2_PLACEMENT_3D('',#42143,#32007,#32008);
#29038=AXIS2_PLACEMENT_3D('',#42144,#32009,#32010);
#29039=AXIS2_PLACEMENT_3D('',#42145,#32011,#32012);
#29040=AXIS2_PLACEMENT_3D('',#42147,#32014,#32015);
#29041=AXIS2_PLACEMENT_3D('',#42149,#32017,#32018);
#29042=AXIS2_PLACEMENT_3D('',#42150,#32019,#32020);
#29043=AXIS2_PLACEMENT_3D('',#42151,#32021,#32022);
#29044=AXIS2_PLACEMENT_3D('',#42152,#32023,#32024);
#30857=DIRECTION('axis',(0.,0.,1.));
#30858=DIRECTION('refdir',(1.,0.,0.));
#30859=DIRECTION('center_axis',(-0.707106781186548,0.707106781186548,0.));
#30860=DIRECTION('ref_axis',(0.,0.,1.));
#30861=DIRECTION('',(0.577350269189581,0.577350269189581,-0.577350269189715));
#30862=DIRECTION('',(0.,0.,-1.));
#30863=DIRECTION('',(-0.577350269189619,-0.577350269189619,-0.57735026918964));
#30864=DIRECTION('',(-0.577350269189617,-0.577350269189617,0.577350269189644));
#30865=DIRECTION('',(0.,0.,1.));
#30866=DIRECTION('center_axis',(0.,0.70710678118656,-0.707106781186535));
#30867=DIRECTION('ref_axis',(-1.,0.,0.));
#30868=DIRECTION('',(1.,0.,0.));
#30869=DIRECTION('',(-0.577350269189619,0.577350269189619,0.57735026918964));
#30870=DIRECTION('',(0.577350269189614,0.577350269189621,0.577350269189642));
#30871=DIRECTION('',(-1.,0.,0.));
#30872=DIRECTION('',(0.577350269189605,-0.577350269189626,-0.577350269189646));
#30873=DIRECTION('center_axis',(0.,1.,0.));
#30874=DIRECTION('ref_axis',(-1.,0.,0.));
#30875=DIRECTION('',(-1.,0.,0.));
#30876=DIRECTION('',(0.,0.,1.));
#30877=DIRECTION('center_axis',(0.,0.707106781186629,0.707106781186466));
#30878=DIRECTION('ref_axis',(1.,0.,0.));
#30879=DIRECTION('',(1.,0.,0.));
#30880=DIRECTION('',(-0.577350269189581,0.577350269189581,-0.577350269189715));
#30881=DIRECTION('center_axis',(0.707106781186548,0.707106781186548,0.));
#30882=DIRECTION('ref_axis',(0.,0.,-1.));
#30883=DIRECTION('',(0.,0.,-1.));
#30884=DIRECTION('',(-0.577350269189617,0.577350269189617,-0.577350269189644));
#30885=DIRECTION('center_axis',(0.707106781186564,0.,-0.707106781186531));
#30886=DIRECTION('ref_axis',(-0.707106781186531,0.,-0.707106781186564));
#30887=DIRECTION('',(0.,-1.,0.));
#30888=DIRECTION('',(0.577350269189617,0.577350269189617,0.577350269189644));
#30889=DIRECTION('',(0.577350269189614,-0.577350269189621,0.577350269189642));
#30890=DIRECTION('',(0.,1.,0.));
#30891=DIRECTION('center_axis',(1.,0.,0.));
#30892=DIRECTION('ref_axis',(0.,1.,0.));
#30893=DIRECTION('',(0.,1.,0.));
#30894=DIRECTION('',(0.,1.,0.));
#30895=DIRECTION('',(0.,1.,0.));
#30896=DIRECTION('',(0.,1.,0.));
#30897=DIRECTION('',(0.,1.,0.));
#30898=DIRECTION('',(0.,0.,1.));
#30899=DIRECTION('center_axis',(-0.707106781186548,-0.707106781186548,0.));
#30900=DIRECTION('ref_axis',(0.,0.,1.));
#30901=DIRECTION('',(-0.577350269189581,0.577350269189581,0.577350269189715));
#30902=DIRECTION('',(0.,0.,-1.));
#30903=DIRECTION('',(0.577350269189617,-0.577350269189617,-0.577350269189644));
#30904=DIRECTION('',(0.577350269189619,-0.577350269189619,0.57735026918964));
#30905=DIRECTION('',(0.,0.,1.));
#30906=DIRECTION('center_axis',(0.,-1.,0.));
#30907=DIRECTION('ref_axis',(1.,0.,0.));
#30908=DIRECTION('',(-1.,0.,0.));
#30909=DIRECTION('',(0.,0.,-1.));
#30910=DIRECTION('',(1.,0.,0.));
#30911=DIRECTION('center_axis',(0.,-0.70710678118656,-0.707106781186535));
#30912=DIRECTION('ref_axis',(-1.,0.,0.));
#30913=DIRECTION('',(-0.577350269189614,-0.577350269189621,0.577350269189642));
#30914=DIRECTION('',(1.,0.,0.));
#30915=DIRECTION('',(0.577350269189619,0.577350269189619,-0.57735026918964));
#30916=DIRECTION('center_axis',(-0.707106781186564,0.,-0.707106781186531));
#30917=DIRECTION('ref_axis',(-0.707106781186531,0.,0.707106781186564));
#30918=DIRECTION('',(0.,-1.,0.));
#30919=DIRECTION('',(0.,1.,0.));
#30920=DIRECTION('center_axis',(0.,-0.707106781186629,0.707106781186466));
#30921=DIRECTION('ref_axis',(1.,0.,0.));
#30922=DIRECTION('',(0.577350269189581,0.577350269189581,0.577350269189715));
#30923=DIRECTION('',(-1.,0.,0.));
#30924=DIRECTION('center_axis',(0.,0.,1.));
#30925=DIRECTION('ref_axis',(1.,0.,0.));
#30926=DIRECTION('',(1.,0.,0.));
#30927=DIRECTION('',(0.,-1.,0.));
#30928=DIRECTION('center_axis',(0.707106781186548,-0.707106781186548,0.));
#30929=DIRECTION('ref_axis',(0.,0.,-1.));
#30930=DIRECTION('center_axis',(0.,-1.,0.));
#30931=DIRECTION('ref_axis',(1.,0.,0.));
#30932=DIRECTION('center_axis',(0.,-1.,0.));
#30933=DIRECTION('ref_axis',(1.,0.,0.));
#30934=DIRECTION('',(0.707106781186554,0.707106781186541,8.65956056235501E-17));
#30935=DIRECTION('center_axis',(0.,1.,0.));
#30936=DIRECTION('ref_axis',(1.,0.,0.));
#30937=DIRECTION('center_axis',(0.,-1.,0.));
#30938=DIRECTION('ref_axis',(0.,0.,-1.));
#30939=DIRECTION('',(0.,0.,1.));
#30940=DIRECTION('',(-1.,0.,0.));
#30941=DIRECTION('',(0.,0.,-1.));
#30942=DIRECTION('',(1.,0.,0.));
#30943=DIRECTION('center_axis',(0.,-1.,0.));
#30944=DIRECTION('ref_axis',(1.,0.,0.));
#30945=DIRECTION('center_axis',(0.,-1.,0.));
#30946=DIRECTION('ref_axis',(1.,0.,0.));
#30947=DIRECTION('center_axis',(0.,-1.,0.));
#30948=DIRECTION('ref_axis',(1.,0.,0.));
#30949=DIRECTION('center_axis',(0.,1.,0.));
#30950=DIRECTION('ref_axis',(1.,0.,0.));
#30951=DIRECTION('',(0.,1.,0.));
#30952=DIRECTION('center_axis',(0.,-1.,0.));
#30953=DIRECTION('ref_axis',(1.,0.,0.));
#30954=DIRECTION('center_axis',(0.,-1.,0.));
#30955=DIRECTION('ref_axis',(1.,0.,0.));
#30956=DIRECTION('',(0.707106781186554,0.707106781186541,8.65956056235501E-17));
#30957=DIRECTION('center_axis',(0.,1.,0.));
#30958=DIRECTION('ref_axis',(1.,0.,0.));
#30959=DIRECTION('center_axis',(0.,1.,0.));
#30960=DIRECTION('ref_axis',(1.,0.,0.));
#30961=DIRECTION('',(0.,1.,0.));
#30962=DIRECTION('center_axis',(0.,-1.,0.));
#30963=DIRECTION('ref_axis',(1.,0.,0.));
#30964=DIRECTION('center_axis',(0.,-1.,0.));
#30965=DIRECTION('ref_axis',(1.,0.,0.));
#30966=DIRECTION('',(0.707106781186554,0.707106781186541,8.65956056235501E-17));
#30967=DIRECTION('center_axis',(0.,1.,0.));
#30968=DIRECTION('ref_axis',(1.,0.,0.));
#30969=DIRECTION('center_axis',(0.,1.,0.));
#30970=DIRECTION('ref_axis',(1.,0.,0.));
#30971=DIRECTION('',(0.,1.,0.));
#30972=DIRECTION('center_axis',(0.,-1.,0.));
#30973=DIRECTION('ref_axis',(1.,0.,0.));
#30974=DIRECTION('center_axis',(0.,-1.,0.));
#30975=DIRECTION('ref_axis',(1.,0.,0.));
#30976=DIRECTION('',(0.707106781186554,0.707106781186541,8.65956056235501E-17));
#30977=DIRECTION('center_axis',(0.,1.,0.));
#30978=DIRECTION('ref_axis',(1.,0.,0.));
#30979=DIRECTION('center_axis',(0.,1.,0.));
#30980=DIRECTION('ref_axis',(1.,0.,0.));
#30981=DIRECTION('',(0.,1.,0.));
#30982=DIRECTION('center_axis',(0.,-1.,0.));
#30983=DIRECTION('ref_axis',(1.,0.,0.));
#30984=DIRECTION('center_axis',(0.,1.,0.));
#30985=DIRECTION('ref_axis',(1.,0.,0.));
#30986=DIRECTION('center_axis',(0.,1.,0.));
#30987=DIRECTION('ref_axis',(1.,0.,0.));
#30988=DIRECTION('',(0.707106781186554,-0.707106781186541,-8.65956056235501E-17));
#30989=DIRECTION('center_axis',(0.,1.,0.));
#30990=DIRECTION('ref_axis',(0.,0.,1.));
#30991=DIRECTION('',(0.,0.,1.));
#30992=DIRECTION('',(1.,0.,0.));
#30993=DIRECTION('',(0.,0.,-1.));
#30994=DIRECTION('',(-1.,0.,0.));
#30995=DIRECTION('center_axis',(0.,1.,0.));
#30996=DIRECTION('ref_axis',(1.,0.,0.));
#30997=DIRECTION('center_axis',(0.,1.,0.));
#30998=DIRECTION('ref_axis',(1.,0.,0.));
#30999=DIRECTION('center_axis',(0.,1.,0.));
#31000=DIRECTION('ref_axis',(1.,0.,0.));
#31001=DIRECTION('center_axis',(0.,1.,0.));
#31002=DIRECTION('ref_axis',(1.,0.,0.));
#31003=DIRECTION('',(0.707106781186554,-0.707106781186541,-8.65956056235501E-17));
#31004=DIRECTION('center_axis',(0.,1.,0.));
#31005=DIRECTION('ref_axis',(1.,0.,0.));
#31006=DIRECTION('',(0.707106781186554,-0.707106781186541,-8.65956056235501E-17));
#31007=DIRECTION('center_axis',(0.,1.,0.));
#31008=DIRECTION('ref_axis',(1.,0.,0.));
#31009=DIRECTION('',(0.707106781186554,-0.707106781186541,-8.65956056235501E-17));
#31010=DIRECTION('center_axis',(0.,1.,0.));
#31011=DIRECTION('ref_axis',(1.,0.,0.));
#31012=DIRECTION('center_axis',(0.,1.,0.));
#31013=DIRECTION('ref_axis',(1.,0.,0.));
#31014=DIRECTION('',(0.707106781186554,-0.707106781186541,-8.65956056235501E-17));
#31015=DIRECTION('center_axis',(0.,-1.,0.));
#31016=DIRECTION('ref_axis',(1.,0.,0.));
#31017=DIRECTION('center_axis',(0.,1.,0.));
#31018=DIRECTION('ref_axis',(0.,0.,1.));
#31019=DIRECTION('',(0.,0.,1.));
#31020=DIRECTION('',(1.,0.,0.));
#31021=DIRECTION('',(0.,0.,-1.));
#31022=DIRECTION('',(-1.,0.,0.));
#31023=DIRECTION('center_axis',(0.,1.,0.));
#31024=DIRECTION('ref_axis',(1.,0.,0.));
#31025=DIRECTION('center_axis',(0.,1.,0.));
#31026=DIRECTION('ref_axis',(1.,0.,0.));
#31027=DIRECTION('center_axis',(0.,1.,0.));
#31028=DIRECTION('ref_axis',(1.,0.,0.));
#31029=DIRECTION('center_axis',(0.,1.,0.));
#31030=DIRECTION('ref_axis',(1.,0.,0.));
#31031=DIRECTION('center_axis',(0.,1.,0.));
#31032=DIRECTION('ref_axis',(1.,0.,0.));
#31033=DIRECTION('',(0.,1.,0.));
#31034=DIRECTION('center_axis',(0.,1.,0.));
#31035=DIRECTION('ref_axis',(1.,0.,0.));
#31036=DIRECTION('',(0.707106781186554,-0.707106781186541,-8.65956056235501E-17));
#31037=DIRECTION('center_axis',(0.,-1.,0.));
#31038=DIRECTION('ref_axis',(1.,0.,0.));
#31039=DIRECTION('center_axis',(0.,1.,0.));
#31040=DIRECTION('ref_axis',(1.,0.,0.));
#31041=DIRECTION('center_axis',(0.,1.,0.));
#31042=DIRECTION('ref_axis',(1.,0.,0.));
#31043=DIRECTION('',(0.,1.,0.));
#31044=DIRECTION('center_axis',(0.,1.,0.));
#31045=DIRECTION('ref_axis',(1.,0.,0.));
#31046=DIRECTION('',(0.707106781186554,-0.707106781186541,-8.65956056235501E-17));
#31047=DIRECTION('center_axis',(0.,-1.,0.));
#31048=DIRECTION('ref_axis',(1.,0.,0.));
#31049=DIRECTION('center_axis',(0.,1.,0.));
#31050=DIRECTION('ref_axis',(1.,0.,0.));
#31051=DIRECTION('center_axis',(0.,1.,0.));
#31052=DIRECTION('ref_axis',(1.,0.,0.));
#31053=DIRECTION('',(0.,1.,0.));
#31054=DIRECTION('center_axis',(0.,1.,0.));
#31055=DIRECTION('ref_axis',(1.,0.,0.));
#31056=DIRECTION('',(0.707106781186554,-0.707106781186541,-8.65956056235501E-17));
#31057=DIRECTION('center_axis',(0.,-1.,0.));
#31058=DIRECTION('ref_axis',(1.,0.,0.));
#31059=DIRECTION('center_axis',(0.,1.,0.));
#31060=DIRECTION('ref_axis',(1.,0.,0.));
#31061=DIRECTION('center_axis',(0.,1.,0.));
#31062=DIRECTION('ref_axis',(1.,0.,0.));
#31063=DIRECTION('',(0.,1.,0.));
#31064=DIRECTION('center_axis',(0.,-1.,0.));
#31065=DIRECTION('ref_axis',(6.12323399573677E-17,0.,-1.));
#31066=DIRECTION('',(-0.315789473684196,0.707106781186531,-0.632674488430095));
#31067=DIRECTION('center_axis',(0.,1.,0.));
#31068=DIRECTION('ref_axis',(1.,0.,0.));
#31069=DIRECTION('center_axis',(0.,1.,0.));
#31070=DIRECTION('ref_axis',(1.,0.,0.));
#31071=DIRECTION('',(-0.315789473684196,-0.707106781186531,0.632674488430095));
#31072=DIRECTION('center_axis',(0.,-1.,0.));
#31073=DIRECTION('ref_axis',(1.,0.,0.));
#31074=DIRECTION('',(0.238798209365739,-0.687106448937468,0.686192497067885));
#31075=DIRECTION('',(0.238798209365798,0.687106448937561,-0.686192497067771));
#31076=DIRECTION('center_axis',(1.,0.,0.));
#31077=DIRECTION('ref_axis',(0.,-0.707106781186543,0.707106781186552));
#31078=DIRECTION('',(1.,0.,0.));
#31079=DIRECTION('center_axis',(1.,0.,0.));
#31080=DIRECTION('ref_axis',(0.,-0.707106781186543,0.707106781186552));
#31081=DIRECTION('',(-1.,0.,0.));
#31082=DIRECTION('center_axis',(-1.,0.,0.));
#31083=DIRECTION('ref_axis',(0.,-0.707106781186543,0.707106781186552));
#31084=DIRECTION('',(1.,0.,0.));
#31085=DIRECTION('',(1.,0.,0.));
#31086=DIRECTION('center_axis',(0.,1.,0.));
#31087=DIRECTION('ref_axis',(1.,0.,0.));
#31088=DIRECTION('',(0.,1.,0.));
#31089=DIRECTION('center_axis',(0.,-1.,0.));
#31090=DIRECTION('ref_axis',(1.,0.,0.));
#31091=DIRECTION('center_axis',(0.,-1.,0.));
#31092=DIRECTION('ref_axis',(1.,0.,0.));
#31093=DIRECTION('center_axis',(0.,-1.,0.));
#31094=DIRECTION('ref_axis',(1.,0.,0.));
#31095=DIRECTION('center_axis',(0.,-1.,0.));
#31096=DIRECTION('ref_axis',(1.,0.,0.));
#31097=DIRECTION('',(0.707106781186554,0.707106781186541,8.65956056235501E-17));
#31098=DIRECTION('center_axis',(0.,-1.,0.));
#31099=DIRECTION('ref_axis',(0.,0.,-1.));
#31100=DIRECTION('',(0.,0.,1.));
#31101=DIRECTION('',(-1.,0.,0.));
#31102=DIRECTION('',(0.,0.,-1.));
#31103=DIRECTION('',(1.,0.,0.));
#31104=DIRECTION('center_axis',(0.,-1.,0.));
#31105=DIRECTION('ref_axis',(1.,0.,0.));
#31106=DIRECTION('center_axis',(0.,-1.,0.));
#31107=DIRECTION('ref_axis',(1.,0.,0.));
#31108=DIRECTION('center_axis',(0.,-1.,0.));
#31109=DIRECTION('ref_axis',(1.,0.,0.));
#31110=DIRECTION('center_axis',(0.,-1.,0.));
#31111=DIRECTION('ref_axis',(1.,0.,0.));
#31112=DIRECTION('',(0.707106781186554,0.707106781186541,8.65956056235501E-17));
#31113=DIRECTION('center_axis',(0.,-1.,0.));
#31114=DIRECTION('ref_axis',(1.,0.,0.));
#31115=DIRECTION('',(0.707106781186554,0.707106781186541,8.65956056235501E-17));
#31116=DIRECTION('center_axis',(0.,-1.,0.));
#31117=DIRECTION('ref_axis',(1.,0.,0.));
#31118=DIRECTION('',(0.707106781186554,0.707106781186541,8.65956056235501E-17));
#31119=DIRECTION('center_axis',(-1.,0.,0.));
#31120=DIRECTION('ref_axis',(0.,-0.707106781186543,-0.707106781186552));
#31121=DIRECTION('',(-0.707106781186566,-0.707106781186529,0.));
#31122=DIRECTION('center_axis',(1.,0.,0.));
#31123=DIRECTION('ref_axis',(0.,-0.707106781186543,-0.707106781186552));
#31124=DIRECTION('',(0.707106781186548,0.,0.707106781186548));
#31125=DIRECTION('center_axis',(-1.,0.,0.));
#31126=DIRECTION('ref_axis',(0.,-0.707106781186543,-0.707106781186552));
#31127=DIRECTION('center_axis',(0.707106781186566,-0.707106781186529,0.));
#31128=DIRECTION('ref_axis',(0.,0.,-1.));
#31129=DIRECTION('',(0.,0.,1.));
#31130=DIRECTION('',(-0.707106781186529,-0.707106781186566,0.));
#31131=DIRECTION('',(0.,0.,-1.));
#31132=DIRECTION('center_axis',(-1.,0.,0.));
#31133=DIRECTION('ref_axis',(0.,-0.707106781186543,0.707106781186552));
#31134=DIRECTION('',(-0.707106781186548,0.,0.707106781186548));
#31135=DIRECTION('center_axis',(-1.,0.,0.));
#31136=DIRECTION('ref_axis',(0.,-0.707106781186543,0.707106781186552));
#31137=DIRECTION('center_axis',(0.707106781186548,0.,0.707106781186548));
#31138=DIRECTION('ref_axis',(0.707106781186548,0.,-0.707106781186548));
#31139=DIRECTION('',(0.,1.,0.));
#31140=DIRECTION('',(-0.707106781186548,0.,0.707106781186548));
#31141=DIRECTION('',(0.,-1.,0.));
#31142=DIRECTION('center_axis',(-1.,0.,0.));
#31143=DIRECTION('ref_axis',(0.,0.707106781186543,0.707106781186552));
#31144=DIRECTION('',(-0.707106781186566,0.707106781186529,0.));
#31145=DIRECTION('center_axis',(1.,0.,0.));
#31146=DIRECTION('ref_axis',(0.,0.707106781186543,0.707106781186552));
#31147=DIRECTION('center_axis',(-1.,0.,0.));
#31148=DIRECTION('ref_axis',(0.,0.707106781186543,0.707106781186552));
#31149=DIRECTION('center_axis',(0.707106781186566,0.707106781186529,0.));
#31150=DIRECTION('ref_axis',(0.,0.,-1.));
#31151=DIRECTION('',(0.,0.,-1.));
#31152=DIRECTION('',(-0.707106781186529,0.707106781186566,0.));
#31153=DIRECTION('center_axis',(-1.,0.,0.));
#31154=DIRECTION('ref_axis',(0.,0.707106781186542,-0.707106781186553));
#31155=DIRECTION('',(-0.707106781186548,0.,-0.707106781186548));
#31156=DIRECTION('center_axis',(1.,0.,0.));
#31157=DIRECTION('ref_axis',(0.,0.707106781186542,-0.707106781186553));
#31158=DIRECTION('center_axis',(-1.,0.,0.));
#31159=DIRECTION('ref_axis',(0.,0.707106781186542,-0.707106781186553));
#31160=DIRECTION('center_axis',(0.707106781186548,0.,-0.707106781186548));
#31161=DIRECTION('ref_axis',(-0.707106781186548,0.,-0.707106781186548));
#31162=DIRECTION('',(0.,-1.,0.));
#31163=DIRECTION('',(0.,1.,0.));
#31164=DIRECTION('center_axis',(1.,0.,0.));
#31165=DIRECTION('ref_axis',(0.,0.707106781186542,-0.707106781186553));
#31166=DIRECTION('',(-1.,0.,0.));
#31167=DIRECTION('',(-1.,0.,0.));
#31168=DIRECTION('',(-1.,0.,0.));
#31169=DIRECTION('center_axis',(-1.,0.,0.));
#31170=DIRECTION('ref_axis',(0.,0.707106781186542,-0.707106781186553));
#31171=DIRECTION('center_axis',(0.,0.,-1.));
#31172=DIRECTION('ref_axis',(0.,1.,0.));
#31173=DIRECTION('',(1.,0.,0.));
#31174=DIRECTION('center_axis',(1.,0.,0.));
#31175=DIRECTION('ref_axis',(0.,-0.707106781186543,-0.707106781186552));
#31176=DIRECTION('',(-1.,0.,0.));
#31177=DIRECTION('',(-1.,0.,0.));
#31178=DIRECTION('',(-1.,0.,0.));
#31179=DIRECTION('center_axis',(-1.,0.,0.));
#31180=DIRECTION('ref_axis',(0.,-0.707106781186543,-0.707106781186552));
#31181=DIRECTION('',(1.,0.,0.));
#31182=DIRECTION('center_axis',(1.,0.,0.));
#31183=DIRECTION('ref_axis',(0.,0.,-1.));
#31184=DIRECTION('',(0.,0.,-1.));
#31185=DIRECTION('center_axis',(1.,0.,0.));
#31186=DIRECTION('ref_axis',(0.,-0.707106781186568,0.707106781186527));
#31187=DIRECTION('',(0.,-1.,0.));
#31188=DIRECTION('center_axis',(1.,0.,0.));
#31189=DIRECTION('ref_axis',(0.,0.707106781186568,0.707106781186527));
#31190=DIRECTION('',(0.,0.,1.));
#31191=DIRECTION('center_axis',(1.,0.,0.));
#31192=DIRECTION('ref_axis',(0.,0.707106781186568,-0.707106781186527));
#31193=DIRECTION('',(0.,1.,0.));
#31194=DIRECTION('center_axis',(1.,0.,0.));
#31195=DIRECTION('ref_axis',(0.,-0.707106781186566,-0.707106781186529));
#31196=DIRECTION('center_axis',(1.,0.,0.));
#31197=DIRECTION('ref_axis',(0.,-0.707106781186543,-0.707106781186552));
#31198=DIRECTION('',(0.707106781186573,0.,-0.707106781186522));
#31199=DIRECTION('',(-0.707106781186592,0.707106781186504,0.));
#31200=DIRECTION('center_axis',(1.,0.,0.));
#31201=DIRECTION('ref_axis',(0.,-0.707106781186543,-0.707106781186552));
#31202=DIRECTION('center_axis',(-0.707106781186548,0.,-0.707106781186548));
#31203=DIRECTION('ref_axis',(-0.707106781186548,0.,0.707106781186548));
#31204=DIRECTION('',(0.,1.,0.));
#31205=DIRECTION('',(0.707106781186548,0.,-0.707106781186548));
#31206=DIRECTION('',(0.,-1.,0.));
#31207=DIRECTION('center_axis',(1.,0.,0.));
#31208=DIRECTION('ref_axis',(0.,0.707106781186542,-0.707106781186553));
#31209=DIRECTION('',(0.707106781186592,0.707106781186504,0.));
#31210=DIRECTION('center_axis',(1.,0.,0.));
#31211=DIRECTION('ref_axis',(0.,0.707106781186542,-0.707106781186553));
#31212=DIRECTION('center_axis',(-0.707106781186566,0.707106781186529,0.));
#31213=DIRECTION('ref_axis',(0.,0.,1.));
#31214=DIRECTION('',(0.,0.,1.));
#31215=DIRECTION('',(0.707106781186529,0.707106781186566,0.));
#31216=DIRECTION('center_axis',(1.,0.,0.));
#31217=DIRECTION('ref_axis',(0.,0.707106781186543,0.707106781186552));
#31218=DIRECTION('',(0.707106781186573,0.,0.707106781186522));
#31219=DIRECTION('center_axis',(-1.,0.,0.));
#31220=DIRECTION('ref_axis',(0.,0.707106781186543,0.707106781186552));
#31221=DIRECTION('center_axis',(1.,0.,0.));
#31222=DIRECTION('ref_axis',(0.,0.707106781186543,0.707106781186552));
#31223=DIRECTION('center_axis',(-0.707106781186548,0.,0.707106781186548));
#31224=DIRECTION('ref_axis',(0.707106781186548,0.,0.707106781186548));
#31225=DIRECTION('',(0.,-1.,0.));
#31226=DIRECTION('',(0.707106781186548,0.,0.707106781186548));
#31227=DIRECTION('',(0.,1.,0.));
#31228=DIRECTION('center_axis',(1.,0.,0.));
#31229=DIRECTION('ref_axis',(0.,-0.707106781186543,0.707106781186552));
#31230=DIRECTION('',(0.707106781186592,-0.707106781186504,0.));
#31231=DIRECTION('center_axis',(1.,0.,0.));
#31232=DIRECTION('ref_axis',(0.,-0.707106781186543,0.707106781186552));
#31233=DIRECTION('center_axis',(-0.707106781186566,-0.707106781186529,0.));
#31234=DIRECTION('ref_axis',(0.,0.,1.));
#31235=DIRECTION('',(0.,0.,-1.));
#31236=DIRECTION('',(0.,0.,1.));
#31237=DIRECTION('center_axis',(0.,0.,1.));
#31238=DIRECTION('ref_axis',(0.,-1.,0.));
#31239=DIRECTION('',(1.,0.,0.));
#31240=DIRECTION('center_axis',(0.,-1.,0.));
#31241=DIRECTION('ref_axis',(0.,0.,-1.));
#31242=DIRECTION('center_axis',(0.,-1.,0.));
#31243=DIRECTION('ref_axis',(1.,0.,0.));
#31244=DIRECTION('center_axis',(0.,-1.,0.));
#31245=DIRECTION('ref_axis',(1.,0.,0.));
#31246=DIRECTION('center_axis',(0.,-1.,0.));
#31247=DIRECTION('ref_axis',(1.,0.,0.));
#31248=DIRECTION('',(-1.,0.,0.));
#31249=DIRECTION('',(0.,0.,1.));
#31250=DIRECTION('',(1.,0.,0.));
#31251=DIRECTION('',(0.,0.,-1.));
#31252=DIRECTION('',(-1.,0.,0.));
#31253=DIRECTION('',(0.,0.,-1.));
#31254=DIRECTION('',(-1.,0.,0.));
#31255=DIRECTION('',(0.,0.,1.));
#31256=DIRECTION('',(1.,0.,0.));
#31257=DIRECTION('',(0.,0.,-1.));
#31258=DIRECTION('',(-1.,0.,0.));
#31259=DIRECTION('',(-0.996744950321709,0.,0.0806195014135826));
#31260=DIRECTION('',(-1.,0.,0.));
#31261=DIRECTION('',(0.,0.,1.));
#31262=DIRECTION('',(1.,0.,0.));
#31263=DIRECTION('',(0.562642705730145,0.,-0.826700178836718));
#31264=DIRECTION('',(0.,0.,1.));
#31265=DIRECTION('',(1.,0.,0.));
#31266=DIRECTION('',(0.,0.,-1.));
#31267=DIRECTION('',(-1.,0.,0.));
#31268=DIRECTION('',(-0.563462182256227,0.,0.826141857774468));
#31269=DIRECTION('',(0.,0.,-1.));
#31270=DIRECTION('center_axis',(1.,0.,0.));
#31271=DIRECTION('ref_axis',(0.,0.,-1.));
#31272=DIRECTION('',(0.,0.,1.));
#31273=DIRECTION('center_axis',(-1.,0.,0.));
#31274=DIRECTION('ref_axis',(0.,-0.707106781186566,-0.707106781186529));
#31275=DIRECTION('',(0.,-1.,0.));
#31276=DIRECTION('center_axis',(-1.,0.,0.));
#31277=DIRECTION('ref_axis',(0.,0.707106781186568,-0.707106781186527));
#31278=DIRECTION('',(0.,0.,-1.));
#31279=DIRECTION('center_axis',(-1.,0.,0.));
#31280=DIRECTION('ref_axis',(0.,0.707106781186568,0.707106781186527));
#31281=DIRECTION('',(0.,1.,0.));
#31282=DIRECTION('center_axis',(-1.,0.,0.));
#31283=DIRECTION('ref_axis',(0.,-0.707106781186568,0.707106781186527));
#31284=DIRECTION('center_axis',(0.,-1.,0.));
#31285=DIRECTION('ref_axis',(-1.83697019872103E-16,0.,1.));
#31286=DIRECTION('',(0.315789473684196,0.707106781186531,0.632674488430095));
#31287=DIRECTION('center_axis',(0.,1.,0.));
#31288=DIRECTION('ref_axis',(1.,0.,0.));
#31289=DIRECTION('center_axis',(0.,1.,0.));
#31290=DIRECTION('ref_axis',(1.,0.,0.));
#31291=DIRECTION('',(0.315789473684196,-0.707106781186531,-0.632674488430095));
#31292=DIRECTION('',(-0.238798209365739,-0.687106448937468,-0.686192497067885));
#31293=DIRECTION('',(-0.238798209365764,0.687106448937464,0.686192497067881));
#31294=DIRECTION('center_axis',(0.,1.,0.));
#31295=DIRECTION('ref_axis',(1.,0.,0.));
#31296=DIRECTION('',(0.,1.,0.));
#31297=DIRECTION('center_axis',(0.,-1.,0.));
#31298=DIRECTION('ref_axis',(1.,0.,0.));
#31299=DIRECTION('center_axis',(0.,-1.,0.));
#31300=DIRECTION('ref_axis',(1.,0.,0.));
#31301=DIRECTION('center_axis',(0.,-1.,0.));
#31302=DIRECTION('ref_axis',(6.12323399573677E-17,0.,-1.));
#31303=DIRECTION('',(-0.315789473684196,0.707106781186531,-0.632674488430095));
#31304=DIRECTION('center_axis',(0.,1.,0.));
#31305=DIRECTION('ref_axis',(1.,0.,0.));
#31306=DIRECTION('center_axis',(0.,1.,0.));
#31307=DIRECTION('ref_axis',(1.,0.,0.));
#31308=DIRECTION('',(-0.315789473684196,-0.707106781186531,0.632674488430095));
#31309=DIRECTION('',(0.238798209365739,-0.687106448937468,0.686192497067885));
#31310=DIRECTION('',(0.238798209365798,0.687106448937561,-0.686192497067771));
#31311=DIRECTION('center_axis',(0.,1.,0.));
#31312=DIRECTION('ref_axis',(1.,0.,0.));
#31313=DIRECTION('',(0.,1.,0.));
#31314=DIRECTION('center_axis',(0.,-1.,0.));
#31315=DIRECTION('ref_axis',(1.,0.,0.));
#31316=DIRECTION('center_axis',(0.,-1.,0.));
#31317=DIRECTION('ref_axis',(1.,0.,0.));
#31318=DIRECTION('center_axis',(-0.707106781186541,0.707106781186554,0.));
#31319=DIRECTION('ref_axis',(0.,0.,1.));
#31320=DIRECTION('',(0.707106781186554,0.707106781186541,0.));
#31321=DIRECTION('',(0.,0.,-1.));
#31322=DIRECTION('',(-0.707106781186554,-0.707106781186541,0.));
#31323=DIRECTION('center_axis',(-1.,0.,0.));
#31324=DIRECTION('ref_axis',(0.,-0.707106781186568,0.707106781186527));
#31325=DIRECTION('',(0.707106781186673,0.,-0.707106781186422));
#31326=DIRECTION('center_axis',(1.,0.,0.));
#31327=DIRECTION('ref_axis',(0.,-0.707106781186568,0.707106781186527));
#31328=DIRECTION('center_axis',(-0.707106781186522,0.,-0.707106781186573));
#31329=DIRECTION('ref_axis',(-0.707106781186573,0.,0.707106781186522));
#31330=DIRECTION('',(0.707106781186573,0.,-0.707106781186522));
#31331=DIRECTION('',(0.,-1.,0.));
#31332=DIRECTION('center_axis',(-1.,0.,0.));
#31333=DIRECTION('ref_axis',(0.,0.707106781186568,0.707106781186527));
#31334=DIRECTION('',(0.707106781186607,-0.707106781186488,0.));
#31335=DIRECTION('center_axis',(1.,0.,0.));
#31336=DIRECTION('ref_axis',(0.,0.707106781186568,0.707106781186527));
#31337=DIRECTION('center_axis',(-0.707106781186541,-0.707106781186554,0.));
#31338=DIRECTION('ref_axis',(0.,0.,1.));
#31339=DIRECTION('',(0.707106781186554,-0.707106781186541,0.));
#31340=DIRECTION('center_axis',(-1.,0.,0.));
#31341=DIRECTION('ref_axis',(0.,0.707106781186568,-0.707106781186527));
#31342=DIRECTION('',(0.707106781186673,0.,0.707106781186422));
#31343=DIRECTION('center_axis',(1.,0.,0.));
#31344=DIRECTION('ref_axis',(0.,0.707106781186568,-0.707106781186527));
#31345=DIRECTION('center_axis',(-0.707106781186522,0.,0.707106781186573));
#31346=DIRECTION('ref_axis',(0.707106781186573,0.,0.707106781186522));
#31347=DIRECTION('',(0.707106781186573,0.,0.707106781186522));
#31348=DIRECTION('',(0.,1.,0.));
#31349=DIRECTION('center_axis',(-1.,0.,0.));
#31350=DIRECTION('ref_axis',(0.,-0.707106781186566,-0.707106781186529));
#31351=DIRECTION('center_axis',(1.,0.,0.));
#31352=DIRECTION('ref_axis',(0.,-0.707106781186566,-0.707106781186529));
#31353=DIRECTION('center_axis',(1.,0.,0.));
#31354=DIRECTION('ref_axis',(0.,0.707106781186568,-0.707106781186527));
#31355=DIRECTION('',(1.,0.,0.));
#31356=DIRECTION('center_axis',(-1.,0.,0.));
#31357=DIRECTION('ref_axis',(0.,0.707106781186568,-0.707106781186527));
#31358=DIRECTION('center_axis',(0.,0.,1.));
#31359=DIRECTION('ref_axis',(0.,-1.,0.));
#31360=DIRECTION('',(-1.,0.,0.));
#31361=DIRECTION('',(0.,-1.,0.));
#31362=DIRECTION('center_axis',(1.,0.,0.));
#31363=DIRECTION('ref_axis',(0.,-0.707106781186566,-0.707106781186529));
#31364=DIRECTION('',(1.,0.,0.));
#31365=DIRECTION('',(1.,0.,0.));
#31366=DIRECTION('',(1.,0.,0.));
#31367=DIRECTION('center_axis',(-1.,0.,0.));
#31368=DIRECTION('ref_axis',(0.,-0.707106781186566,-0.707106781186529));
#31369=DIRECTION('center_axis',(0.,1.,0.));
#31370=DIRECTION('ref_axis',(0.,0.,1.));
#31371=DIRECTION('',(-1.,0.,0.));
#31372=DIRECTION('center_axis',(0.,1.,0.));
#31373=DIRECTION('ref_axis',(1.,0.,0.));
#31374=DIRECTION('',(-1.,0.,0.));
#31375=DIRECTION('center_axis',(0.,1.,0.));
#31376=DIRECTION('ref_axis',(1.,0.,0.));
#31377=DIRECTION('',(-1.,0.,0.));
#31378=DIRECTION('',(0.,0.,1.));
#31379=DIRECTION('center_axis',(0.,1.,0.));
#31380=DIRECTION('ref_axis',(1.,0.,0.));
#31381=DIRECTION('center_axis',(0.,1.,0.));
#31382=DIRECTION('ref_axis',(1.,0.,0.));
#31383=DIRECTION('',(0.373458905374385,-0.737256835467264,0.563010483519946));
#31384=DIRECTION('',(-0.373458905374355,-0.737256835467348,0.563010483519854));
#31385=DIRECTION('center_axis',(0.,1.,0.));
#31386=DIRECTION('ref_axis',(6.12323399573677E-17,0.,1.));
#31387=DIRECTION('',(-0.43401111848607,-0.707106781186588,0.558242195673539));
#31388=DIRECTION('',(-0.43401111848607,0.707106781186588,-0.558242195673539));
#31389=DIRECTION('center_axis',(0.707106781186566,0.707106781186529,0.));
#31390=DIRECTION('ref_axis',(0.,0.,-1.));
#31391=DIRECTION('',(0.707106781186529,-0.707106781186566,0.));
#31392=DIRECTION('',(-0.707106781186529,0.707106781186566,0.));
#31393=DIRECTION('center_axis',(1.,0.,0.));
#31394=DIRECTION('ref_axis',(0.,-0.707106781186568,0.707106781186527));
#31395=DIRECTION('center_axis',(-1.,0.,0.));
#31396=DIRECTION('ref_axis',(0.,-0.707106781186568,0.707106781186527));
#31397=DIRECTION('',(0.707106781186648,0.,0.707106781186447));
#31398=DIRECTION('center_axis',(0.707106781186548,0.,-0.707106781186548));
#31399=DIRECTION('ref_axis',(-0.707106781186548,0.,-0.707106781186548));
#31400=DIRECTION('',(0.707106781186548,0.,0.707106781186548));
#31401=DIRECTION('',(0.,1.,0.));
#31402=DIRECTION('center_axis',(1.,0.,0.));
#31403=DIRECTION('ref_axis',(0.,0.707106781186568,0.707106781186527));
#31404=DIRECTION('center_axis',(-1.,0.,0.));
#31405=DIRECTION('ref_axis',(0.,0.707106781186568,0.707106781186527));
#31406=DIRECTION('',(0.707106781186582,0.707106781186513,0.));
#31407=DIRECTION('center_axis',(0.707106781186566,-0.707106781186529,0.));
#31408=DIRECTION('ref_axis',(0.,0.,-1.));
#31409=DIRECTION('',(0.707106781186529,0.707106781186566,0.));
#31410=DIRECTION('center_axis',(1.,0.,0.));
#31411=DIRECTION('ref_axis',(0.,0.707106781186568,-0.707106781186527));
#31412=DIRECTION('',(0.707106781186648,0.,-0.707106781186447));
#31413=DIRECTION('center_axis',(0.707106781186548,0.,0.707106781186548));
#31414=DIRECTION('ref_axis',(0.707106781186548,0.,-0.707106781186548));
#31415=DIRECTION('',(0.707106781186548,0.,-0.707106781186548));
#31416=DIRECTION('center_axis',(1.,0.,0.));
#31417=DIRECTION('ref_axis',(0.,-0.707106781186566,-0.707106781186529));
#31418=DIRECTION('center_axis',(1.,0.,0.));
#31419=DIRECTION('ref_axis',(0.,0.707106781186568,0.707106781186527));
#31420=DIRECTION('',(-1.,0.,0.));
#31421=DIRECTION('center_axis',(0.,0.,-1.));
#31422=DIRECTION('ref_axis',(0.,1.,0.));
#31423=DIRECTION('',(1.,0.,0.));
#31424=DIRECTION('center_axis',(1.,0.,0.));
#31425=DIRECTION('ref_axis',(0.,-0.707106781186568,0.707106781186527));
#31426=DIRECTION('',(-0.373458905374326,-0.737256835467278,-0.563010483519966));
#31427=DIRECTION('',(0.373458905374459,-0.737256835467315,-0.563010483519829));
#31428=DIRECTION('center_axis',(0.,1.,0.));
#31429=DIRECTION('ref_axis',(-1.83697019872103E-16,0.,-1.));
#31430=DIRECTION('',(0.43401111848607,-0.707106781186588,-0.558242195673539));
#31431=DIRECTION('',(0.43401111848607,0.707106781186588,0.558242195673539));
#31432=DIRECTION('',(-0.373458905374367,-0.737256835467265,-0.563010483519956));
#31433=DIRECTION('',(0.373458905374397,-0.737256835467335,-0.563010483519844));
#31434=DIRECTION('center_axis',(0.,1.,0.));
#31435=DIRECTION('ref_axis',(-1.83697019872103E-16,0.,-1.));
#31436=DIRECTION('',(0.43401111848607,-0.707106781186588,-0.558242195673539));
#31437=DIRECTION('',(0.43401111848607,0.707106781186588,0.558242195673539));
#31438=DIRECTION('center_axis',(0.,-1.,0.));
#31439=DIRECTION('ref_axis',(-1.83697019872103E-16,0.,1.));
#31440=DIRECTION('',(0.315789473684196,0.707106781186531,0.632674488430095));
#31441=DIRECTION('center_axis',(0.,1.,0.));
#31442=DIRECTION('ref_axis',(1.,0.,0.));
#31443=DIRECTION('center_axis',(0.,1.,0.));
#31444=DIRECTION('ref_axis',(1.,0.,0.));
#31445=DIRECTION('',(0.315789473684196,-0.707106781186531,-0.632674488430095));
#31446=DIRECTION('',(-0.238798209365739,-0.687106448937468,-0.686192497067885));
#31447=DIRECTION('',(-0.23879820936573,0.687106448937366,0.68619249706799));
#31448=DIRECTION('center_axis',(0.,1.,0.));
#31449=DIRECTION('ref_axis',(1.,0.,0.));
#31450=DIRECTION('',(0.,1.,0.));
#31451=DIRECTION('center_axis',(0.,-1.,0.));
#31452=DIRECTION('ref_axis',(1.,0.,0.));
#31453=DIRECTION('center_axis',(0.,-1.,0.));
#31454=DIRECTION('ref_axis',(1.,0.,0.));
#31455=DIRECTION('',(0.373458905374429,-0.737256835467245,0.56301048351994));
#31456=DIRECTION('',(-0.373458905374459,-0.737256835467315,0.563010483519829));
#31457=DIRECTION('center_axis',(0.,1.,0.));
#31458=DIRECTION('ref_axis',(6.12323399573677E-17,0.,1.));
#31459=DIRECTION('',(-0.43401111848607,-0.707106781186588,0.558242195673539));
#31460=DIRECTION('',(-0.43401111848607,0.707106781186588,-0.558242195673539));
#31461=DIRECTION('center_axis',(1.,0.,0.));
#31462=DIRECTION('ref_axis',(0.,0.707106781186543,-0.707106781186552));
#31463=DIRECTION('',(0.707106781186592,0.707106781186504,0.));
#31464=DIRECTION('center_axis',(-1.,0.,0.));
#31465=DIRECTION('ref_axis',(0.,0.707106781186543,-0.707106781186552));
#31466=DIRECTION('',(-0.707106781186573,0.,0.707106781186522));
#31467=DIRECTION('center_axis',(1.,0.,0.));
#31468=DIRECTION('ref_axis',(0.,0.707106781186543,-0.707106781186552));
#31469=DIRECTION('center_axis',(-0.707106781186541,0.707106781186554,0.));
#31470=DIRECTION('ref_axis',(0.,0.,1.));
#31471=DIRECTION('',(0.707106781186554,0.707106781186541,0.));
#31472=DIRECTION('',(0.,0.,-1.));
#31473=DIRECTION('',(0.,0.,1.));
#31474=DIRECTION('center_axis',(1.,0.,0.));
#31475=DIRECTION('ref_axis',(0.,0.707106781186543,0.707106781186552));
#31476=DIRECTION('',(0.707106781186573,0.,0.707106781186522));
#31477=DIRECTION('center_axis',(-1.,0.,0.));
#31478=DIRECTION('ref_axis',(0.,0.707106781186543,0.707106781186552));
#31479=DIRECTION('center_axis',(1.,0.,0.));
#31480=DIRECTION('ref_axis',(0.,0.707106781186543,0.707106781186552));
#31481=DIRECTION('center_axis',(-0.707106781186623,0.,0.707106781186472));
#31482=DIRECTION('ref_axis',(0.707106781186472,0.,0.707106781186623));
#31483=DIRECTION('',(0.707106781186472,0.,0.707106781186623));
#31484=DIRECTION('',(0.,1.,0.));
#31485=DIRECTION('',(0.,-1.,0.));
#31486=DIRECTION('center_axis',(1.,0.,0.));
#31487=DIRECTION('ref_axis',(0.,-0.707106781186542,0.707106781186553));
#31488=DIRECTION('',(0.707106781186592,-0.707106781186504,0.));
#31489=DIRECTION('center_axis',(-1.,0.,0.));
#31490=DIRECTION('ref_axis',(0.,-0.707106781186542,0.707106781186553));
#31491=DIRECTION('center_axis',(1.,0.,0.));
#31492=DIRECTION('ref_axis',(0.,-0.707106781186542,0.707106781186553));
#31493=DIRECTION('center_axis',(-0.707106781186541,-0.707106781186554,0.));
#31494=DIRECTION('ref_axis',(0.,0.,1.));
#31495=DIRECTION('',(0.707106781186554,-0.707106781186541,0.));
#31496=DIRECTION('',(0.,0.,-1.));
#31497=DIRECTION('center_axis',(1.,0.,0.));
#31498=DIRECTION('ref_axis',(0.,-0.707106781186543,-0.707106781186552));
#31499=DIRECTION('',(0.707106781186573,0.,-0.707106781186522));
#31500=DIRECTION('center_axis',(-1.,0.,0.));
#31501=DIRECTION('ref_axis',(0.,-0.707106781186543,-0.707106781186552));
#31502=DIRECTION('center_axis',(1.,0.,0.));
#31503=DIRECTION('ref_axis',(0.,-0.707106781186543,-0.707106781186552));
#31504=DIRECTION('center_axis',(-0.707106781186623,0.,-0.707106781186472));
#31505=DIRECTION('ref_axis',(-0.707106781186472,0.,0.707106781186623));
#31506=DIRECTION('',(0.,-1.,0.));
#31507=DIRECTION('',(0.,1.,0.));
#31508=DIRECTION('center_axis',(1.,0.,0.));
#31509=DIRECTION('ref_axis',(0.,-0.707106781186543,-0.707106781186552));
#31510=DIRECTION('',(1.,0.,0.));
#31511=DIRECTION('',(1.,0.,0.));
#31512=DIRECTION('',(1.,0.,0.));
#31513=DIRECTION('center_axis',(1.,0.,0.));
#31514=DIRECTION('ref_axis',(0.,-0.707106781186543,-0.707106781186552));
#31515=DIRECTION('center_axis',(0.,0.,-1.));
#31516=DIRECTION('ref_axis',(0.,1.,0.));
#31517=DIRECTION('',(-1.,0.,0.));
#31518=DIRECTION('',(0.,-1.,0.));
#31519=DIRECTION('center_axis',(1.,0.,0.));
#31520=DIRECTION('ref_axis',(0.,0.707106781186543,-0.707106781186552));
#31521=DIRECTION('',(1.,0.,0.));
#31522=DIRECTION('',(1.,0.,0.));
#31523=DIRECTION('',(1.,0.,0.));
#31524=DIRECTION('center_axis',(1.,0.,0.));
#31525=DIRECTION('ref_axis',(0.,0.707106781186543,-0.707106781186552));
#31526=DIRECTION('',(-1.,0.,0.));
#31527=DIRECTION('',(-1.,0.,0.));
#31528=DIRECTION('center_axis',(1.,0.,0.));
#31529=DIRECTION('ref_axis',(0.,0.,-1.));
#31530=DIRECTION('',(0.,0.,-1.));
#31531=DIRECTION('center_axis',(-1.,0.,0.));
#31532=DIRECTION('ref_axis',(0.,0.707106781186566,0.707106781186529));
#31533=DIRECTION('',(0.,1.,0.));
#31534=DIRECTION('center_axis',(-1.,0.,0.));
#31535=DIRECTION('ref_axis',(0.,-0.707106781186568,0.707106781186527));
#31536=DIRECTION('',(0.,0.,1.));
#31537=DIRECTION('center_axis',(-1.,0.,0.));
#31538=DIRECTION('ref_axis',(0.,-0.707106781186568,-0.707106781186527));
#31539=DIRECTION('',(0.,-1.,0.));
#31540=DIRECTION('center_axis',(-1.,0.,0.));
#31541=DIRECTION('ref_axis',(0.,0.707106781186568,-0.707106781186527));
#31542=DIRECTION('center_axis',(-1.,0.,0.));
#31543=DIRECTION('ref_axis',(0.,0.707106781186543,-0.707106781186552));
#31544=DIRECTION('',(-0.707106781186548,0.,-0.707106781186548));
#31545=DIRECTION('',(0.707106781186566,-0.707106781186529,0.));
#31546=DIRECTION('center_axis',(-1.,0.,0.));
#31547=DIRECTION('ref_axis',(0.,0.707106781186543,-0.707106781186552));
#31548=DIRECTION('center_axis',(0.707106781186548,0.,-0.707106781186548));
#31549=DIRECTION('ref_axis',(-0.707106781186548,0.,-0.707106781186548));
#31550=DIRECTION('',(0.,-1.,0.));
#31551=DIRECTION('',(-0.707106781186548,0.,-0.707106781186548));
#31552=DIRECTION('',(0.,1.,0.));
#31553=DIRECTION('center_axis',(-1.,0.,0.));
#31554=DIRECTION('ref_axis',(0.,-0.707106781186543,-0.707106781186552));
#31555=DIRECTION('',(-0.707106781186566,-0.707106781186529,0.));
#31556=DIRECTION('center_axis',(-1.,0.,0.));
#31557=DIRECTION('ref_axis',(0.,-0.707106781186543,-0.707106781186552));
#31558=DIRECTION('center_axis',(0.707106781186566,-0.707106781186529,0.));
#31559=DIRECTION('ref_axis',(0.,0.,-1.));
#31560=DIRECTION('',(0.,0.,1.));
#31561=DIRECTION('',(-0.707106781186529,-0.707106781186566,0.));
#31562=DIRECTION('center_axis',(-1.,0.,0.));
#31563=DIRECTION('ref_axis',(0.,-0.707106781186542,0.707106781186553));
#31564=DIRECTION('',(-0.707106781186548,0.,0.707106781186548));
#31565=DIRECTION('center_axis',(1.,0.,0.));
#31566=DIRECTION('ref_axis',(0.,-0.707106781186542,0.707106781186553));
#31567=DIRECTION('center_axis',(-1.,0.,0.));
#31568=DIRECTION('ref_axis',(0.,-0.707106781186542,0.707106781186553));
#31569=DIRECTION('center_axis',(0.707106781186548,0.,0.707106781186548));
#31570=DIRECTION('ref_axis',(0.707106781186548,0.,-0.707106781186548));
#31571=DIRECTION('',(0.,1.,0.));
#31572=DIRECTION('',(-0.707106781186548,0.,0.707106781186548));
#31573=DIRECTION('',(0.,-1.,0.));
#31574=DIRECTION('center_axis',(-1.,0.,0.));
#31575=DIRECTION('ref_axis',(0.,0.707106781186543,0.707106781186552));
#31576=DIRECTION('',(-0.707106781186566,0.707106781186529,0.));
#31577=DIRECTION('center_axis',(1.,0.,0.));
#31578=DIRECTION('ref_axis',(0.,0.707106781186543,0.707106781186552));
#31579=DIRECTION('center_axis',(-1.,0.,0.));
#31580=DIRECTION('ref_axis',(0.,0.707106781186543,0.707106781186552));
#31581=DIRECTION('center_axis',(0.707106781186566,0.707106781186529,0.));
#31582=DIRECTION('ref_axis',(0.,0.,-1.));
#31583=DIRECTION('',(0.,0.,-1.));
#31584=DIRECTION('',(0.,0.,1.));
#31585=DIRECTION('center_axis',(0.,0.,1.));
#31586=DIRECTION('ref_axis',(0.,-1.,0.));
#31587=DIRECTION('',(-1.,0.,0.));
#31588=DIRECTION('',(1.,0.,0.));
#31589=DIRECTION('center_axis',(1.,0.,0.));
#31590=DIRECTION('ref_axis',(0.,0.707106781186543,0.707106781186552));
#31591=DIRECTION('',(-1.,0.,0.));
#31592=DIRECTION('',(-1.,0.,0.));
#31593=DIRECTION('',(-1.,0.,0.));
#31594=DIRECTION('center_axis',(0.,1.,0.));
#31595=DIRECTION('ref_axis',(0.,0.,1.));
#31596=DIRECTION('center_axis',(0.,1.,0.));
#31597=DIRECTION('ref_axis',(1.,0.,0.));
#31598=DIRECTION('center_axis',(0.,1.,0.));
#31599=DIRECTION('ref_axis',(1.,0.,0.));
#31600=DIRECTION('center_axis',(0.,1.,0.));
#31601=DIRECTION('ref_axis',(1.,0.,0.));
#31602=DIRECTION('center_axis',(0.,1.,0.));
#31603=DIRECTION('ref_axis',(1.,0.,0.));
#31604=DIRECTION('center_axis',(1.,0.,0.));
#31605=DIRECTION('ref_axis',(0.,0.,-1.));
#31606=DIRECTION('',(0.,0.,1.));
#31607=DIRECTION('center_axis',(1.,0.,0.));
#31608=DIRECTION('ref_axis',(0.,0.707106781186568,-0.707106781186527));
#31609=DIRECTION('',(0.,1.,0.));
#31610=DIRECTION('center_axis',(1.,0.,0.));
#31611=DIRECTION('ref_axis',(0.,-0.707106781186568,-0.707106781186527));
#31612=DIRECTION('',(0.,0.,-1.));
#31613=DIRECTION('center_axis',(1.,0.,0.));
#31614=DIRECTION('ref_axis',(0.,-0.707106781186568,0.707106781186527));
#31615=DIRECTION('',(0.,-1.,0.));
#31616=DIRECTION('center_axis',(1.,0.,0.));
#31617=DIRECTION('ref_axis',(0.,0.707106781186566,0.707106781186529));
#31618=DIRECTION('',(-0.238798209365737,0.687106448937475,0.686192497067879));
#31619=DIRECTION('',(-0.238798209365775,-0.687106448937559,-0.686192497067782));
#31620=DIRECTION('center_axis',(0.,1.,0.));
#31621=DIRECTION('ref_axis',(-1.83697019872103E-16,0.,-1.));
#31622=DIRECTION('',(0.315789473684196,-0.707106781186531,-0.632674488430095));
#31623=DIRECTION('center_axis',(0.,-1.,0.));
#31624=DIRECTION('ref_axis',(1.,0.,0.));
#31625=DIRECTION('center_axis',(0.,-1.,0.));
#31626=DIRECTION('ref_axis',(1.,0.,0.));
#31627=DIRECTION('',(0.315789473684196,0.707106781186531,0.632674488430095));
#31628=DIRECTION('center_axis',(0.,-1.,0.));
#31629=DIRECTION('ref_axis',(1.,0.,0.));
#31630=DIRECTION('',(0.,-1.,0.));
#31631=DIRECTION('center_axis',(0.,1.,0.));
#31632=DIRECTION('ref_axis',(1.,0.,0.));
#31633=DIRECTION('center_axis',(0.,1.,0.));
#31634=DIRECTION('ref_axis',(1.,0.,0.));
#31635=DIRECTION('center_axis',(0.707106781186566,-0.707106781186529,0.));
#31636=DIRECTION('ref_axis',(0.,0.,-1.));
#31637=DIRECTION('',(0.707106781186529,0.707106781186566,0.));
#31638=DIRECTION('',(-0.707106781186529,-0.707106781186566,0.));
#31639=DIRECTION('',(0.,0.,-1.));
#31640=DIRECTION('center_axis',(1.,0.,0.));
#31641=DIRECTION('ref_axis',(0.,0.707106781186568,-0.707106781186527));
#31642=DIRECTION('center_axis',(-1.,0.,0.));
#31643=DIRECTION('ref_axis',(0.,0.707106781186568,-0.707106781186527));
#31644=DIRECTION('',(0.707106781186648,0.,-0.707106781186447));
#31645=DIRECTION('center_axis',(0.707106781186548,0.,0.707106781186548));
#31646=DIRECTION('ref_axis',(0.707106781186548,0.,-0.707106781186548));
#31647=DIRECTION('',(0.707106781186548,0.,-0.707106781186548));
#31648=DIRECTION('',(0.,-1.,0.));
#31649=DIRECTION('center_axis',(1.,0.,0.));
#31650=DIRECTION('ref_axis',(0.,-0.707106781186568,-0.707106781186527));
#31651=DIRECTION('center_axis',(-1.,0.,0.));
#31652=DIRECTION('ref_axis',(0.,-0.707106781186568,-0.707106781186527));
#31653=DIRECTION('',(0.707106781186582,-0.707106781186513,0.));
#31654=DIRECTION('center_axis',(0.707106781186566,0.707106781186529,0.));
#31655=DIRECTION('ref_axis',(0.,0.,-1.));
#31656=DIRECTION('',(0.707106781186529,-0.707106781186566,0.));
#31657=DIRECTION('center_axis',(1.,0.,0.));
#31658=DIRECTION('ref_axis',(0.,-0.707106781186568,0.707106781186527));
#31659=DIRECTION('center_axis',(-1.,0.,0.));
#31660=DIRECTION('ref_axis',(0.,-0.707106781186568,0.707106781186527));
#31661=DIRECTION('',(0.707106781186648,0.,0.707106781186447));
#31662=DIRECTION('center_axis',(0.707106781186548,0.,-0.707106781186548));
#31663=DIRECTION('ref_axis',(-0.707106781186548,0.,-0.707106781186548));
#31664=DIRECTION('',(0.707106781186548,0.,0.707106781186548));
#31665=DIRECTION('',(0.,1.,0.));
#31666=DIRECTION('center_axis',(1.,0.,0.));
#31667=DIRECTION('ref_axis',(0.,0.707106781186566,0.707106781186529));
#31668=DIRECTION('center_axis',(-1.,0.,0.));
#31669=DIRECTION('ref_axis',(0.,0.707106781186566,0.707106781186529));
#31670=DIRECTION('center_axis',(1.,0.,0.));
#31671=DIRECTION('ref_axis',(0.,-0.707106781186568,-0.707106781186527));
#31672=DIRECTION('',(-1.,0.,0.));
#31673=DIRECTION('center_axis',(1.,0.,0.));
#31674=DIRECTION('ref_axis',(0.,-0.707106781186568,-0.707106781186527));
#31675=DIRECTION('center_axis',(0.,0.,1.));
#31676=DIRECTION('ref_axis',(0.,-1.,0.));
#31677=DIRECTION('',(1.,0.,0.));
#31678=DIRECTION('',(0.,1.,0.));
#31679=DIRECTION('center_axis',(1.,0.,0.));
#31680=DIRECTION('ref_axis',(0.,0.707106781186568,-0.707106781186527));
#31681=DIRECTION('',(-1.,0.,0.));
#31682=DIRECTION('',(-1.,0.,0.));
#31683=DIRECTION('',(-1.,0.,0.));
#31684=DIRECTION('center_axis',(1.,0.,0.));
#31685=DIRECTION('ref_axis',(0.,0.707106781186568,-0.707106781186527));
#31686=DIRECTION('center_axis',(0.,-1.,0.));
#31687=DIRECTION('ref_axis',(0.,0.,-1.));
#31688=DIRECTION('',(1.,0.,0.));
#31689=DIRECTION('center_axis',(0.,-1.,0.));
#31690=DIRECTION('ref_axis',(1.,0.,0.));
#31691=DIRECTION('',(1.,0.,0.));
#31692=DIRECTION('center_axis',(0.,-1.,0.));
#31693=DIRECTION('ref_axis',(1.,0.,0.));
#31694=DIRECTION('',(1.,0.,0.));
#31695=DIRECTION('',(0.,0.,1.));
#31696=DIRECTION('center_axis',(0.,-1.,0.));
#31697=DIRECTION('ref_axis',(1.,0.,0.));
#31698=DIRECTION('center_axis',(0.,-1.,0.));
#31699=DIRECTION('ref_axis',(1.,0.,0.));
#31700=DIRECTION('center_axis',(-0.707106781186541,-0.707106781186554,0.));
#31701=DIRECTION('ref_axis',(0.,0.,1.));
#31702=DIRECTION('',(0.707106781186554,-0.707106781186541,0.));
#31703=DIRECTION('',(-0.707106781186554,0.707106781186541,0.));
#31704=DIRECTION('center_axis',(-1.,0.,0.));
#31705=DIRECTION('ref_axis',(0.,0.707106781186568,-0.707106781186527));
#31706=DIRECTION('',(0.707106781186673,0.,0.707106781186422));
#31707=DIRECTION('center_axis',(-0.707106781186522,0.,0.707106781186573));
#31708=DIRECTION('ref_axis',(0.707106781186573,0.,0.707106781186522));
#31709=DIRECTION('',(0.707106781186573,0.,0.707106781186522));
#31710=DIRECTION('center_axis',(-1.,0.,0.));
#31711=DIRECTION('ref_axis',(0.,-0.707106781186568,-0.707106781186527));
#31712=DIRECTION('',(0.707106781186607,0.707106781186488,0.));
#31713=DIRECTION('center_axis',(-0.707106781186541,0.707106781186554,0.));
#31714=DIRECTION('ref_axis',(0.,0.,1.));
#31715=DIRECTION('',(0.707106781186554,0.707106781186541,0.));
#31716=DIRECTION('center_axis',(-1.,0.,0.));
#31717=DIRECTION('ref_axis',(0.,-0.707106781186568,0.707106781186527));
#31718=DIRECTION('',(0.707106781186673,0.,-0.707106781186422));
#31719=DIRECTION('center_axis',(1.,0.,0.));
#31720=DIRECTION('ref_axis',(0.,-0.707106781186568,0.707106781186527));
#31721=DIRECTION('center_axis',(-0.707106781186522,0.,-0.707106781186573));
#31722=DIRECTION('ref_axis',(-0.707106781186573,0.,0.707106781186522));
#31723=DIRECTION('',(0.707106781186573,0.,-0.707106781186522));
#31724=DIRECTION('',(0.,-1.,0.));
#31725=DIRECTION('center_axis',(-1.,0.,0.));
#31726=DIRECTION('ref_axis',(0.,0.707106781186566,0.707106781186529));
#31727=DIRECTION('center_axis',(1.,0.,0.));
#31728=DIRECTION('ref_axis',(0.,0.707106781186566,0.707106781186529));
#31729=DIRECTION('center_axis',(1.,0.,0.));
#31730=DIRECTION('ref_axis',(0.,-0.707106781186568,0.707106781186527));
#31731=DIRECTION('',(1.,0.,0.));
#31732=DIRECTION('center_axis',(0.,0.,-1.));
#31733=DIRECTION('ref_axis',(0.,1.,0.));
#31734=DIRECTION('',(-1.,0.,0.));
#31735=DIRECTION('center_axis',(1.,0.,0.));
#31736=DIRECTION('ref_axis',(0.,0.707106781186566,0.707106781186529));
#31737=DIRECTION('',(0.373458905374385,0.737256835467264,-0.563010483519946));
#31738=DIRECTION('',(-0.373458905374456,0.73725683546732,-0.563010483519824));
#31739=DIRECTION('center_axis',(0.,-1.,0.));
#31740=DIRECTION('ref_axis',(6.12323399573677E-17,0.,-1.));
#31741=DIRECTION('',(-0.43401111848607,0.707106781186588,-0.558242195673539));
#31742=DIRECTION('',(-0.43401111848607,-0.707106781186588,0.558242195673539));
#31743=DIRECTION('center_axis',(0.,1.,0.));
#31744=DIRECTION('ref_axis',(6.12323399573677E-17,0.,1.));
#31745=DIRECTION('',(-0.315789473684196,-0.707106781186531,0.632674488430095));
#31746=DIRECTION('center_axis',(0.,-1.,0.));
#31747=DIRECTION('ref_axis',(1.,0.,0.));
#31748=DIRECTION('center_axis',(0.,-1.,0.));
#31749=DIRECTION('ref_axis',(1.,0.,0.));
#31750=DIRECTION('',(-0.315789473684196,0.707106781186531,-0.632674488430095));
#31751=DIRECTION('',(0.238798209365739,0.687106448937468,-0.686192497067885));
#31752=DIRECTION('',(0.238798209365766,-0.687106448937457,0.686192497067887));
#31753=DIRECTION('center_axis',(0.,-1.,0.));
#31754=DIRECTION('ref_axis',(1.,0.,0.));
#31755=DIRECTION('',(0.,-1.,0.));
#31756=DIRECTION('center_axis',(0.,1.,0.));
#31757=DIRECTION('ref_axis',(1.,0.,0.));
#31758=DIRECTION('center_axis',(0.,1.,0.));
#31759=DIRECTION('ref_axis',(1.,0.,0.));
#31760=DIRECTION('',(-0.373458905374388,0.737256835467258,0.563010483519951));
#31761=DIRECTION('',(0.3734589053744,0.737256835467329,0.563010483519849));
#31762=DIRECTION('center_axis',(0.,-1.,0.));
#31763=DIRECTION('ref_axis',(-1.83697019872103E-16,0.,1.));
#31764=DIRECTION('',(0.43401111848607,0.707106781186588,0.558242195673539));
#31765=DIRECTION('',(0.43401111848607,-0.707106781186588,-0.558242195673539));
#31766=DIRECTION('',(-0.238798209365762,0.687106448937471,0.686192497067875));
#31767=DIRECTION('',(-0.238798209365739,-0.687106448937468,-0.686192497067885));
#31768=DIRECTION('center_axis',(0.,1.,0.));
#31769=DIRECTION('ref_axis',(-1.83697019872103E-16,0.,-1.));
#31770=DIRECTION('',(0.315789473684196,-0.707106781186531,-0.632674488430095));
#31771=DIRECTION('center_axis',(0.,-1.,0.));
#31772=DIRECTION('ref_axis',(1.,0.,0.));
#31773=DIRECTION('center_axis',(0.,-1.,0.));
#31774=DIRECTION('ref_axis',(1.,0.,0.));
#31775=DIRECTION('',(0.315789473684196,0.707106781186531,0.632674488430095));
#31776=DIRECTION('center_axis',(0.,-1.,0.));
#31777=DIRECTION('ref_axis',(1.,0.,0.));
#31778=DIRECTION('',(0.,-1.,0.));
#31779=DIRECTION('center_axis',(0.,1.,0.));
#31780=DIRECTION('ref_axis',(1.,0.,0.));
#31781=DIRECTION('center_axis',(0.,1.,0.));
#31782=DIRECTION('ref_axis',(1.,0.,0.));
#31783=DIRECTION('',(0.373458905374343,0.737256835467277,-0.563010483519956));
#31784=DIRECTION('',(-0.373458905374373,0.737256835467347,-0.563010483519844));
#31785=DIRECTION('center_axis',(0.,-1.,0.));
#31786=DIRECTION('ref_axis',(6.12323399573677E-17,0.,-1.));
#31787=DIRECTION('',(-0.43401111848607,0.707106781186588,-0.558242195673539));
#31788=DIRECTION('',(-0.43401111848607,-0.707106781186588,0.558242195673539));
#31789=DIRECTION('center_axis',(0.,1.,0.));
#31790=DIRECTION('ref_axis',(6.12323399573677E-17,0.,1.));
#31791=DIRECTION('',(-0.315789473684196,-0.707106781186531,0.632674488430095));
#31792=DIRECTION('center_axis',(0.,-1.,0.));
#31793=DIRECTION('ref_axis',(1.,0.,0.));
#31794=DIRECTION('center_axis',(0.,-1.,0.));
#31795=DIRECTION('ref_axis',(1.,0.,0.));
#31796=DIRECTION('',(-0.315789473684196,0.707106781186531,-0.632674488430095));
#31797=DIRECTION('',(0.238798209365762,0.687106448937471,-0.686192497067875));
#31798=DIRECTION('',(0.238798209365737,-0.687106448937475,0.686192497067879));
#31799=DIRECTION('center_axis',(0.,-1.,0.));
#31800=DIRECTION('ref_axis',(1.,0.,0.));
#31801=DIRECTION('',(0.,-1.,0.));
#31802=DIRECTION('center_axis',(0.,1.,0.));
#31803=DIRECTION('ref_axis',(1.,0.,0.));
#31804=DIRECTION('center_axis',(0.,1.,0.));
#31805=DIRECTION('ref_axis',(1.,0.,0.));
#31806=DIRECTION('',(-0.373458905374388,0.737256835467258,0.563010483519951));
#31807=DIRECTION('',(0.373458905374438,0.737256835467322,0.563010483519834));
#31808=DIRECTION('center_axis',(0.,-1.,0.));
#31809=DIRECTION('ref_axis',(-1.83697019872103E-16,0.,1.));
#31810=DIRECTION('',(0.43401111848607,0.707106781186588,0.558242195673539));
#31811=DIRECTION('',(0.43401111848607,-0.707106781186588,-0.558242195673539));
#31812=DIRECTION('center_axis',(0.,0.,-1.));
#31813=DIRECTION('ref_axis',(1.,0.,0.));
#31814=DIRECTION('center_axis',(0.,0.,-1.));
#31815=DIRECTION('ref_axis',(1.,0.,0.));
#31816=DIRECTION('',(0.707106781186573,-8.65956056235524E-17,0.707106781186522));
#31817=DIRECTION('center_axis',(0.,0.,1.));
#31818=DIRECTION('ref_axis',(1.,0.,0.));
#31819=DIRECTION('center_axis',(0.,0.,1.));
#31820=DIRECTION('ref_axis',(1.,0.,0.));
#31821=DIRECTION('',(0.,0.,1.));
#31822=DIRECTION('center_axis',(0.,0.,-1.));
#31823=DIRECTION('ref_axis',(1.,0.,0.));
#31824=DIRECTION('center_axis',(0.,0.,1.));
#31825=DIRECTION('ref_axis',(1.,0.,0.));
#31826=DIRECTION('center_axis',(0.,0.,-1.));
#31827=DIRECTION('ref_axis',(1.,0.,0.));
#31828=DIRECTION('center_axis',(0.,0.,1.));
#31829=DIRECTION('ref_axis',(1.,0.,0.));
#31830=DIRECTION('center_axis',(0.,0.,1.));
#31831=DIRECTION('ref_axis',(1.,0.,0.));
#31832=DIRECTION('',(0.707106781186573,8.65956056235524E-17,-0.707106781186522));
#31833=DIRECTION('center_axis',(0.,0.,1.));
#31834=DIRECTION('ref_axis',(1.,0.,0.));
#31835=DIRECTION('',(0.,-1.,0.));
#31836=DIRECTION('center_axis',(0.,0.,1.));
#31837=DIRECTION('ref_axis',(1.,0.,0.));
#31838=DIRECTION('center_axis',(0.,0.,-1.));
#31839=DIRECTION('ref_axis',(1.,0.,0.));
#31840=DIRECTION('',(0.707106781186573,-8.65956056235524E-17,0.707106781186522));
#31841=DIRECTION('center_axis',(0.,0.,1.));
#31842=DIRECTION('ref_axis',(1.,0.,0.));
#31843=DIRECTION('center_axis',(0.,0.,1.));
#31844=DIRECTION('ref_axis',(1.,0.,0.));
#31845=DIRECTION('',(0.,0.,1.));
#31846=DIRECTION('center_axis',(0.,0.,-1.));
#31847=DIRECTION('ref_axis',(1.,0.,0.));
#31848=DIRECTION('center_axis',(0.,0.,1.));
#31849=DIRECTION('ref_axis',(1.,0.,0.));
#31850=DIRECTION('',(0.707106781186573,8.65956056235524E-17,-0.707106781186522));
#31851=DIRECTION('',(0.,1.,0.));
#31852=DIRECTION('',(0.,1.,0.));
#31853=DIRECTION('',(0.,1.,0.));
#31854=DIRECTION('',(0.,1.,0.));
#31855=DIRECTION('',(0.,1.,0.));
#31856=DIRECTION('',(0.,1.,0.));
#31857=DIRECTION('',(0.,1.,0.));
#31858=DIRECTION('',(0.,1.,0.));
#31859=DIRECTION('',(0.,1.,0.));
#31860=DIRECTION('',(0.,1.,0.));
#31861=DIRECTION('',(0.,1.,0.));
#31862=DIRECTION('',(0.,1.,0.));
#31863=DIRECTION('',(0.,1.,0.));
#31864=DIRECTION('',(0.,1.,0.));
#31865=DIRECTION('',(0.,1.,0.));
#31866=DIRECTION('',(0.,1.,0.));
#31867=DIRECTION('',(0.,1.,0.));
#31868=DIRECTION('',(0.,1.,0.));
#31869=DIRECTION('center_axis',(5.78607088678386E-16,1.,-3.04931671898278E-16));
#31870=DIRECTION('ref_axis',(1.,-5.78607088678386E-16,0.));
#31871=DIRECTION('center_axis',(0.,0.,-1.));
#31872=DIRECTION('ref_axis',(-1.,7.44994596638861E-32,0.));
#31873=DIRECTION('',(0.,1.,0.));
#31874=DIRECTION('',(-1.,7.44994596638861E-32,0.));
#31875=DIRECTION('',(0.,1.,0.));
#31876=DIRECTION('center_axis',(-1.,0.,0.));
#31877=DIRECTION('ref_axis',(0.,1.22464679914735E-16,1.));
#31878=DIRECTION('',(0.,1.,0.));
#31879=DIRECTION('',(0.,1.22464679914735E-16,1.));
#31880=DIRECTION('center_axis',(0.,0.,-1.));
#31881=DIRECTION('ref_axis',(-1.,-7.59796397489589E-32,0.));
#31882=DIRECTION('',(0.,1.,0.));
#31883=DIRECTION('',(-1.,-7.59796397489589E-32,0.));
#31884=DIRECTION('center_axis',(1.,0.,0.));
#31885=DIRECTION('ref_axis',(0.,-1.22464679914735E-16,-1.));
#31886=DIRECTION('',(0.,1.,0.));
#31887=DIRECTION('',(0.,-1.22464679914735E-16,-1.));
#31888=DIRECTION('center_axis',(0.,0.,-1.));
#31889=DIRECTION('ref_axis',(-1.,1.86248514964948E-32,0.));
#31890=DIRECTION('',(0.,1.,0.));
#31891=DIRECTION('',(-1.,1.86248514964948E-32,0.));
#31892=DIRECTION('center_axis',(1.,0.,0.));
#31893=DIRECTION('ref_axis',(0.,-1.22464679914735E-16,-1.));
#31894=DIRECTION('',(0.,1.,0.));
#31895=DIRECTION('',(0.,-1.22464679914735E-16,-1.));
#31896=DIRECTION('center_axis',(0.,0.,1.));
#31897=DIRECTION('ref_axis',(1.,0.,0.));
#31898=DIRECTION('',(0.,1.,0.));
#31899=DIRECTION('',(1.,0.,0.));
#31900=DIRECTION('center_axis',(-1.,0.,0.));
#31901=DIRECTION('ref_axis',(0.,1.22464679914735E-16,1.));
#31902=DIRECTION('',(0.,1.22464679914735E-16,1.));
#31903=DIRECTION('center_axis',(0.,1.,0.));
#31904=DIRECTION('ref_axis',(0.,0.,1.));
#31905=DIRECTION('',(0.,1.,0.));
#31906=DIRECTION('',(0.,1.,0.));
#31907=DIRECTION('',(0.,1.,0.));
#31908=DIRECTION('',(0.,1.,0.));
#31909=DIRECTION('',(0.,1.,0.));
#31910=DIRECTION('',(0.,1.,0.));
#31911=DIRECTION('',(0.,1.,0.));
#31912=DIRECTION('',(0.,1.,0.));
#31913=DIRECTION('',(0.,1.,0.));
#31914=DIRECTION('',(0.,1.,0.));
#31915=DIRECTION('',(0.,1.,0.));
#31916=DIRECTION('',(0.,1.,0.));
#31917=DIRECTION('',(0.,1.,0.));
#31918=DIRECTION('',(0.,1.,0.));
#31919=DIRECTION('',(0.,1.,0.));
#31920=DIRECTION('',(0.,1.,0.));
#31921=DIRECTION('',(0.,1.,0.));
#31922=DIRECTION('',(0.,1.,0.));
#31923=DIRECTION('',(0.,1.,0.));
#31924=DIRECTION('',(0.,1.,0.));
#31925=DIRECTION('',(0.,1.,0.));
#31926=DIRECTION('',(0.,1.,0.));
#31927=DIRECTION('center_axis',(6.36041226292982E-16,1.,-2.54585982322281E-16));
#31928=DIRECTION('ref_axis',(1.,-6.36041226292982E-16,0.));
#31929=DIRECTION('center_axis',(0.,0.,1.));
#31930=DIRECTION('ref_axis',(1.,0.,0.));
#31931=DIRECTION('',(0.,1.,0.));
#31932=DIRECTION('',(1.,0.,0.));
#31933=DIRECTION('',(0.,1.,0.));
#31934=DIRECTION('',(0.,1.,0.));
#31935=DIRECTION('',(0.,1.,0.));
#31936=DIRECTION('',(0.,1.,0.));
#31937=DIRECTION('',(0.,1.,0.));
#31938=DIRECTION('',(0.,1.,0.));
#31939=DIRECTION('',(0.,1.,0.));
#31940=DIRECTION('',(0.,1.,0.));
#31941=DIRECTION('',(0.,1.,0.));
#31942=DIRECTION('',(0.,1.,0.));
#31943=DIRECTION('',(0.,1.,0.));
#31944=DIRECTION('center_axis',(-0.0806195014135826,0.,-0.996744950321709));
#31945=DIRECTION('ref_axis',(-0.996744950321709,9.87304143549995E-18,0.0806195014135826));
#31946=DIRECTION('',(0.,1.,0.));
#31947=DIRECTION('',(-0.996744950321709,9.87304143549995E-18,0.0806195014135826));
#31948=DIRECTION('',(0.,1.,0.));
#31949=DIRECTION('',(0.,1.,0.));
#31950=DIRECTION('',(0.,1.,0.));
#31951=DIRECTION('',(0.,1.,0.));
#31952=DIRECTION('',(0.,1.,0.));
#31953=DIRECTION('',(0.,1.,0.));
#31954=DIRECTION('',(0.,1.,0.));
#31955=DIRECTION('',(0.,1.,0.));
#31956=DIRECTION('center_axis',(0.,0.,-1.));
#31957=DIRECTION('ref_axis',(-1.,0.,0.));
#31958=DIRECTION('',(0.,1.,0.));
#31959=DIRECTION('',(-1.,0.,0.));
#31960=DIRECTION('center_axis',(1.,0.,0.));
#31961=DIRECTION('ref_axis',(0.,-1.22464679914735E-16,-1.));
#31962=DIRECTION('',(0.,-1.22464679914735E-16,-1.));
#31963=DIRECTION('center_axis',(1.79916134966616E-15,1.,-7.85768930404053E-16));
#31964=DIRECTION('ref_axis',(1.,-1.79916134966616E-15,0.));
#31965=DIRECTION('center_axis',(0.,0.,-1.));
#31966=DIRECTION('ref_axis',(-1.,-8.07952632620863E-32,0.));
#31967=DIRECTION('',(0.,1.,0.));
#31968=DIRECTION('',(-1.,-8.07952632620863E-32,0.));
#31969=DIRECTION('',(0.,1.,0.));
#31970=DIRECTION('center_axis',(1.,0.,0.));
#31971=DIRECTION('ref_axis',(0.,-1.22464679914735E-16,-1.));
#31972=DIRECTION('',(0.,1.,0.));
#31973=DIRECTION('',(0.,-1.22464679914735E-16,-1.));
#31974=DIRECTION('center_axis',(-0.826141857774468,0.,-0.563462182256227));
#31975=DIRECTION('ref_axis',(-0.563462182256227,1.01173198176515E-16,0.826141857774468));
#31976=DIRECTION('',(0.,1.,0.));
#31977=DIRECTION('',(-0.563462182256227,1.01173198176515E-16,0.826141857774468));
#31978=DIRECTION('center_axis',(0.,0.,-1.));
#31979=DIRECTION('ref_axis',(-1.,-4.03029640013317E-32,0.));
#31980=DIRECTION('',(0.,1.,0.));
#31981=DIRECTION('',(-1.,-4.03029640013317E-32,0.));
#31982=DIRECTION('center_axis',(1.,0.,0.));
#31983=DIRECTION('ref_axis',(0.,-1.22464679914735E-16,-1.));
#31984=DIRECTION('',(0.,1.,0.));
#31985=DIRECTION('',(0.,-1.22464679914735E-16,-1.));
#31986=DIRECTION('center_axis',(0.,0.,1.));
#31987=DIRECTION('ref_axis',(1.,0.,0.));
#31988=DIRECTION('',(0.,1.,0.));
#31989=DIRECTION('',(1.,0.,0.));
#31990=DIRECTION('center_axis',(-1.,0.,0.));
#31991=DIRECTION('ref_axis',(0.,1.22464679914735E-16,1.));
#31992=DIRECTION('',(0.,1.,0.));
#31993=DIRECTION('',(0.,1.22464679914735E-16,1.));
#31994=DIRECTION('center_axis',(0.826700178836718,0.,0.562642705730145));
#31995=DIRECTION('ref_axis',(0.562642705730145,-1.01241572786693E-16,-0.826700178836718));
#31996=DIRECTION('',(0.,1.,0.));
#31997=DIRECTION('',(0.562642705730145,-1.01241572786693E-16,-0.826700178836718));
#31998=DIRECTION('center_axis',(0.,0.,1.));
#31999=DIRECTION('ref_axis',(1.,0.,0.));
#32000=DIRECTION('',(0.,1.,0.));
#32001=DIRECTION('',(1.,0.,0.));
#32002=DIRECTION('center_axis',(-1.,0.,0.));
#32003=DIRECTION('ref_axis',(0.,1.22464679914735E-16,1.));
#32004=DIRECTION('',(0.,1.22464679914735E-16,1.));
#32005=DIRECTION('center_axis',(0.,1.,0.));
#32006=DIRECTION('ref_axis',(0.,0.,1.));
#32007=DIRECTION('center_axis',(0.,-1.,0.));
#32008=DIRECTION('ref_axis',(0.,0.,-1.));
#32009=DIRECTION('center_axis',(0.,-1.,0.));
#32010=DIRECTION('ref_axis',(0.,0.,-1.));
#32011=DIRECTION('center_axis',(0.,0.,1.));
#32012=DIRECTION('ref_axis',(1.,0.,0.));
#32013=DIRECTION('',(0.,-1.,0.));
#32014=DIRECTION('center_axis',(-1.,0.,0.));
#32015=DIRECTION('ref_axis',(0.,-1.,0.));
#32016=DIRECTION('',(0.,-1.,0.));
#32017=DIRECTION('center_axis',(0.,0.,-1.));
#32018=DIRECTION('ref_axis',(0.,1.,0.));
#32019=DIRECTION('center_axis',(1.,0.,0.));
#32020=DIRECTION('ref_axis',(0.,-0.707106781186542,0.707106781186553));
#32021=DIRECTION('center_axis',(0.,0.,-1.));
#32022=DIRECTION('ref_axis',(0.,1.,0.));
#32023=DIRECTION('center_axis',(1.,0.,0.));
#32024=DIRECTION('ref_axis',(0.,0.707106781186543,0.707106781186552));
#37678=CARTESIAN_POINT('',(0.,0.,0.));
#37679=CARTESIAN_POINT('Origin',(-25.75,8.95,134.));
#37680=CARTESIAN_POINT('',(-25.8,8.9,135.));
#37681=CARTESIAN_POINT('',(-25.7,9.,134.9));
#37682=CARTESIAN_POINT('',(-19.150000000001,15.549999999999,128.349999999999));
#37683=CARTESIAN_POINT('',(-25.7,9.,134.15));
#37684=CARTESIAN_POINT('',(-25.7,9.,134.));
#37685=CARTESIAN_POINT('',(-25.75,8.95,134.1));
#37686=CARTESIAN_POINT('',(-19.3333333333335,15.3666666666665,140.516666666667));
#37687=CARTESIAN_POINT('',(-25.8,8.9,134.15));
#37688=CARTESIAN_POINT('',(-26.4666666666666,8.23333333333335,134.816666666667));
#37689=CARTESIAN_POINT('',(-25.8,8.9,134.));
#37690=CARTESIAN_POINT('Origin',(12.9,8.925,134.075));
#37691=CARTESIAN_POINT('',(25.7,9.,134.15));
#37692=CARTESIAN_POINT('',(12.9,9.,134.15));
#37693=CARTESIAN_POINT('',(25.75,8.95,134.1));
#37694=CARTESIAN_POINT('',(23.6333333333334,11.0666666666666,136.216666666667));
#37695=CARTESIAN_POINT('',(25.65,8.85,134.));
#37696=CARTESIAN_POINT('',(25.65,8.85,134.));
#37697=CARTESIAN_POINT('',(-25.65,8.85,134.));
#37698=CARTESIAN_POINT('',(12.9,8.85,134.));
#37699=CARTESIAN_POINT('',(-25.8,9.,134.15));
#37700=CARTESIAN_POINT('Origin',(25.8,9.,134.));
#37701=CARTESIAN_POINT('',(25.7,9.,134.9));
#37702=CARTESIAN_POINT('',(12.9,9.,134.9));
#37703=CARTESIAN_POINT('',(25.7,9.,134.));
#37704=CARTESIAN_POINT('Origin',(12.9,8.95,134.95));
#37705=CARTESIAN_POINT('',(25.8,8.9,135.));
#37706=CARTESIAN_POINT('',(12.9,8.9,135.));
#37707=CARTESIAN_POINT('',(23.4500000000003,11.2499999999997,132.65));
#37708=CARTESIAN_POINT('Origin',(25.75,8.95,134.));
#37709=CARTESIAN_POINT('',(25.8,8.9,134.15));
#37710=CARTESIAN_POINT('',(25.8,8.9,134.));
#37711=CARTESIAN_POINT('',(27.9666666666666,6.7333333333334,136.316666666667));
#37712=CARTESIAN_POINT('Origin',(25.725,-4.5,134.075));
#37713=CARTESIAN_POINT('',(25.8,-8.9,134.15));
#37714=CARTESIAN_POINT('',(25.8,-4.5,134.15));
#37715=CARTESIAN_POINT('',(25.75,-8.95,134.1));
#37716=CARTESIAN_POINT('',(26.4666666666666,-8.23333333333335,134.816666666667));
#37717=CARTESIAN_POINT('',(25.65,-8.85,134.));
#37718=CARTESIAN_POINT('',(25.65,-8.85,134.));
#37719=CARTESIAN_POINT('',(25.65,-4.5,134.));
#37720=CARTESIAN_POINT('Origin',(25.8,-9.,134.));
#37721=CARTESIAN_POINT('',(25.8,8.2,135.));
#37722=CARTESIAN_POINT('',(25.8,-9.,135.));
#37723=CARTESIAN_POINT('',(25.8,4.8,135.));
#37724=CARTESIAN_POINT('',(25.8,-2.5,135.));
#37725=CARTESIAN_POINT('',(25.8,-4.8,135.));
#37726=CARTESIAN_POINT('',(25.8,-9.,135.));
#37727=CARTESIAN_POINT('',(25.8,-8.2,135.));
#37728=CARTESIAN_POINT('',(25.8,-9.,135.));
#37729=CARTESIAN_POINT('',(25.8,-8.9,135.));
#37730=CARTESIAN_POINT('',(25.8,-9.,135.));
#37731=CARTESIAN_POINT('',(25.8,-8.9,134.));
#37732=CARTESIAN_POINT('Origin',(-25.75,-8.95,134.));
#37733=CARTESIAN_POINT('',(-25.7,-9.,134.9));
#37734=CARTESIAN_POINT('',(-25.8,-8.9,135.));
#37735=CARTESIAN_POINT('',(-23.4500000000003,-11.2499999999997,132.65));
#37736=CARTESIAN_POINT('',(-25.8,-8.9,134.15));
#37737=CARTESIAN_POINT('',(-25.8,-8.9,134.));
#37738=CARTESIAN_POINT('',(-25.75,-8.95,134.1));
#37739=CARTESIAN_POINT('',(-27.9666666666666,-6.7333333333334,136.316666666667));
#37740=CARTESIAN_POINT('',(-25.7,-9.,134.15));
#37741=CARTESIAN_POINT('',(-23.6333333333334,-11.0666666666666,136.216666666667));
#37742=CARTESIAN_POINT('',(-25.7,-9.,134.));
#37743=CARTESIAN_POINT('Origin',(-25.8,-9.,134.));
#37744=CARTESIAN_POINT('',(25.7,-9.,134.15));
#37745=CARTESIAN_POINT('',(-12.9,-9.,134.15));
#37746=CARTESIAN_POINT('',(25.7,-9.,134.9));
#37747=CARTESIAN_POINT('',(25.7,-9.,134.));
#37748=CARTESIAN_POINT('',(-12.9,-9.,134.9));
#37749=CARTESIAN_POINT('Origin',(-12.9,-8.925,134.075));
#37750=CARTESIAN_POINT('',(-25.65,-8.85,134.));
#37751=CARTESIAN_POINT('',(-25.65,-8.85,134.));
#37752=CARTESIAN_POINT('',(-12.9,-8.85,134.));
#37753=CARTESIAN_POINT('',(19.3333333333335,-15.3666666666665,140.516666666667));
#37754=CARTESIAN_POINT('Origin',(-25.725,4.5,134.075));
#37755=CARTESIAN_POINT('',(-25.65,4.5,134.));
#37756=CARTESIAN_POINT('',(-25.8,4.5,134.15));
#37757=CARTESIAN_POINT('Origin',(-12.9,-8.95,134.95));
#37758=CARTESIAN_POINT('',(19.150000000001,-15.549999999999,128.349999999999));
#37759=CARTESIAN_POINT('',(-12.9,-8.9,135.));
#37760=CARTESIAN_POINT('Origin',(0.,0.,135.));
#37761=CARTESIAN_POINT('',(-25.8,-8.2,135.));
#37762=CARTESIAN_POINT('',(-38.,-8.2,135.));
#37763=CARTESIAN_POINT('',(-25.8,9.,135.));
#37764=CARTESIAN_POINT('Origin',(25.75,-8.95,134.));
#37765=CARTESIAN_POINT('Origin',(30.,-4.55,142.5));
#37766=CARTESIAN_POINT('',(29.025,-4.6,142.5));
#37767=CARTESIAN_POINT('Origin',(30.,-4.6,142.5));
#37768=CARTESIAN_POINT('',(29.125,-4.5,142.5));
#37769=CARTESIAN_POINT('',(29.075,-4.55,142.5));
#37770=CARTESIAN_POINT('Origin',(30.,-4.5,142.5));
#37771=CARTESIAN_POINT('Origin',(-38.,-4.6,144.4));
#37772=CARTESIAN_POINT('',(-37.9,-4.6,136.));
#37773=CARTESIAN_POINT('',(-37.9,-4.6,144.));
#37774=CARTESIAN_POINT('',(-37.9,-4.6,142.2));
#37775=CARTESIAN_POINT('',(37.9,-4.6,136.));
#37776=CARTESIAN_POINT('',(-38.,-4.6,136.));
#37777=CARTESIAN_POINT('',(37.9,-4.6,144.));
#37778=CARTESIAN_POINT('',(37.9,-4.6,142.2));
#37779=CARTESIAN_POINT('',(-38.,-4.6,144.));
#37780=CARTESIAN_POINT('',(-30.975,-4.6,137.5));
#37781=CARTESIAN_POINT('Origin',(-30.,-4.6,137.5));
#37782=CARTESIAN_POINT('',(29.025,-4.6,137.5));
#37783=CARTESIAN_POINT('Origin',(30.,-4.6,137.5));
#37784=CARTESIAN_POINT('',(-30.975,-4.6,142.5));
#37785=CARTESIAN_POINT('Origin',(-30.,-4.6,142.5));
#37786=CARTESIAN_POINT('Origin',(30.,0.,142.5));
#37787=CARTESIAN_POINT('',(29.125,-4.1,142.5));
#37788=CARTESIAN_POINT('',(29.125,0.,142.5));
#37789=CARTESIAN_POINT('Origin',(30.,-4.1,142.5));
#37790=CARTESIAN_POINT('Origin',(-30.,-4.55,137.5));
#37791=CARTESIAN_POINT('',(-30.875,-4.5,137.5));
#37792=CARTESIAN_POINT('',(-30.925,-4.55,137.5));
#37793=CARTESIAN_POINT('Origin',(-30.,-4.5,137.5));
#37794=CARTESIAN_POINT('Origin',(-30.,0.,137.5));
#37795=CARTESIAN_POINT('',(-30.875,-4.1,137.5));
#37796=CARTESIAN_POINT('',(-30.875,0.,137.5));
#37797=CARTESIAN_POINT('Origin',(-30.,-4.1,137.5));
#37798=CARTESIAN_POINT('Origin',(-30.,-4.55,142.5));
#37799=CARTESIAN_POINT('',(-30.875,-4.5,142.5));
#37800=CARTESIAN_POINT('',(-30.925,-4.55,142.5));
#37801=CARTESIAN_POINT('Origin',(-30.,-4.5,142.5));
#37802=CARTESIAN_POINT('Origin',(-30.,0.,142.5));
#37803=CARTESIAN_POINT('',(-30.875,-4.1,142.5));
#37804=CARTESIAN_POINT('',(-30.875,0.,142.5));
#37805=CARTESIAN_POINT('Origin',(-30.,-4.1,142.5));
#37806=CARTESIAN_POINT('Origin',(30.,-4.55,137.5));
#37807=CARTESIAN_POINT('',(29.125,-4.5,137.5));
#37808=CARTESIAN_POINT('',(29.075,-4.55,137.5));
#37809=CARTESIAN_POINT('Origin',(30.,-4.5,137.5));
#37810=CARTESIAN_POINT('Origin',(30.,0.,137.5));
#37811=CARTESIAN_POINT('',(29.125,-4.1,137.5));
#37812=CARTESIAN_POINT('',(29.125,0.,137.5));
#37813=CARTESIAN_POINT('Origin',(30.,-4.1,137.5));
#37814=CARTESIAN_POINT('Origin',(30.,-4.05,137.5));
#37815=CARTESIAN_POINT('',(29.025,-4.,137.5));
#37816=CARTESIAN_POINT('Origin',(30.,-4.,137.5));
#37817=CARTESIAN_POINT('',(29.075,-4.05,137.5));
#37818=CARTESIAN_POINT('Origin',(-38.,-4.,135.));
#37819=CARTESIAN_POINT('',(37.9,-4.,135.8));
#37820=CARTESIAN_POINT('',(37.9,-4.,144.2));
#37821=CARTESIAN_POINT('',(37.9,-4.,137.5));
#37822=CARTESIAN_POINT('',(-37.9,-4.,135.8));
#37823=CARTESIAN_POINT('',(-38.,-4.,135.8));
#37824=CARTESIAN_POINT('',(-37.9,-4.,144.2));
#37825=CARTESIAN_POINT('',(-37.9,-4.,137.5));
#37826=CARTESIAN_POINT('',(-38.,-4.,144.2));
#37827=CARTESIAN_POINT('',(-30.975,-4.,142.5));
#37828=CARTESIAN_POINT('Origin',(-30.,-4.,142.5));
#37829=CARTESIAN_POINT('',(29.025,-4.,142.5));
#37830=CARTESIAN_POINT('Origin',(30.,-4.,142.5));
#37831=CARTESIAN_POINT('',(-30.975,-4.,137.5));
#37832=CARTESIAN_POINT('Origin',(-30.,-4.,137.5));
#37833=CARTESIAN_POINT('Origin',(-30.,-4.05,142.5));
#37834=CARTESIAN_POINT('',(-30.925,-4.05,142.5));
#37835=CARTESIAN_POINT('Origin',(-30.,-4.05,137.5));
#37836=CARTESIAN_POINT('',(-30.925,-4.05,137.5));
#37837=CARTESIAN_POINT('Origin',(30.,-4.05,142.5));
#37838=CARTESIAN_POINT('',(29.075,-4.05,142.5));
#37839=CARTESIAN_POINT('Origin',(30.,4.55,142.5));
#37840=CARTESIAN_POINT('',(29.025,4.6,142.5));
#37841=CARTESIAN_POINT('Origin',(30.,4.6,142.5));
#37842=CARTESIAN_POINT('',(29.125,4.5,142.5));
#37843=CARTESIAN_POINT('',(29.075,4.55,142.5));
#37844=CARTESIAN_POINT('Origin',(30.,4.5,142.5));
#37845=CARTESIAN_POINT('Origin',(-38.,4.6,135.6));
#37846=CARTESIAN_POINT('',(37.9,4.6,136.));
#37847=CARTESIAN_POINT('',(37.9,4.6,144.));
#37848=CARTESIAN_POINT('',(37.9,4.6,137.8));
#37849=CARTESIAN_POINT('',(-37.9,4.6,136.));
#37850=CARTESIAN_POINT('',(-38.,4.6,136.));
#37851=CARTESIAN_POINT('',(-37.9,4.6,144.));
#37852=CARTESIAN_POINT('',(-37.9,4.6,137.8));
#37853=CARTESIAN_POINT('',(-38.,4.6,144.));
#37854=CARTESIAN_POINT('',(-30.975,4.6,137.5));
#37855=CARTESIAN_POINT('Origin',(-30.,4.6,137.5));
#37856=CARTESIAN_POINT('',(29.025,4.6,137.5));
#37857=CARTESIAN_POINT('Origin',(30.,4.6,137.5));
#37858=CARTESIAN_POINT('',(-30.975,4.6,142.5));
#37859=CARTESIAN_POINT('Origin',(-30.,4.6,142.5));
#37860=CARTESIAN_POINT('Origin',(30.,0.,142.5));
#37861=CARTESIAN_POINT('',(29.125,4.1,142.5));
#37862=CARTESIAN_POINT('Origin',(30.,4.1,142.5));
#37863=CARTESIAN_POINT('',(29.125,0.,142.5));
#37864=CARTESIAN_POINT('Origin',(-30.,4.55,137.5));
#37865=CARTESIAN_POINT('',(-30.875,4.5,137.5));
#37866=CARTESIAN_POINT('',(-30.925,4.55,137.5));
#37867=CARTESIAN_POINT('Origin',(-30.,4.5,137.5));
#37868=CARTESIAN_POINT('Origin',(-30.,0.,137.5));
#37869=CARTESIAN_POINT('',(-30.875,4.1,137.5));
#37870=CARTESIAN_POINT('Origin',(-30.,4.1,137.5));
#37871=CARTESIAN_POINT('',(-30.875,0.,137.5));
#37872=CARTESIAN_POINT('Origin',(-30.,4.55,142.5));
#37873=CARTESIAN_POINT('',(-30.875,4.5,142.5));
#37874=CARTESIAN_POINT('',(-30.925,4.55,142.5));
#37875=CARTESIAN_POINT('Origin',(-30.,4.5,142.5));
#37876=CARTESIAN_POINT('Origin',(-30.,0.,142.5));
#37877=CARTESIAN_POINT('',(-30.875,4.1,142.5));
#37878=CARTESIAN_POINT('Origin',(-30.,4.1,142.5));
#37879=CARTESIAN_POINT('',(-30.875,0.,142.5));
#37880=CARTESIAN_POINT('Origin',(30.,4.55,137.5));
#37881=CARTESIAN_POINT('',(29.125,4.5,137.5));
#37882=CARTESIAN_POINT('',(29.075,4.55,137.5));
#37883=CARTESIAN_POINT('Origin',(30.,4.5,137.5));
#37884=CARTESIAN_POINT('Origin',(30.,0.,137.5));
#37885=CARTESIAN_POINT('',(29.125,4.1,137.5));
#37886=CARTESIAN_POINT('Origin',(30.,4.1,137.5));
#37887=CARTESIAN_POINT('',(29.125,0.,137.5));
#37888=CARTESIAN_POINT('Origin',(30.,-8.95,142.5));
#37889=CARTESIAN_POINT('',(30.8485281374239,-9.,144.2));
#37890=CARTESIAN_POINT('',(30.80386876177,-8.9,144.110526315789));
#37891=CARTESIAN_POINT('',(30.8485281374239,-9.,144.2));
#37892=CARTESIAN_POINT('',(28.2,-8.9,142.5));
#37893=CARTESIAN_POINT('Origin',(30.,-8.9,142.5));
#37894=CARTESIAN_POINT('',(29.19613123823,-8.9,144.110526315789));
#37895=CARTESIAN_POINT('Origin',(30.,-8.9,142.5));
#37896=CARTESIAN_POINT('',(29.1514718625761,-9.,144.2));
#37897=CARTESIAN_POINT('',(29.19613123823,-8.9,144.110526315789));
#37898=CARTESIAN_POINT('Origin',(30.,-9.,142.5));
#37899=CARTESIAN_POINT('Ctrl Pts',(29.37557606376,-8.99442305443429,144.29429745799));
#37900=CARTESIAN_POINT('Ctrl Pts',(29.4528789423666,-8.99125209441901,144.321011685441));
#37901=CARTESIAN_POINT('Ctrl Pts',(29.6108779014912,-8.98340236313526,144.364462672992));
#37902=CARTESIAN_POINT('Ctrl Pts',(29.8538300241761,-8.97543935789693,144.397225194892));
#37903=CARTESIAN_POINT('Ctrl Pts',(30.1578937093748,-8.97381382255402,144.402534138038));
#37904=CARTESIAN_POINT('Ctrl Pts',(30.4034174830284,-8.98452879794544,144.36323637123));
#37905=CARTESIAN_POINT('Ctrl Pts',(30.5816912715748,-8.99263170993257,144.308616992978));
#37906=CARTESIAN_POINT('Ctrl Pts',(30.6031336007836,-8.99354972599348,144.301654944207));
#37907=CARTESIAN_POINT('Ctrl Pts',(30.62442393624,-8.99442305443429,144.29429745799));
#37908=CARTESIAN_POINT('Ctrl Pts',(29.3865147164033,-8.96294870295619,144.262864971993));
#37909=CARTESIAN_POINT('Ctrl Pts',(29.4621247530599,-8.96082929478778,144.289053145881));
#37910=CARTESIAN_POINT('Ctrl Pts',(29.6170733795065,-8.95481417908684,144.331935721362));
#37911=CARTESIAN_POINT('Ctrl Pts',(29.8560577408031,-8.94828380943131,144.364473342857));
#37912=CARTESIAN_POINT('Ctrl Pts',(30.1554889558999,-8.9469018651377,144.369780678576));
#37913=CARTESIAN_POINT('Ctrl Pts',(30.3970550842887,-8.95587368877562,144.3306496463));
#37914=CARTESIAN_POINT('Ctrl Pts',(30.5716687838969,-8.96172308279366,144.276909344891));
#37915=CARTESIAN_POINT('Ctrl Pts',(30.5926595579726,-8.9623708163431,144.270081805573));
#37916=CARTESIAN_POINT('Ctrl Pts',(30.6134852835967,-8.96294870295619,144.262864971993));
#37917=CARTESIAN_POINT('Ctrl Pts',(29.3974533690466,-8.9314743514781,144.231432485996));
#37918=CARTESIAN_POINT('Ctrl Pts',(29.4713946846489,-8.93042279963123,144.257101347462));
#37919=CARTESIAN_POINT('Ctrl Pts',(29.6232594585157,-8.92620755420488,144.299394395606));
#37920=CARTESIAN_POINT('Ctrl Pts',(29.8582882281875,-8.92111994873181,144.331713130336));
#37921=CARTESIAN_POINT('Ctrl Pts',(30.1530997401632,-8.91998748202325,144.337018634271));
#37922=CARTESIAN_POINT('Ctrl Pts',(30.3906863776209,-8.92714570081842,144.297997431227));
#37923=CARTESIAN_POINT('Ctrl Pts',(30.5616480648658,-8.93082793618361,144.245213046289));
#37924=CARTESIAN_POINT('Ctrl Pts',(30.5821837421954,-8.93117890965038,144.238497833085));
#37925=CARTESIAN_POINT('Ctrl Pts',(30.6025466309533,-8.9314743514781,144.231432485997));
#37926=CARTESIAN_POINT('Ctrl Pts',(29.40839202169,-8.9,144.2));
#37927=CARTESIAN_POINT('Ctrl Pts',(29.4806404953422,-8.9,144.225142807902));
#37928=CARTESIAN_POINT('Ctrl Pts',(29.6294549365309,-8.89761937015647,144.266867443976));
#37929=CARTESIAN_POINT('Ctrl Pts',(29.8605159448146,-8.89396440026619,144.298961278301));
#37930=CARTESIAN_POINT('Ctrl Pts',(30.1506949866883,-8.89307552460693,144.304265174808));
#37931=CARTESIAN_POINT('Ctrl Pts',(30.3843239788812,-8.8984905916486,144.265410706296));
#37932=CARTESIAN_POINT('Ctrl Pts',(30.5516255771879,-8.8999193090447,144.213505398201));
#37933=CARTESIAN_POINT('Ctrl Pts',(30.5717096993844,-8.9,144.206924694451));
#37934=CARTESIAN_POINT('Ctrl Pts',(30.59160797831,-8.9,144.2));
#37935=CARTESIAN_POINT('',(30.59160797831,-8.9,144.2));
#37936=CARTESIAN_POINT('',(30.62442393624,-8.99442305443429,144.29429745799));
#37937=CARTESIAN_POINT('',(30.59160797831,-8.9,144.2));
#37938=CARTESIAN_POINT('',(29.37557606376,-8.99442305443429,144.29429745799));
#37939=CARTESIAN_POINT('Ctrl Pts',(30.62442393624,-8.99442305443429,144.29429745799));
#37940=CARTESIAN_POINT('Ctrl Pts',(30.6031336007836,-8.99354972599348,144.301654944207));
#37941=CARTESIAN_POINT('Ctrl Pts',(30.5816912715748,-8.99263170993257,144.308616992978));
#37942=CARTESIAN_POINT('Ctrl Pts',(30.4034174830284,-8.98452879794544,144.36323637123));
#37943=CARTESIAN_POINT('Ctrl Pts',(30.1578937093748,-8.97381382255402,144.402534138038));
#37944=CARTESIAN_POINT('Ctrl Pts',(29.8538300241761,-8.97543935789693,144.397225194892));
#37945=CARTESIAN_POINT('Ctrl Pts',(29.6108779014912,-8.98340236313526,144.364462672992));
#37946=CARTESIAN_POINT('Ctrl Pts',(29.4528789423666,-8.99125209441901,144.321011685441));
#37947=CARTESIAN_POINT('Ctrl Pts',(29.37557606376,-8.99442305443429,144.29429745799));
#37948=CARTESIAN_POINT('',(29.40839202169,-8.9,144.2));
#37949=CARTESIAN_POINT('',(29.37557606376,-8.99442305443429,144.29429745799));
#37950=CARTESIAN_POINT('Ctrl Pts',(29.40839202169,-8.9,144.2));
#37951=CARTESIAN_POINT('Ctrl Pts',(29.4806404953422,-8.9,144.225142807902));
#37952=CARTESIAN_POINT('Ctrl Pts',(29.6294549365309,-8.89761937015647,144.266867443976));
#37953=CARTESIAN_POINT('Ctrl Pts',(29.8605159448146,-8.89396440026619,144.298961278301));
#37954=CARTESIAN_POINT('Ctrl Pts',(30.1506949866883,-8.89307552460693,144.304265174808));
#37955=CARTESIAN_POINT('Ctrl Pts',(30.3843239788812,-8.8984905916486,144.265410706296));
#37956=CARTESIAN_POINT('Ctrl Pts',(30.5516255771879,-8.8999193090447,144.213505398201));
#37957=CARTESIAN_POINT('Ctrl Pts',(30.5717096993844,-8.9,144.206924694451));
#37958=CARTESIAN_POINT('Ctrl Pts',(30.59160797831,-8.9,144.2));
#37959=CARTESIAN_POINT('Ctrl Pts',(29.1514718625761,-9.,144.2));
#37960=CARTESIAN_POINT('Ctrl Pts',(29.2240383852933,-9.,144.236220433153));
#37961=CARTESIAN_POINT('Ctrl Pts',(29.2989266202372,-8.99756721057679,144.267809043778));
#37962=CARTESIAN_POINT('Ctrl Pts',(29.37557606376,-8.99442305443429,144.29429745799));
#37963=CARTESIAN_POINT('Ctrl Pts',(29.1663583211274,-8.96666666666667,144.170175438596));
#37964=CARTESIAN_POINT('Ctrl Pts',(29.2376517469549,-8.96666666666667,144.205760425554));
#37965=CARTESIAN_POINT('Ctrl Pts',(29.3112262464824,-8.96504480705119,144.236788199029));
#37966=CARTESIAN_POINT('Ctrl Pts',(29.3865147164034,-8.96294870295619,144.262864971993));
#37967=CARTESIAN_POINT('Ctrl Pts',(29.1812447796787,-8.93333333333333,144.140350877193));
#37968=CARTESIAN_POINT('Ctrl Pts',(29.2512651086164,-8.93333333333333,144.175300417955));
#37969=CARTESIAN_POINT('Ctrl Pts',(29.3235258727276,-8.9325224035256,144.20576735428));
#37970=CARTESIAN_POINT('Ctrl Pts',(29.3974533690467,-8.9314743514781,144.231432485997));
#37971=CARTESIAN_POINT('Ctrl Pts',(29.19613123823,-8.9,144.110526315789));
#37972=CARTESIAN_POINT('Ctrl Pts',(29.2648784702779,-8.9,144.144840410356));
#37973=CARTESIAN_POINT('Ctrl Pts',(29.3358254989728,-8.9,144.174746509531));
#37974=CARTESIAN_POINT('Ctrl Pts',(29.40839202169,-8.9,144.2));
#37975=CARTESIAN_POINT('Ctrl Pts',(29.37557606376,-8.99442305443429,144.29429745799));
#37976=CARTESIAN_POINT('Ctrl Pts',(29.2989266202372,-8.99756721057679,144.267809043778));
#37977=CARTESIAN_POINT('Ctrl Pts',(29.2240383852933,-9.,144.236220433153));
#37978=CARTESIAN_POINT('Ctrl Pts',(29.1514718625761,-9.,144.2));
#37979=CARTESIAN_POINT('Ctrl Pts',(29.19613123823,-8.9,144.110526315789));
#37980=CARTESIAN_POINT('Ctrl Pts',(29.2648784702779,-8.9,144.144840410356));
#37981=CARTESIAN_POINT('Ctrl Pts',(29.3358254989728,-8.9,144.174746509531));
#37982=CARTESIAN_POINT('Ctrl Pts',(29.40839202169,-8.9,144.2));
#37983=CARTESIAN_POINT('Ctrl Pts',(30.62442393624,-8.99442305443429,144.29429745799));
#37984=CARTESIAN_POINT('Ctrl Pts',(30.7010733797633,-8.99756721057681,144.267809043778));
#37985=CARTESIAN_POINT('Ctrl Pts',(30.7759616147076,-9.00000000000003,144.236220433153));
#37986=CARTESIAN_POINT('Ctrl Pts',(30.8485281374252,-9.,144.199999999999));
#37987=CARTESIAN_POINT('Ctrl Pts',(30.6134852835966,-8.96294870295619,144.262864971993));
#37988=CARTESIAN_POINT('Ctrl Pts',(30.688773753518,-8.96504480705121,144.236788199029));
#37989=CARTESIAN_POINT('Ctrl Pts',(30.762348253046,-8.96666666666669,144.205760425554));
#37990=CARTESIAN_POINT('Ctrl Pts',(30.8336416788739,-8.96666666666667,144.170175438596));
#37991=CARTESIAN_POINT('Ctrl Pts',(30.6025466309533,-8.9314743514781,144.231432485997));
#37992=CARTESIAN_POINT('Ctrl Pts',(30.6764741272728,-8.9325224035256,144.20576735428));
#37993=CARTESIAN_POINT('Ctrl Pts',(30.7487348913845,-8.93333333333334,144.175300417955));
#37994=CARTESIAN_POINT('Ctrl Pts',(30.8187552203225,-8.93333333333333,144.140350877192));
#37995=CARTESIAN_POINT('Ctrl Pts',(30.59160797831,-8.9,144.2));
#37996=CARTESIAN_POINT('Ctrl Pts',(30.6641745010276,-8.9,144.174746509531));
#37997=CARTESIAN_POINT('Ctrl Pts',(30.7351215297229,-8.9,144.144840410355));
#37998=CARTESIAN_POINT('Ctrl Pts',(30.8038687617712,-8.9,144.110526315789));
#37999=CARTESIAN_POINT('Ctrl Pts',(30.8485281374252,-9.,144.199999999999));
#38000=CARTESIAN_POINT('Ctrl Pts',(30.7759616147076,-9.00000000000003,144.236220433153));
#38001=CARTESIAN_POINT('Ctrl Pts',(30.7010733797633,-8.99756721057681,144.267809043778));
#38002=CARTESIAN_POINT('Ctrl Pts',(30.62442393624,-8.99442305443429,144.29429745799));
#38003=CARTESIAN_POINT('Ctrl Pts',(30.59160797831,-8.9,144.2));
#38004=CARTESIAN_POINT('Ctrl Pts',(30.6641745010276,-8.9,144.174746509531));
#38005=CARTESIAN_POINT('Ctrl Pts',(30.7351215297229,-8.9,144.144840410355));
#38006=CARTESIAN_POINT('Ctrl Pts',(30.8038687617712,-8.9,144.110526315789));
#38007=CARTESIAN_POINT('Origin',(-38.,-8.2,144.2));
#38008=CARTESIAN_POINT('',(37.9,-9.,144.2));
#38009=CARTESIAN_POINT('',(-38.,-9.,144.2));
#38010=CARTESIAN_POINT('',(37.9,-8.2,145.));
#38011=CARTESIAN_POINT('Origin',(37.9,-8.2,144.2));
#38012=CARTESIAN_POINT('',(-37.9,-8.2,145.));
#38013=CARTESIAN_POINT('',(-38.,-8.2,145.));
#38014=CARTESIAN_POINT('',(-37.9,-9.,144.2));
#38015=CARTESIAN_POINT('Origin',(-37.9,-8.2,144.2));
#38016=CARTESIAN_POINT('',(-30.8485281374239,-9.,144.2));
#38017=CARTESIAN_POINT('',(-38.,-9.,144.2));
#38018=CARTESIAN_POINT('',(-30.62442393624,-8.99442305443429,144.29429745799));
#38019=CARTESIAN_POINT('Ctrl Pts',(-30.62442393624,-8.99442305443429,144.29429745799));
#38020=CARTESIAN_POINT('Ctrl Pts',(-30.7010733797628,-8.99756721057679,
144.267809043778));
#38021=CARTESIAN_POINT('Ctrl Pts',(-30.7759616147067,-9.,144.236220433153));
#38022=CARTESIAN_POINT('Ctrl Pts',(-30.8485281374239,-9.,144.2));
#38023=CARTESIAN_POINT('',(-29.37557606376,-8.99442305443429,144.29429745799));
#38024=CARTESIAN_POINT('Ctrl Pts',(-29.37557606376,-8.99442305443429,144.29429745799));
#38025=CARTESIAN_POINT('Ctrl Pts',(-29.3968663992163,-8.99354972599348,
144.301654944207));
#38026=CARTESIAN_POINT('Ctrl Pts',(-29.4183151210873,-8.99261764548661,
144.308633020031));
#38027=CARTESIAN_POINT('Ctrl Pts',(-29.5181405190621,-8.98818372075475,
144.339120021515));
#38028=CARTESIAN_POINT('Ctrl Pts',(-29.6784757526138,-8.98055560583611,
144.37677095198));
#38029=CARTESIAN_POINT('Ctrl Pts',(-29.917310908637,-8.97429943254969,144.401048817597));
#38030=CARTESIAN_POINT('Ctrl Pts',(-30.1466727558104,-8.97528496697549,
144.397455998416));
#38031=CARTESIAN_POINT('Ctrl Pts',(-30.3890975283267,-8.98340931878656,
144.364446023987));
#38032=CARTESIAN_POINT('Ctrl Pts',(-30.5471210576335,-8.99125209441902,
144.321011685441));
#38033=CARTESIAN_POINT('Ctrl Pts',(-30.62442393624,-8.99442305443429,144.29429745799));
#38034=CARTESIAN_POINT('',(-29.1514718625761,-9.,144.2));
#38035=CARTESIAN_POINT('Ctrl Pts',(-29.1514718625749,-9.,144.199999999999));
#38036=CARTESIAN_POINT('Ctrl Pts',(-29.2240383852925,-9.00000000000003,
144.236220433153));
#38037=CARTESIAN_POINT('Ctrl Pts',(-29.2989266202368,-8.99756721057681,
144.267809043778));
#38038=CARTESIAN_POINT('Ctrl Pts',(-29.37557606376,-8.99442305443429,144.29429745799));
#38039=CARTESIAN_POINT('',(-38.,-9.,144.2));
#38040=CARTESIAN_POINT('Origin',(30.,-9.1,142.5));
#38041=CARTESIAN_POINT('',(28.2,-8.5,142.5));
#38042=CARTESIAN_POINT('',(28.2,-9.1,142.5));
#38043=CARTESIAN_POINT('',(28.8951880620293,-8.5,143.921052631579));
#38044=CARTESIAN_POINT('Origin',(30.,-8.5,142.5));
#38045=CARTESIAN_POINT('',(29.0050125628934,-8.5,144.));
#38046=CARTESIAN_POINT('Ctrl Pts',(29.0050125628934,-8.5,144.));
#38047=CARTESIAN_POINT('Ctrl Pts',(28.9674326867105,-8.5,143.975072330207));
#38048=CARTESIAN_POINT('Ctrl Pts',(28.9307900499921,-8.5,143.948731762135));
#38049=CARTESIAN_POINT('Ctrl Pts',(28.8951880620293,-8.5,143.921052631579));
#38050=CARTESIAN_POINT('',(30.9949874371066,-8.5,144.));
#38051=CARTESIAN_POINT('Ctrl Pts',(30.9949874371066,-8.5,144.));
#38052=CARTESIAN_POINT('Ctrl Pts',(30.9864258065899,-8.5,144.005679143204));
#38053=CARTESIAN_POINT('Ctrl Pts',(30.9778381533882,-8.49988803935537,144.011270671384));
#38054=CARTESIAN_POINT('Ctrl Pts',(30.9692257738747,-8.49967189801602,144.016774735463));
#38055=CARTESIAN_POINT('Ctrl Pts',(30.957514713753,-8.49937799036647,144.024259127581));
#38056=CARTESIAN_POINT('Ctrl Pts',(30.9457617930679,-8.49889895697764,144.031575977005));
#38057=CARTESIAN_POINT('Ctrl Pts',(30.9339633564761,-8.49823699277985,144.038742874564));
#38058=CARTESIAN_POINT('Ctrl Pts',(30.7924312547142,-8.4902961793105,144.124715797054));
#38059=CARTESIAN_POINT('Ctrl Pts',(30.6455798173351,-8.45921759112122,144.187305181965));
#38060=CARTESIAN_POINT('Ctrl Pts',(30.4983882415935,-8.42943950721129,144.229760076013));
#38061=CARTESIAN_POINT('Ctrl Pts',(30.351196665852,-8.39966142330136,144.272214970061));
#38062=CARTESIAN_POINT('Ctrl Pts',(30.203664951748,-8.37118384367076,144.294535373247));
#38063=CARTESIAN_POINT('Ctrl Pts',(30.0579688188435,-8.36568430314537,144.299260363718));
#38064=CARTESIAN_POINT('Ctrl Pts',(30.0552225698401,-8.36558064145315,144.299349425796));
#38065=CARTESIAN_POINT('Ctrl Pts',(30.0524708101528,-8.36548152859756,144.29943128211));
#38066=CARTESIAN_POINT('Ctrl Pts',(30.0497199697297,-8.36539021135648,144.299506886864));
#38067=CARTESIAN_POINT('Ctrl Pts',(30.0414674484601,-8.36511625963326,144.299733701128));
#38068=CARTESIAN_POINT('Ctrl Pts',(30.033223200568,-8.36491246844071,144.299904251363));
#38069=CARTESIAN_POINT('Ctrl Pts',(30.0249742066664,-8.36477495772506,144.300018317497));
#38070=CARTESIAN_POINT('Ctrl Pts',(30.0019993209539,-8.36439196641558,144.300336011563));
#38071=CARTESIAN_POINT('Ctrl Pts',(29.9790119784398,-8.36454534261746,144.300212596464));
#38072=CARTESIAN_POINT('Ctrl Pts',(29.9560473210098,-8.36522412779964,144.299650865472));
#38073=CARTESIAN_POINT('Ctrl Pts',(29.9330826635799,-8.36590291298182,144.29908913448));
#38074=CARTESIAN_POINT('Ctrl Pts',(29.910140691234,-8.36710710714431,144.298089087593));
#38075=CARTESIAN_POINT('Ctrl Pts',(29.8871242708781,-8.36880464134516,144.296640642262));
#38076=CARTESIAN_POINT('Ctrl Pts',(29.8702147027416,-8.37005177577307,144.295576506978));
#38077=CARTESIAN_POINT('Ctrl Pts',(29.8533332047851,-8.37156072057906,144.294283011609));
#38078=CARTESIAN_POINT('Ctrl Pts',(29.8364165493979,-8.37330886307701,144.292734900211));
#38079=CARTESIAN_POINT('Ctrl Pts',(29.8194998940106,-8.37505700557497,144.291186788813));
#38080=CARTESIAN_POINT('Ctrl Pts',(29.8025480811926,-8.3770443457649,144.289384061385));
#38081=CARTESIAN_POINT('Ctrl Pts',(29.7856564998322,-8.37924514274765,144.287392801698));
#38082=CARTESIAN_POINT('Ctrl Pts',(29.5878470697021,-8.40501764963735,144.264074088329));
#38083=CARTESIAN_POINT('Ctrl Pts',(29.3817564945146,-8.46015770243706,144.20400082464));
#38084=CARTESIAN_POINT('Ctrl Pts',(29.1909226085664,-8.4860152481162,144.108025770902));
#38085=CARTESIAN_POINT('Ctrl Pts',(29.1273113132504,-8.49463443000924,144.076034086322));
#38086=CARTESIAN_POINT('Ctrl Pts',(29.0653952056276,-8.5,144.04005331396));
#38087=CARTESIAN_POINT('Ctrl Pts',(29.0050125628934,-8.5,144.));
#38088=CARTESIAN_POINT('',(31.1048119379707,-8.5,143.921052631579));
#38089=CARTESIAN_POINT('Ctrl Pts',(31.1048119379707,-8.5,143.921052631579));
#38090=CARTESIAN_POINT('Ctrl Pts',(31.0692099500079,-8.5,143.948731762135));
#38091=CARTESIAN_POINT('Ctrl Pts',(31.0325673132895,-8.5,143.975072330207));
#38092=CARTESIAN_POINT('Ctrl Pts',(30.9949874371066,-8.5,144.));
#38093=CARTESIAN_POINT('Origin',(30.,-8.5,142.5));
#38094=CARTESIAN_POINT('Origin',(30.,4.05,137.5));
#38095=CARTESIAN_POINT('',(29.025,4.,137.5));
#38096=CARTESIAN_POINT('Origin',(30.,4.,137.5));
#38097=CARTESIAN_POINT('',(29.075,4.05,137.5));
#38098=CARTESIAN_POINT('Origin',(-38.,4.,145.));
#38099=CARTESIAN_POINT('',(-37.9,4.,135.8));
#38100=CARTESIAN_POINT('',(-37.9,4.,144.2));
#38101=CARTESIAN_POINT('',(-37.9,4.,142.5));
#38102=CARTESIAN_POINT('',(37.9,4.,135.8));
#38103=CARTESIAN_POINT('',(-38.,4.,135.8));
#38104=CARTESIAN_POINT('',(37.9,4.,144.2));
#38105=CARTESIAN_POINT('',(37.9,4.,142.5));
#38106=CARTESIAN_POINT('',(-38.,4.,144.2));
#38107=CARTESIAN_POINT('',(-30.975,4.,142.5));
#38108=CARTESIAN_POINT('Origin',(-30.,4.,142.5));
#38109=CARTESIAN_POINT('',(29.025,4.,142.5));
#38110=CARTESIAN_POINT('Origin',(30.,4.,142.5));
#38111=CARTESIAN_POINT('',(-30.975,4.,137.5));
#38112=CARTESIAN_POINT('Origin',(-30.,4.,137.5));
#38113=CARTESIAN_POINT('Origin',(-30.,4.05,142.5));
#38114=CARTESIAN_POINT('',(-30.925,4.05,142.5));
#38115=CARTESIAN_POINT('Origin',(-30.,4.05,137.5));
#38116=CARTESIAN_POINT('',(-30.925,4.05,137.5));
#38117=CARTESIAN_POINT('Origin',(30.,4.05,142.5));
#38118=CARTESIAN_POINT('',(29.075,4.05,142.5));
#38119=CARTESIAN_POINT('Origin',(37.95,-8.2,135.8));
#38120=CARTESIAN_POINT('',(38.,-8.90000000000001,135.8));
#38121=CARTESIAN_POINT('',(37.9,-9.,135.8));
#38122=CARTESIAN_POINT('',(38.,-8.90000000000001,135.8));
#38123=CARTESIAN_POINT('',(37.9,-8.2,135.));
#38124=CARTESIAN_POINT('Origin',(37.9,-8.2,135.8));
#38125=CARTESIAN_POINT('',(38.,-8.2,135.1));
#38126=CARTESIAN_POINT('',(37.9,-8.2,135.));
#38127=CARTESIAN_POINT('Origin',(38.,-8.2,135.8));
#38128=CARTESIAN_POINT('Origin',(37.95,-8.95,142.5));
#38129=CARTESIAN_POINT('',(38.,-8.9,144.2));
#38130=CARTESIAN_POINT('',(38.,-8.9,142.5));
#38131=CARTESIAN_POINT('',(38.,-8.9,144.2));
#38132=CARTESIAN_POINT('',(37.9,-9.,142.5));
#38133=CARTESIAN_POINT('Origin',(37.95,-8.2,144.2));
#38134=CARTESIAN_POINT('',(38.,-8.2,144.9));
#38135=CARTESIAN_POINT('',(38.,-8.2,144.9));
#38136=CARTESIAN_POINT('Origin',(38.,-8.2,144.2));
#38137=CARTESIAN_POINT('Origin',(37.95,-5.25,144.95));
#38138=CARTESIAN_POINT('',(38.,-4.8,144.9));
#38139=CARTESIAN_POINT('',(38.,-5.25,144.9));
#38140=CARTESIAN_POINT('',(37.9,-4.8,145.));
#38141=CARTESIAN_POINT('',(38.,-4.8,144.9));
#38142=CARTESIAN_POINT('',(37.9,-5.25,145.));
#38143=CARTESIAN_POINT('Origin',(37.95,-4.8,144.2));
#38144=CARTESIAN_POINT('',(38.,-4.09999999999999,144.2));
#38145=CARTESIAN_POINT('',(38.,-4.09999999999999,144.2));
#38146=CARTESIAN_POINT('Origin',(37.9,-4.8,144.2));
#38147=CARTESIAN_POINT('Origin',(38.,-4.8,144.2));
#38148=CARTESIAN_POINT('Origin',(37.95,-4.05,137.5));
#38149=CARTESIAN_POINT('',(38.,-4.1,135.8));
#38150=CARTESIAN_POINT('',(38.,-4.1,137.5));
#38151=CARTESIAN_POINT('',(38.,-4.1,135.8));
#38152=CARTESIAN_POINT('Origin',(37.95,-4.8,135.8));
#38153=CARTESIAN_POINT('',(38.,-4.8,135.1));
#38154=CARTESIAN_POINT('',(37.9,-4.8,135.));
#38155=CARTESIAN_POINT('',(38.,-4.8,135.1));
#38156=CARTESIAN_POINT('Origin',(37.9,-4.8,135.8));
#38157=CARTESIAN_POINT('Origin',(38.,-4.8,135.8));
#38158=CARTESIAN_POINT('Origin',(37.95,-7.75,135.05));
#38159=CARTESIAN_POINT('',(38.,-7.75,135.1));
#38160=CARTESIAN_POINT('',(37.9,-7.75,135.));
#38161=CARTESIAN_POINT('Origin',(-38.,-4.8,135.8));
#38162=CARTESIAN_POINT('',(-38.,-4.8,135.));
#38163=CARTESIAN_POINT('',(-25.8,-4.8,135.));
#38164=CARTESIAN_POINT('',(-38.,-4.8,135.));
#38165=CARTESIAN_POINT('',(-37.9,-4.8,135.));
#38166=CARTESIAN_POINT('',(-38.,-4.8,135.));
#38167=CARTESIAN_POINT('Origin',(-37.9,-4.8,135.8));
#38168=CARTESIAN_POINT('Origin',(-38.,-9.,135.));
#38169=CARTESIAN_POINT('',(-38.,-8.2,135.));
#38170=CARTESIAN_POINT('Origin',(-38.,-8.2,135.8));
#38171=CARTESIAN_POINT('',(30.8485281374239,-9.,135.8));
#38172=CARTESIAN_POINT('',(-38.,-9.,135.8));
#38173=CARTESIAN_POINT('',(30.62442393624,-8.99442305443429,135.70570254201));
#38174=CARTESIAN_POINT('Ctrl Pts',(30.62442393624,-8.99442305443429,135.70570254201));
#38175=CARTESIAN_POINT('Ctrl Pts',(30.7010733797628,-8.99756721057679,135.732190956222));
#38176=CARTESIAN_POINT('Ctrl Pts',(30.7759616147067,-9.,135.763779566847));
#38177=CARTESIAN_POINT('Ctrl Pts',(30.8485281374239,-9.,135.8));
#38178=CARTESIAN_POINT('',(29.37557606376,-8.99442305443429,135.70570254201));
#38179=CARTESIAN_POINT('Ctrl Pts',(29.37557606376,-8.99442305443429,135.70570254201));
#38180=CARTESIAN_POINT('Ctrl Pts',(29.3968663992163,-8.99354972599348,135.698345055793));
#38181=CARTESIAN_POINT('Ctrl Pts',(29.418327451187,-8.9926309002887,135.69138245992));
#38182=CARTESIAN_POINT('Ctrl Pts',(29.5876626138109,-8.9849459908676,135.639432675438));
#38183=CARTESIAN_POINT('Ctrl Pts',(29.8198774693528,-8.97481364719588,135.600649477793));
#38184=CARTESIAN_POINT('Ctrl Pts',(30.1802232821902,-8.97487183787893,135.600774173325));
#38185=CARTESIAN_POINT('Ctrl Pts',(30.4123094665995,-8.98495128128084,135.639444028187));
#38186=CARTESIAN_POINT('Ctrl Pts',(30.5816752394099,-8.9926310079646,135.691382689721));
#38187=CARTESIAN_POINT('Ctrl Pts',(30.6031336007837,-8.99354972599348,135.698345055793));
#38188=CARTESIAN_POINT('Ctrl Pts',(30.62442393624,-8.99442305443429,135.70570254201));
#38189=CARTESIAN_POINT('',(29.1514718625761,-9.,135.8));
#38190=CARTESIAN_POINT('Ctrl Pts',(29.1514718625748,-9.,135.800000000001));
#38191=CARTESIAN_POINT('Ctrl Pts',(29.2240383852925,-9.00000000000003,135.763779566847));
#38192=CARTESIAN_POINT('Ctrl Pts',(29.2989266202368,-8.99756721057681,135.732190956222));
#38193=CARTESIAN_POINT('Ctrl Pts',(29.37557606376,-8.99442305443429,135.70570254201));
#38194=CARTESIAN_POINT('',(-29.1514718625761,-9.,135.8));
#38195=CARTESIAN_POINT('',(-38.,-9.,135.8));
#38196=CARTESIAN_POINT('',(-29.37557606376,-8.99442305443429,135.70570254201));
#38197=CARTESIAN_POINT('Ctrl Pts',(-29.37557606376,-8.99442305443429,135.70570254201));
#38198=CARTESIAN_POINT('Ctrl Pts',(-29.2989266202372,-8.99756721057679,
135.732190956222));
#38199=CARTESIAN_POINT('Ctrl Pts',(-29.2240383852933,-9.,135.763779566847));
#38200=CARTESIAN_POINT('Ctrl Pts',(-29.1514718625761,-9.,135.8));
#38201=CARTESIAN_POINT('',(-30.62442393624,-8.99442305443429,135.70570254201));
#38202=CARTESIAN_POINT('Ctrl Pts',(-30.62442393624,-8.99442305443429,135.70570254201));
#38203=CARTESIAN_POINT('Ctrl Pts',(-30.6031336007836,-8.99354972599348,
135.698345055793));
#38204=CARTESIAN_POINT('Ctrl Pts',(-30.5816983343991,-8.992618351102,135.691367354698));
#38205=CARTESIAN_POINT('Ctrl Pts',(-30.4860771888921,-8.98837705676011,
135.662197780903));
#38206=CARTESIAN_POINT('Ctrl Pts',(-30.3737545882272,-8.98306085361229,
135.635119083645));
#38207=CARTESIAN_POINT('Ctrl Pts',(-30.1448588692225,-8.97549018477832,
135.602654705543));
#38208=CARTESIAN_POINT('Ctrl Pts',(-29.8570705077091,-8.9729461125948,135.594307424048));
#38209=CARTESIAN_POINT('Ctrl Pts',(-29.5879619148511,-8.98495065878909,
135.639399710956));
#38210=CARTESIAN_POINT('Ctrl Pts',(-29.4183017766692,-8.99262938782785,
135.691384779087));
#38211=CARTESIAN_POINT('Ctrl Pts',(-29.3968663992164,-8.99354972599348,
135.698345055793));
#38212=CARTESIAN_POINT('Ctrl Pts',(-29.37557606376,-8.99442305443429,135.70570254201));
#38213=CARTESIAN_POINT('',(-30.8485281374239,-9.,135.8));
#38214=CARTESIAN_POINT('Ctrl Pts',(-30.8485281374251,-9.,135.800000000001));
#38215=CARTESIAN_POINT('Ctrl Pts',(-30.7759616147075,-9.00000000000003,
135.763779566847));
#38216=CARTESIAN_POINT('Ctrl Pts',(-30.7010733797632,-8.99756721057681,
135.732190956222));
#38217=CARTESIAN_POINT('Ctrl Pts',(-30.62442393624,-8.99442305443429,135.70570254201));
#38218=CARTESIAN_POINT('',(-37.9,-9.,135.8));
#38219=CARTESIAN_POINT('',(-38.,-9.,135.8));
#38220=CARTESIAN_POINT('',(-37.9,-8.2,135.));
#38221=CARTESIAN_POINT('Origin',(-37.9,-8.2,135.8));
#38222=CARTESIAN_POINT('',(-38.,-8.2,135.));
#38223=CARTESIAN_POINT('Origin',(38.,-6.5,140.));
#38224=CARTESIAN_POINT('',(38.,-8.5,144.));
#38225=CARTESIAN_POINT('',(38.,-8.5,136.));
#38226=CARTESIAN_POINT('',(38.,-8.5,137.8));
#38227=CARTESIAN_POINT('',(38.,-8.,144.5));
#38228=CARTESIAN_POINT('Origin',(38.,-8.,144.));
#38229=CARTESIAN_POINT('',(38.,-5.,144.5));
#38230=CARTESIAN_POINT('',(38.,-7.45,144.5));
#38231=CARTESIAN_POINT('',(38.,-4.50000000000002,144.));
#38232=CARTESIAN_POINT('Origin',(38.,-5.,144.));
#38233=CARTESIAN_POINT('',(38.,-4.5,136.));
#38234=CARTESIAN_POINT('',(38.,-4.5,142.2));
#38235=CARTESIAN_POINT('',(38.,-5.,135.5));
#38236=CARTESIAN_POINT('Origin',(38.,-5.,136.));
#38237=CARTESIAN_POINT('',(38.,-8.,135.5));
#38238=CARTESIAN_POINT('',(38.,-5.55,135.5));
#38239=CARTESIAN_POINT('Origin',(38.,-8.,136.));
#38240=CARTESIAN_POINT('Origin',(-37.95,-8.2,135.8));
#38241=CARTESIAN_POINT('',(-38.,-8.2,135.1));
#38242=CARTESIAN_POINT('',(-38.,-8.2,135.1));
#38243=CARTESIAN_POINT('',(-38.,-8.90000000000001,135.8));
#38244=CARTESIAN_POINT('',(-37.9,-9.,135.8));
#38245=CARTESIAN_POINT('Origin',(-38.,-8.2,135.8));
#38246=CARTESIAN_POINT('Origin',(-37.95,-7.75,135.05));
#38247=CARTESIAN_POINT('',(-38.,-4.8,135.1));
#38248=CARTESIAN_POINT('',(-38.,-7.75,135.1));
#38249=CARTESIAN_POINT('',(-38.,-4.8,135.1));
#38250=CARTESIAN_POINT('',(-37.9,-7.75,135.));
#38251=CARTESIAN_POINT('Origin',(-37.95,-4.8,135.8));
#38252=CARTESIAN_POINT('',(-38.,-4.09999999999999,135.8));
#38253=CARTESIAN_POINT('',(-38.,-4.09999999999999,135.8));
#38254=CARTESIAN_POINT('Origin',(-38.,-4.8,135.8));
#38255=CARTESIAN_POINT('Origin',(-37.95,-4.05,137.5));
#38256=CARTESIAN_POINT('',(-38.,-4.1,144.2));
#38257=CARTESIAN_POINT('',(-38.,-4.1,137.5));
#38258=CARTESIAN_POINT('',(-38.,-4.1,144.2));
#38259=CARTESIAN_POINT('Origin',(-37.95,-4.8,144.2));
#38260=CARTESIAN_POINT('',(-38.,-4.8,144.9));
#38261=CARTESIAN_POINT('',(-37.9,-4.8,145.));
#38262=CARTESIAN_POINT('',(-38.,-4.8,144.9));
#38263=CARTESIAN_POINT('Origin',(-37.9,-4.8,144.2));
#38264=CARTESIAN_POINT('Origin',(-38.,-4.8,144.2));
#38265=CARTESIAN_POINT('Origin',(-37.95,-5.25,144.95));
#38266=CARTESIAN_POINT('',(-38.,-8.2,144.9));
#38267=CARTESIAN_POINT('',(-38.,-5.25,144.9));
#38268=CARTESIAN_POINT('',(-38.,-8.2,144.9));
#38269=CARTESIAN_POINT('',(-37.9,-5.25,145.));
#38270=CARTESIAN_POINT('Origin',(-37.95,-8.2,144.2));
#38271=CARTESIAN_POINT('',(-38.,-8.90000000000001,144.2));
#38272=CARTESIAN_POINT('',(-38.,-8.90000000000001,144.2));
#38273=CARTESIAN_POINT('Origin',(-38.,-8.2,144.2));
#38274=CARTESIAN_POINT('Origin',(-37.95,-8.95,142.5));
#38275=CARTESIAN_POINT('',(-38.,-8.9,142.5));
#38276=CARTESIAN_POINT('',(-37.9,-9.,142.5));
#38277=CARTESIAN_POINT('Origin',(-38.,-4.,145.));
#38278=CARTESIAN_POINT('',(-38.,-4.8,145.));
#38279=CARTESIAN_POINT('Origin',(-38.,-9.,145.));
#38280=CARTESIAN_POINT('Origin',(-30.,-9.,142.5));
#38281=CARTESIAN_POINT('Origin',(-30.,-9.,137.5));
#38282=CARTESIAN_POINT('Origin',(30.,-9.,137.5));
#38283=CARTESIAN_POINT('',(3.47230558097363,-9.,138.054707050323));
#38284=CARTESIAN_POINT('',(2.71739415824413,-9.,138.770942211151));
#38285=CARTESIAN_POINT('Ctrl Pts',(3.47230558097363,-9.,138.054707050323));
#38286=CARTESIAN_POINT('Ctrl Pts',(3.00675420463085,-9.,138.281037330627));
#38287=CARTESIAN_POINT('Ctrl Pts',(2.71739415824413,-9.,138.770942211151));
#38288=CARTESIAN_POINT('',(2.42803601920605,-9.,139.997135639191));
#38289=CARTESIAN_POINT('Ctrl Pts',(2.71739415824413,-9.,138.770942211151));
#38290=CARTESIAN_POINT('Ctrl Pts',(2.42803601920605,-9.,139.260846614838));
#38291=CARTESIAN_POINT('Ctrl Pts',(2.42803601920605,-9.,139.997135639191));
#38292=CARTESIAN_POINT('',(3.00102452933788,-9.,141.598636388779));
#38293=CARTESIAN_POINT('Ctrl Pts',(2.42803601920605,-9.,139.997135639191));
#38294=CARTESIAN_POINT('Ctrl Pts',(2.42803601920605,-9.,141.025648593903));
#38295=CARTESIAN_POINT('Ctrl Pts',(3.00102452933788,-9.,141.598636388779));
#38296=CARTESIAN_POINT('',(4.59679441154003,-9.,142.171624183655));
#38297=CARTESIAN_POINT('Ctrl Pts',(3.00102452933788,-9.,141.598636388779));
#38298=CARTESIAN_POINT('Ctrl Pts',(3.57401113212109,-9.,142.171624183655));
#38299=CARTESIAN_POINT('Ctrl Pts',(4.59679441154003,-9.,142.171624183655));
#38300=CARTESIAN_POINT('',(6.2126200646162,-9.,141.60866355896));
#38301=CARTESIAN_POINT('Ctrl Pts',(4.59679441154003,-9.,142.171624183655));
#38302=CARTESIAN_POINT('Ctrl Pts',(5.64536122977734,-9.,142.171624183655));
#38303=CARTESIAN_POINT('Ctrl Pts',(6.2126200646162,-9.,141.60866355896));
#38304=CARTESIAN_POINT('',(6.77987699210644,-9.,140.031514644623));
#38305=CARTESIAN_POINT('Ctrl Pts',(6.2126200646162,-9.,141.60866355896));
#38306=CARTESIAN_POINT('Ctrl Pts',(6.77987699210644,-9.,141.045703411102));
#38307=CARTESIAN_POINT('Ctrl Pts',(6.77987699210644,-9.,140.031514644623));
#38308=CARTESIAN_POINT('',(6.53206090629101,-9.,138.823943138123));
#38309=CARTESIAN_POINT('Ctrl Pts',(6.77987699210644,-9.,140.031514644623));
#38310=CARTESIAN_POINT('Ctrl Pts',(6.77987699210644,-9.,139.29522562027));
#38311=CARTESIAN_POINT('Ctrl Pts',(6.53206090629101,-9.,138.823943138123));
#38312=CARTESIAN_POINT('',(5.81582669913769,-9.,138.090518951416));
#38313=CARTESIAN_POINT('Ctrl Pts',(6.53206090629101,-9.,138.823943138123));
#38314=CARTESIAN_POINT('Ctrl Pts',(6.28424291312695,-9.,138.352660655975));
#38315=CARTESIAN_POINT('Ctrl Pts',(5.81582669913769,-9.,138.090518951416));
#38316=CARTESIAN_POINT('',(4.64836339652538,-9.,137.828377246857));
#38317=CARTESIAN_POINT('Ctrl Pts',(5.81582669913769,-9.,138.090518951416));
#38318=CARTESIAN_POINT('Ctrl Pts',(5.3474085777998,-9.,137.828377246857));
#38319=CARTESIAN_POINT('Ctrl Pts',(4.64836339652538,-9.,137.828377246857));
#38320=CARTESIAN_POINT('Ctrl Pts',(4.64836339652538,-9.,137.828377246857));
#38321=CARTESIAN_POINT('Ctrl Pts',(3.93785886466503,-9.,137.828377246857));
#38322=CARTESIAN_POINT('Ctrl Pts',(3.47230558097363,-9.,138.054707050323));
#38323=CARTESIAN_POINT('',(-0.41684789955616,-9.,141.062892436981));
#38324=CARTESIAN_POINT('',(-1.74044962227345,-9.,141.062892436981));
#38325=CARTESIAN_POINT('',(-19.2084239497781,-9.,141.062892436981));
#38326=CARTESIAN_POINT('',(-1.74044962227345,-9.,142.10000038147));
#38327=CARTESIAN_POINT('',(-1.74044962227345,-9.,143.031446218491));
#38328=CARTESIAN_POINT('',(2.20457105338573,-9.,142.10000038147));
#38329=CARTESIAN_POINT('',(-19.8702248111367,-9.,142.10000038147));
#38330=CARTESIAN_POINT('',(2.20457105338573,-9.,141.062892436981));
#38331=CARTESIAN_POINT('',(2.20457105338573,-9.,143.550000190735));
#38332=CARTESIAN_POINT('',(0.880968376994133,-9.,141.062892436981));
#38333=CARTESIAN_POINT('',(-17.8977144733071,-9.,141.062892436981));
#38334=CARTESIAN_POINT('',(0.880968376994133,-9.,137.900000572205));
#38335=CARTESIAN_POINT('',(0.880968376994133,-9.,143.031446218491));
#38336=CARTESIAN_POINT('',(-0.41684789955616,-9.,137.900000572205));
#38337=CARTESIAN_POINT('',(-18.5595158115029,-9.,137.900000572205));
#38338=CARTESIAN_POINT('',(-0.41684789955616,-9.,141.450000286102));
#38339=CARTESIAN_POINT('',(-7.1838323622942,-9.,138.493042945862));
#38340=CARTESIAN_POINT('',(-7.42019005119801,-9.,139.127626895905));
#38341=CARTESIAN_POINT('Ctrl Pts',(-7.1838323622942,-9.,138.493042945862));
#38342=CARTESIAN_POINT('Ctrl Pts',(-7.33567447960377,-9.,138.725102901459));
#38343=CARTESIAN_POINT('Ctrl Pts',(-7.42019005119801,-9.,139.127626895905));
#38344=CARTESIAN_POINT('',(-7.50470562279224,-9.,140.01719045639));
#38345=CARTESIAN_POINT('Ctrl Pts',(-7.42019005119801,-9.,139.127626895905));
#38346=CARTESIAN_POINT('Ctrl Pts',(-7.50470562279224,-9.,139.53015089035));
#38347=CARTESIAN_POINT('Ctrl Pts',(-7.50470562279224,-9.,140.01719045639));
#38348=CARTESIAN_POINT('',(-7.07353182137012,-9.,141.693179368973));
#38349=CARTESIAN_POINT('Ctrl Pts',(-7.50470562279224,-9.,140.01719045639));
#38350=CARTESIAN_POINT('Ctrl Pts',(-7.50470562279224,-9.,141.214734554291));
#38351=CARTESIAN_POINT('Ctrl Pts',(-7.07353182137012,-9.,141.693179368973));
#38352=CARTESIAN_POINT('',(-5.75995798408985,-9.,142.171624183655));
#38353=CARTESIAN_POINT('Ctrl Pts',(-7.07353182137012,-9.,141.693179368973));
#38354=CARTESIAN_POINT('Ctrl Pts',(-6.64235849678516,-9.,142.171624183655));
#38355=CARTESIAN_POINT('Ctrl Pts',(-5.75995798408985,-9.,142.171624183655));
#38356=CARTESIAN_POINT('',(-5.06377764046192,-9.,142.067054271698));
#38357=CARTESIAN_POINT('Ctrl Pts',(-5.75995798408985,-9.,142.171624183655));
#38358=CARTESIAN_POINT('Ctrl Pts',(-5.3359467536211,-9.,142.171624183655));
#38359=CARTESIAN_POINT('Ctrl Pts',(-5.06377764046192,-9.,142.067054271698));
#38360=CARTESIAN_POINT('',(-4.61971254646778,-9.,141.794884681702));
#38361=CARTESIAN_POINT('Ctrl Pts',(-5.06377764046192,-9.,142.067054271698));
#38362=CARTESIAN_POINT('Ctrl Pts',(-4.79160852730274,-9.,141.962483882904));
#38363=CARTESIAN_POINT('Ctrl Pts',(-4.61971254646778,-9.,141.794884681702));
#38364=CARTESIAN_POINT('',(-4.34897585213184,-9.,141.442497253418));
#38365=CARTESIAN_POINT('Ctrl Pts',(-4.61971254646778,-9.,141.794884681702));
#38366=CARTESIAN_POINT('Ctrl Pts',(-4.44781656563282,-9.,141.627285718918));
#38367=CARTESIAN_POINT('Ctrl Pts',(-4.34897585213184,-9.,141.442497253418));
#38368=CARTESIAN_POINT('',(-4.18997164070606,-9.,141.011323928833));
#38369=CARTESIAN_POINT('Ctrl Pts',(-4.34897585213184,-9.,141.442497253418));
#38370=CARTESIAN_POINT('Ctrl Pts',(-4.25013513863087,-9.,141.2577085495));
#38371=CARTESIAN_POINT('Ctrl Pts',(-4.18997164070606,-9.,141.011323928833));
#38372=CARTESIAN_POINT('',(-4.07250948250294,-9.,140.031514644623));
#38373=CARTESIAN_POINT('Ctrl Pts',(-4.18997164070606,-9.,141.011323928833));
#38374=CARTESIAN_POINT('Ctrl Pts',(-4.07250948250294,-9.,140.541473865509));
#38375=CARTESIAN_POINT('Ctrl Pts',(-4.07250948250294,-9.,140.031514644623));
#38376=CARTESIAN_POINT('',(-4.45927591621876,-9.,138.358390808105));
#38377=CARTESIAN_POINT('Ctrl Pts',(-4.07250948250294,-9.,140.031514644623));
#38378=CARTESIAN_POINT('Ctrl Pts',(-4.07250948250294,-9.,138.888404369354));
#38379=CARTESIAN_POINT('Ctrl Pts',(-4.45927591621876,-9.,138.358390808105));
#38380=CARTESIAN_POINT('',(-5.7914721518755,-9.,137.828377246857));
#38381=CARTESIAN_POINT('Ctrl Pts',(-4.45927591621876,-9.,138.358390808105));
#38382=CARTESIAN_POINT('Ctrl Pts',(-4.84604234993458,-9.,137.828377246857));
#38383=CARTESIAN_POINT('Ctrl Pts',(-5.7914721518755,-9.,137.828377246857));
#38384=CARTESIAN_POINT('',(-6.64808912575245,-9.,137.997408390045));
#38385=CARTESIAN_POINT('Ctrl Pts',(-5.7914721518755,-9.,137.828377246857));
#38386=CARTESIAN_POINT('Ctrl Pts',(-6.32148618996143,-9.,137.828377246857));
#38387=CARTESIAN_POINT('Ctrl Pts',(-6.64808912575245,-9.,137.997408390045));
#38388=CARTESIAN_POINT('Ctrl Pts',(-6.64808912575245,-9.,137.997408390045));
#38389=CARTESIAN_POINT('Ctrl Pts',(-6.97469206154346,-9.,138.166440010071));
#38390=CARTESIAN_POINT('Ctrl Pts',(-7.1838323622942,-9.,138.493042945862));
#38391=CARTESIAN_POINT('',(-9.82530565559864,-9.,138.851160049438));
#38392=CARTESIAN_POINT('',(-8.00320501625538,-9.,138.851160049438));
#38393=CARTESIAN_POINT('',(-23.9126528277993,-9.,138.851160049438));
#38394=CARTESIAN_POINT('',(-8.00320501625538,-9.,137.900000572205));
#38395=CARTESIAN_POINT('',(-8.00320501625538,-9.,141.925580024719));
#38396=CARTESIAN_POINT('',(-11.5041598826647,-9.,137.900000572205));
#38397=CARTESIAN_POINT('',(-23.0016025081277,-9.,137.900000572205));
#38398=CARTESIAN_POINT('',(-11.1388804465532,-9.,138.875512123108));
#38399=CARTESIAN_POINT('Ctrl Pts',(-11.5041598826647,-9.,137.900000572205));
#38400=CARTESIAN_POINT('Ctrl Pts',(-11.4439961463213,-9.,138.41855430603));
#38401=CARTESIAN_POINT('Ctrl Pts',(-11.1388804465532,-9.,138.875512123108));
#38402=CARTESIAN_POINT('',(-9.99433727562428,-9.,139.954161167145));
#38403=CARTESIAN_POINT('Ctrl Pts',(-11.1388804465532,-9.,138.875512123108));
#38404=CARTESIAN_POINT('Ctrl Pts',(-10.833764269948,-9.,139.332469940186));
#38405=CARTESIAN_POINT('Ctrl Pts',(-9.99433727562428,-9.,139.954161167145));
#38406=CARTESIAN_POINT('',(-9.3382660895586,-9.,140.53287935257));
#38407=CARTESIAN_POINT('Ctrl Pts',(-9.99433727562428,-9.,139.954161167145));
#38408=CARTESIAN_POINT('Ctrl Pts',(-9.48151321709156,-9.,140.335197925568));
#38409=CARTESIAN_POINT('Ctrl Pts',(-9.3382660895586,-9.,140.53287935257));
#38410=CARTESIAN_POINT('',(-9.1950194388628,-9.,140.908185958862));
#38411=CARTESIAN_POINT('Ctrl Pts',(-9.3382660895586,-9.,140.53287935257));
#38412=CARTESIAN_POINT('Ctrl Pts',(-9.1950194388628,-9.,140.730559825897));
#38413=CARTESIAN_POINT('Ctrl Pts',(-9.1950194388628,-9.,140.908185958862));
#38414=CARTESIAN_POINT('',(-9.33683367073536,-9.,141.236221313477));
#38415=CARTESIAN_POINT('Ctrl Pts',(-9.1950194388628,-9.,140.908185958862));
#38416=CARTESIAN_POINT('Ctrl Pts',(-9.1950194388628,-9.,141.100136756897));
#38417=CARTESIAN_POINT('Ctrl Pts',(-9.33683367073536,-9.,141.236221313477));
#38418=CARTESIAN_POINT('',(-9.69351883232594,-9.,141.372305870056));
#38419=CARTESIAN_POINT('Ctrl Pts',(-9.33683367073536,-9.,141.236221313477));
#38420=CARTESIAN_POINT('Ctrl Pts',(-9.47864837944508,-9.,141.372305870056));
#38421=CARTESIAN_POINT('Ctrl Pts',(-9.69351883232594,-9.,141.372305870056));
#38422=CARTESIAN_POINT('',(-10.058798506856,-9.,141.231924057007));
#38423=CARTESIAN_POINT('Ctrl Pts',(-9.69351883232594,-9.,141.372305870056));
#38424=CARTESIAN_POINT('Ctrl Pts',(-9.91698379814625,-9.,141.372305870056));
#38425=CARTESIAN_POINT('Ctrl Pts',(-10.058798506856,-9.,141.231924057007));
#38426=CARTESIAN_POINT('',(-10.2493168860674,-9.,140.73628950119));
#38427=CARTESIAN_POINT('Ctrl Pts',(-10.058798506856,-9.,141.231924057007));
#38428=CARTESIAN_POINT('Ctrl Pts',(-10.2006127387285,-9.,141.09154176712));
#38429=CARTESIAN_POINT('Ctrl Pts',(-10.2493168860674,-9.,140.73628950119));
#38430=CARTESIAN_POINT('',(-11.4182116538286,-9.,140.830832958221));
#38431=CARTESIAN_POINT('',(-24.20578526978,-9.,141.865127447373));
#38432=CARTESIAN_POINT('',(-11.1660971194506,-9.,141.600068569183));
#38433=CARTESIAN_POINT('Ctrl Pts',(-11.4182116538286,-9.,140.830832958221));
#38434=CARTESIAN_POINT('Ctrl Pts',(-11.3494531661272,-9.,141.323601961136));
#38435=CARTESIAN_POINT('Ctrl Pts',(-11.1660971194506,-9.,141.600068569183));
#38436=CARTESIAN_POINT('',(-10.6489760428667,-9.,142.024079322815));
#38437=CARTESIAN_POINT('Ctrl Pts',(-11.1660971194506,-9.,141.600068569183));
#38438=CARTESIAN_POINT('Ctrl Pts',(-10.9827410727739,-9.,141.876535177231));
#38439=CARTESIAN_POINT('Ctrl Pts',(-10.6489760428667,-9.,142.024079322815));
#38440=CARTESIAN_POINT('',(-9.72503300011158,-9.,142.171623706818));
#38441=CARTESIAN_POINT('Ctrl Pts',(-10.6489760428667,-9.,142.024079322815));
#38442=CARTESIAN_POINT('Ctrl Pts',(-10.3152105361223,-9.,142.171623706818));
#38443=CARTESIAN_POINT('Ctrl Pts',(-9.72503300011158,-9.,142.171623706818));
#38444=CARTESIAN_POINT('',(-8.76671095192432,-9.,142.031241893768));
#38445=CARTESIAN_POINT('Ctrl Pts',(-9.72503300011158,-9.,142.171623706818));
#38446=CARTESIAN_POINT('Ctrl Pts',(-9.10907144844532,-9.,142.171623706818));
#38447=CARTESIAN_POINT('Ctrl Pts',(-8.76671095192432,-9.,142.031241893768));
#38448=CARTESIAN_POINT('',(-8.22810240089893,-9.,141.600068569183));
#38449=CARTESIAN_POINT('Ctrl Pts',(-8.76671095192432,-9.,142.031241893768));
#38450=CARTESIAN_POINT('Ctrl Pts',(-8.42435093224049,-9.,141.8908598423));
#38451=CARTESIAN_POINT('Ctrl Pts',(-8.22810240089893,-9.,141.600068569183));
#38452=CARTESIAN_POINT('',(-8.03185434639454,-9.,140.948295116425));
#38453=CARTESIAN_POINT('Ctrl Pts',(-8.22810240089893,-9.,141.600068569183));
#38454=CARTESIAN_POINT('Ctrl Pts',(-8.03185434639454,-9.,141.309277296066));
#38455=CARTESIAN_POINT('Ctrl Pts',(-8.03185434639454,-9.,140.948295116425));
#38456=CARTESIAN_POINT('',(-8.25675220787525,-9.,140.214870929718));
#38457=CARTESIAN_POINT('Ctrl Pts',(-8.03185434639454,-9.,140.948295116425));
#38458=CARTESIAN_POINT('Ctrl Pts',(-8.03185434639454,-9.,140.564393520355));
#38459=CARTESIAN_POINT('Ctrl Pts',(-8.25675220787525,-9.,140.214870929718));
#38460=CARTESIAN_POINT('',(-9.07469196617603,-9.,139.447067260742));
#38461=CARTESIAN_POINT('Ctrl Pts',(-8.25675220787525,-9.,140.214870929718));
#38462=CARTESIAN_POINT('Ctrl Pts',(-8.48165006935596,-9.,139.865348339081));
#38463=CARTESIAN_POINT('Ctrl Pts',(-9.07469196617603,-9.,139.447067260742));
#38464=CARTESIAN_POINT('',(-9.54597444832325,-9.,139.106139659882));
#38465=CARTESIAN_POINT('Ctrl Pts',(-9.07469196617603,-9.,139.447067260742));
#38466=CARTESIAN_POINT('Ctrl Pts',(-9.42707939445972,-9.,139.203547477722));
#38467=CARTESIAN_POINT('Ctrl Pts',(-9.54597444832325,-9.,139.106139659882));
#38468=CARTESIAN_POINT('Ctrl Pts',(-9.54597444832325,-9.,139.106139659882));
#38469=CARTESIAN_POINT('Ctrl Pts',(-9.66486950218678,-9.,139.008731842041));
#38470=CARTESIAN_POINT('Ctrl Pts',(-9.82530565559864,-9.,138.851160049438));
#38471=CARTESIAN_POINT('',(8.70797948539257,-9.,137.900000572205));
#38472=CARTESIAN_POINT('',(7.4875166863203,-9.,137.900000572205));
#38473=CARTESIAN_POINT('',(-14.6460102573037,-9.,137.900000572205));
#38474=CARTESIAN_POINT('',(7.4875166863203,-9.,142.10000038147));
#38475=CARTESIAN_POINT('',(7.4875166863203,-9.,141.450000286102));
#38476=CARTESIAN_POINT('',(8.69938497245312,-9.,142.10000038147));
#38477=CARTESIAN_POINT('',(-15.2562416568398,-9.,142.10000038147));
#38478=CARTESIAN_POINT('',(10.2808306664228,-9.,139.776356220245));
#38479=CARTESIAN_POINT('',(0.633198898756767,-9.,153.951780208601));
#38480=CARTESIAN_POINT('',(10.2808306664228,-9.,142.10000038147));
#38481=CARTESIAN_POINT('',(10.2808306664228,-9.,142.388178110123));
#38482=CARTESIAN_POINT('',(11.5041602104902,-9.,142.10000038147));
#38483=CARTESIAN_POINT('',(-13.8595846667886,-9.,142.10000038147));
#38484=CARTESIAN_POINT('',(11.5041602104902,-9.,137.900000572205));
#38485=CARTESIAN_POINT('',(11.5041602104902,-9.,143.550000190735));
#38486=CARTESIAN_POINT('',(10.2808306664228,-9.,137.900000572205));
#38487=CARTESIAN_POINT('',(-13.2479198947549,-9.,137.900000572205));
#38488=CARTESIAN_POINT('',(8.70797948539257,-9.,140.206097126007));
#38489=CARTESIAN_POINT('',(0.963975333484397,-9.,151.560268138963));
#38490=CARTESIAN_POINT('',(8.70797948539257,-9.,142.603048563004));
#38491=CARTESIAN_POINT('Origin',(-38.,-6.5,140.));
#38492=CARTESIAN_POINT('',(-38.,-8.5,136.));
#38493=CARTESIAN_POINT('',(-38.,-8.5,144.));
#38494=CARTESIAN_POINT('',(-38.,-8.5,137.8));
#38495=CARTESIAN_POINT('',(-38.,-8.,135.5));
#38496=CARTESIAN_POINT('Origin',(-38.,-8.,136.));
#38497=CARTESIAN_POINT('',(-38.,-5.,135.5));
#38498=CARTESIAN_POINT('',(-38.,-5.55,135.5));
#38499=CARTESIAN_POINT('',(-38.,-4.5,136.));
#38500=CARTESIAN_POINT('Origin',(-38.,-5.,136.));
#38501=CARTESIAN_POINT('',(-38.,-4.50000000000002,144.));
#38502=CARTESIAN_POINT('',(-38.,-4.5,142.2));
#38503=CARTESIAN_POINT('',(-38.,-5.,144.5));
#38504=CARTESIAN_POINT('Origin',(-38.,-5.,144.));
#38505=CARTESIAN_POINT('',(-38.,-8.,144.5));
#38506=CARTESIAN_POINT('',(-38.,-7.45,144.5));
#38507=CARTESIAN_POINT('Origin',(-38.,-8.,144.));
#38508=CARTESIAN_POINT('Origin',(-30.,-8.95,137.5));
#38509=CARTESIAN_POINT('',(-30.80386876177,-8.9,135.889473684211));
#38510=CARTESIAN_POINT('',(-30.8485281374239,-9.,135.8));
#38511=CARTESIAN_POINT('',(-31.8,-8.9,137.5));
#38512=CARTESIAN_POINT('Origin',(-30.,-8.9,137.5));
#38513=CARTESIAN_POINT('',(-29.19613123823,-8.9,135.889473684211));
#38514=CARTESIAN_POINT('Origin',(-30.,-8.9,137.5));
#38515=CARTESIAN_POINT('',(-29.19613123823,-8.9,135.889473684211));
#38516=CARTESIAN_POINT('Ctrl Pts',(-29.37557606376,-8.99442305443429,135.70570254201));
#38517=CARTESIAN_POINT('Ctrl Pts',(-29.3968663992164,-8.99354972599348,
135.698345055793));
#38518=CARTESIAN_POINT('Ctrl Pts',(-29.4183017766692,-8.99262938782785,
135.691384779087));
#38519=CARTESIAN_POINT('Ctrl Pts',(-29.5879619148511,-8.98495065878909,
135.639399710956));
#38520=CARTESIAN_POINT('Ctrl Pts',(-29.8570705077091,-8.9729461125948,135.594307424048));
#38521=CARTESIAN_POINT('Ctrl Pts',(-30.1448588692225,-8.97549018477832,
135.602654705543));
#38522=CARTESIAN_POINT('Ctrl Pts',(-30.3737545882272,-8.98306085361229,
135.635119083645));
#38523=CARTESIAN_POINT('Ctrl Pts',(-30.4860771888921,-8.98837705676011,
135.662197780903));
#38524=CARTESIAN_POINT('Ctrl Pts',(-30.5816983343991,-8.992618351102,135.691367354698));
#38525=CARTESIAN_POINT('Ctrl Pts',(-30.6031336007836,-8.99354972599348,
135.698345055793));
#38526=CARTESIAN_POINT('Ctrl Pts',(-30.62442393624,-8.99442305443429,135.70570254201));
#38527=CARTESIAN_POINT('Ctrl Pts',(-29.3865147164033,-8.96294870295619,
135.737135028007));
#38528=CARTESIAN_POINT('Ctrl Pts',(-29.4073401763186,-8.96237080371183,
135.729919445576));
#38529=CARTESIAN_POINT('Ctrl Pts',(-29.4283245697951,-8.96172080557183,
135.72309086562));
#38530=CARTESIAN_POINT('Ctrl Pts',(-29.5945002385617,-8.95618563279747,
135.671952952223));
#38531=CARTESIAN_POINT('Ctrl Pts',(-29.8591951245291,-8.94617870256798,
135.627077056189));
#38532=CARTESIAN_POINT('Ctrl Pts',(-30.1426747355265,-8.94833727126047,
135.635411682665));
#38533=CARTESIAN_POINT('Ctrl Pts',(-30.3677622830885,-8.95449993845067,
135.66762787594));
#38534=CARTESIAN_POINT('Ctrl Pts',(-30.4780284899699,-8.95865446655877,
135.694387451391));
#38535=CARTESIAN_POINT('Ctrl Pts',(-30.5716737136164,-8.96171637205332,
135.723071391253));
#38536=CARTESIAN_POINT('Ctrl Pts',(-30.5926609072949,-8.96236576597913,
135.729921064971));
#38537=CARTESIAN_POINT('Ctrl Pts',(-30.6134852835967,-8.96294870295619,
135.737135028007));
#38538=CARTESIAN_POINT('Ctrl Pts',(-29.3974533690467,-8.9314743514781,135.768567514003));
#38539=CARTESIAN_POINT('Ctrl Pts',(-29.4178165235133,-8.93117892228165,
135.761500915766));
#38540=CARTESIAN_POINT('Ctrl Pts',(-29.4383449903957,-8.93082558621927,
135.754789398524));
#38541=CARTESIAN_POINT('Ctrl Pts',(-29.6010478369904,-8.92735259191528,
135.704550691614));
#38542=CARTESIAN_POINT('Ctrl Pts',(-29.8613411523255,-8.91940114687363,
135.659840357084));
#38543=CARTESIAN_POINT('Ctrl Pts',(-30.1404740235453,-8.92117767633548,
135.668188953759));
#38544=CARTESIAN_POINT('Ctrl Pts',(-30.3617898553802,-8.92591554353793,
135.700139778803));
#38545=CARTESIAN_POINT('Ctrl Pts',(-30.4699427578485,-8.92894382168888,
135.726593040274));
#38546=CARTESIAN_POINT('Ctrl Pts',(-30.561657334651,-8.93081126900573,135.754772293159));
#38547=CARTESIAN_POINT('Ctrl Pts',(-30.5821823928732,-8.93118396001435,
135.761499296371));
#38548=CARTESIAN_POINT('Ctrl Pts',(-30.6025466309533,-8.9314743514781,135.768567514003));
#38549=CARTESIAN_POINT('Ctrl Pts',(-29.40839202169,-8.9,135.8));
#38550=CARTESIAN_POINT('Ctrl Pts',(-29.4282903006156,-8.9,135.793075305549));
#38551=CARTESIAN_POINT('Ctrl Pts',(-29.4483677835215,-8.89991700396325,
135.786495485057));
#38552=CARTESIAN_POINT('Ctrl Pts',(-29.6075861607011,-8.89858756592366,
135.737103932881));
#38553=CARTESIAN_POINT('Ctrl Pts',(-29.8634657691454,-8.89263373684681,
135.692609989225));
#38554=CARTESIAN_POINT('Ctrl Pts',(-30.1382898898493,-8.89402476281763,
135.700945930881));
#38555=CARTESIAN_POINT('Ctrl Pts',(-30.3557975502414,-8.89735462837631,
135.732648571097));
#38556=CARTESIAN_POINT('Ctrl Pts',(-30.4618940589263,-8.89922123148754,
135.758782710762));
#38557=CARTESIAN_POINT('Ctrl Pts',(-30.5516327138684,-8.89990928995705,
135.786476329714));
#38558=CARTESIAN_POINT('Ctrl Pts',(-30.5717096993844,-8.9,135.793075305549));
#38559=CARTESIAN_POINT('Ctrl Pts',(-30.59160797831,-8.9,135.8));
#38560=CARTESIAN_POINT('',(-30.59160797831,-8.9,135.8));
#38561=CARTESIAN_POINT('',(-30.59160797831,-8.9,135.8));
#38562=CARTESIAN_POINT('',(-29.40839202169,-8.9,135.8));
#38563=CARTESIAN_POINT('',(-29.37557606376,-8.99442305443429,135.70570254201));
#38564=CARTESIAN_POINT('Ctrl Pts',(-29.40839202169,-8.9,135.8));
#38565=CARTESIAN_POINT('Ctrl Pts',(-29.4282903006156,-8.9,135.793075305549));
#38566=CARTESIAN_POINT('Ctrl Pts',(-29.4483677835215,-8.89991700396325,
135.786495485057));
#38567=CARTESIAN_POINT('Ctrl Pts',(-29.6075861607011,-8.89858756592366,
135.737103932881));
#38568=CARTESIAN_POINT('Ctrl Pts',(-29.8634657691454,-8.89263373684681,
135.692609989225));
#38569=CARTESIAN_POINT('Ctrl Pts',(-30.1382898898493,-8.89402476281763,
135.700945930881));
#38570=CARTESIAN_POINT('Ctrl Pts',(-30.3557975502414,-8.89735462837631,
135.732648571097));
#38571=CARTESIAN_POINT('Ctrl Pts',(-30.4618940589263,-8.89922123148754,
135.758782710762));
#38572=CARTESIAN_POINT('Ctrl Pts',(-30.5516327138684,-8.89990928995705,
135.786476329714));
#38573=CARTESIAN_POINT('Ctrl Pts',(-30.5717096993844,-8.9,135.793075305549));
#38574=CARTESIAN_POINT('Ctrl Pts',(-30.59160797831,-8.9,135.8));
#38575=CARTESIAN_POINT('Ctrl Pts',(-29.1514718625761,-9.,135.8));
#38576=CARTESIAN_POINT('Ctrl Pts',(-29.2240383852933,-9.,135.763779566847));
#38577=CARTESIAN_POINT('Ctrl Pts',(-29.2989266202372,-8.99756721057679,
135.732190956222));
#38578=CARTESIAN_POINT('Ctrl Pts',(-29.37557606376,-8.99442305443429,135.70570254201));
#38579=CARTESIAN_POINT('Ctrl Pts',(-29.1663583211274,-8.96666666666667,
135.829824561404));
#38580=CARTESIAN_POINT('Ctrl Pts',(-29.2376517469549,-8.96666666666667,
135.794239574446));
#38581=CARTESIAN_POINT('Ctrl Pts',(-29.3112262464824,-8.96504480705119,
135.763211800971));
#38582=CARTESIAN_POINT('Ctrl Pts',(-29.3865147164034,-8.96294870295619,
135.737135028007));
#38583=CARTESIAN_POINT('Ctrl Pts',(-29.1812447796787,-8.93333333333333,
135.859649122807));
#38584=CARTESIAN_POINT('Ctrl Pts',(-29.2512651086164,-8.93333333333333,
135.824699582045));
#38585=CARTESIAN_POINT('Ctrl Pts',(-29.3235258727276,-8.9325224035256,135.79423264572));
#38586=CARTESIAN_POINT('Ctrl Pts',(-29.3974533690467,-8.9314743514781,135.768567514003));
#38587=CARTESIAN_POINT('Ctrl Pts',(-29.19613123823,-8.9,135.889473684211));
#38588=CARTESIAN_POINT('Ctrl Pts',(-29.2648784702779,-8.9,135.855159589644));
#38589=CARTESIAN_POINT('Ctrl Pts',(-29.3358254989728,-8.9,135.825253490469));
#38590=CARTESIAN_POINT('Ctrl Pts',(-29.40839202169,-8.9,135.8));
#38591=CARTESIAN_POINT('Ctrl Pts',(-29.19613123823,-8.9,135.889473684211));
#38592=CARTESIAN_POINT('Ctrl Pts',(-29.2648784702779,-8.9,135.855159589644));
#38593=CARTESIAN_POINT('Ctrl Pts',(-29.3358254989728,-8.9,135.825253490469));
#38594=CARTESIAN_POINT('Ctrl Pts',(-29.40839202169,-8.9,135.8));
#38595=CARTESIAN_POINT('Ctrl Pts',(-30.62442393624,-8.99442305443429,135.70570254201));
#38596=CARTESIAN_POINT('Ctrl Pts',(-30.7010733797632,-8.99756721057681,
135.732190956222));
#38597=CARTESIAN_POINT('Ctrl Pts',(-30.7759616147075,-9.00000000000003,
135.763779566847));
#38598=CARTESIAN_POINT('Ctrl Pts',(-30.8485281374251,-9.,135.800000000001));
#38599=CARTESIAN_POINT('Ctrl Pts',(-30.6134852835967,-8.96294870295619,
135.737135028007));
#38600=CARTESIAN_POINT('Ctrl Pts',(-30.688773753518,-8.96504480705121,135.763211800971));
#38601=CARTESIAN_POINT('Ctrl Pts',(-30.762348253046,-8.96666666666669,135.794239574446));
#38602=CARTESIAN_POINT('Ctrl Pts',(-30.8336416788738,-8.96666666666667,
135.829824561404));
#38603=CARTESIAN_POINT('Ctrl Pts',(-30.6025466309533,-8.9314743514781,135.768567514003));
#38604=CARTESIAN_POINT('Ctrl Pts',(-30.6764741272728,-8.9325224035256,135.79423264572));
#38605=CARTESIAN_POINT('Ctrl Pts',(-30.7487348913845,-8.93333333333334,
135.824699582045));
#38606=CARTESIAN_POINT('Ctrl Pts',(-30.8187552203225,-8.93333333333333,
135.859649122808));
#38607=CARTESIAN_POINT('Ctrl Pts',(-30.59160797831,-8.9,135.8));
#38608=CARTESIAN_POINT('Ctrl Pts',(-30.6641745010276,-8.9,135.825253490469));
#38609=CARTESIAN_POINT('Ctrl Pts',(-30.7351215297229,-8.9,135.855159589645));
#38610=CARTESIAN_POINT('Ctrl Pts',(-30.8038687617712,-8.9,135.889473684211));
#38611=CARTESIAN_POINT('Ctrl Pts',(-30.59160797831,-8.9,135.8));
#38612=CARTESIAN_POINT('Ctrl Pts',(-30.6641745010276,-8.9,135.825253490469));
#38613=CARTESIAN_POINT('Ctrl Pts',(-30.7351215297229,-8.9,135.855159589645));
#38614=CARTESIAN_POINT('Ctrl Pts',(-30.8038687617712,-8.9,135.889473684211));
#38615=CARTESIAN_POINT('Origin',(-30.,-9.1,137.5));
#38616=CARTESIAN_POINT('',(-31.8,-8.5,137.5));
#38617=CARTESIAN_POINT('',(-31.8,-9.1,137.5));
#38618=CARTESIAN_POINT('',(-28.8951880620293,-8.5,136.078947368421));
#38619=CARTESIAN_POINT('Origin',(-30.,-8.5,137.5));
#38620=CARTESIAN_POINT('',(-29.0050125628934,-8.5,136.));
#38621=CARTESIAN_POINT('Ctrl Pts',(-29.0050125628934,-8.5,136.));
#38622=CARTESIAN_POINT('Ctrl Pts',(-28.9674326867105,-8.5,136.024927669793));
#38623=CARTESIAN_POINT('Ctrl Pts',(-28.9307900499921,-8.5,136.051268237865));
#38624=CARTESIAN_POINT('Ctrl Pts',(-28.8951880620293,-8.5,136.078947368421));
#38625=CARTESIAN_POINT('',(-30.9949874371066,-8.5,136.));
#38626=CARTESIAN_POINT('Ctrl Pts',(-30.9949874371066,-8.49999999999999,
136.));
#38627=CARTESIAN_POINT('Ctrl Pts',(-30.9864258065899,-8.49999999999999,
135.994320856796));
#38628=CARTESIAN_POINT('Ctrl Pts',(-30.9778381230699,-8.49988813409469,
135.988729270797));
#38629=CARTESIAN_POINT('Ctrl Pts',(-30.9692255759031,-8.49967145659891,
135.98322540583));
#38630=CARTESIAN_POINT('Ctrl Pts',(-30.9575142878076,-8.49937681988719,
135.975741284465));
#38631=CARTESIAN_POINT('Ctrl Pts',(-30.9457625581667,-8.49890259856714,
135.968422529549));
#38632=CARTESIAN_POINT('Ctrl Pts',(-30.9339621958604,-8.49823351737353,
135.96125838821));
#38633=CARTESIAN_POINT('Ctrl Pts',(-30.7382389594249,-8.48713599907262,
135.842432466377));
#38634=CARTESIAN_POINT('Ctrl Pts',(-30.5325493637783,-8.43232113429654,
135.768015720853));
#38635=CARTESIAN_POINT('Ctrl Pts',(-30.3291860222081,-8.39687027010474,
135.730147139418));
#38636=CARTESIAN_POINT('Ctrl Pts',(-30.2613982416847,-8.38505331537414,
135.71752427894));
#38637=CARTESIAN_POINT('Ctrl Pts',(-30.1938689338364,-8.37538791626402,
135.708962325583));
#38638=CARTESIAN_POINT('Ctrl Pts',(-30.1265373999854,-8.36988598131025,
135.704221903279));
#38639=CARTESIAN_POINT('Ctrl Pts',(-30.1036817054724,-8.36801834905324,
135.702612766552));
#38640=CARTESIAN_POINT('Ctrl Pts',(-30.0808735113911,-8.36662503132802,
135.701446014506));
#38641=CARTESIAN_POINT('Ctrl Pts',(-30.058041456041,-8.3657453936638,135.700711749912));
#38642=CARTESIAN_POINT('Ctrl Pts',(-30.0470380871301,-8.36532147310216,
135.700357888462));
#38643=CARTESIAN_POINT('Ctrl Pts',(-30.0360440525282,-8.36501787270752,
135.700106267186));
#38644=CARTESIAN_POINT('Ctrl Pts',(-30.0250429177668,-8.36483405979588,
135.69995393212));
#38645=CARTESIAN_POINT('Ctrl Pts',(-29.9790828012595,-8.36406613330308,
135.699317512559));
#38646=CARTESIAN_POINT('Ctrl Pts',(-29.9332009560837,-8.36546505443064,
135.700441545649));
#38647=CARTESIAN_POINT('Ctrl Pts',(-29.8872148113109,-8.36886140284219,
135.703319027206));
#38648=CARTESIAN_POINT('Ctrl Pts',(-29.8534299813378,-8.37135661208795,
135.705433038408));
#38649=CARTESIAN_POINT('Ctrl Pts',(-29.8195500300793,-8.37490071039475,
135.708573055883));
#38650=CARTESIAN_POINT('Ctrl Pts',(-29.7857448394163,-8.37930108895748,
135.71256873066));
#38651=CARTESIAN_POINT('Ctrl Pts',(-29.5878064298017,-8.40506647934065,
135.73596447241));
#38652=CARTESIAN_POINT('Ctrl Pts',(-29.3817762259822,-8.46017177748972,
135.795991006845));
#38653=CARTESIAN_POINT('Ctrl Pts',(-29.190935014294,-8.48601923378606,135.891967734794));
#38654=CARTESIAN_POINT('Ctrl Pts',(-29.1273212770646,-8.49463505255151,
135.923959977444));
#38655=CARTESIAN_POINT('Ctrl Pts',(-29.0653952056276,-8.49999999999999,
135.95994668604));
#38656=CARTESIAN_POINT('Ctrl Pts',(-29.0050125628934,-8.49999999999999,
136.));
#38657=CARTESIAN_POINT('',(-31.1048119379707,-8.5,136.078947368421));
#38658=CARTESIAN_POINT('Ctrl Pts',(-31.1048119379707,-8.5,136.078947368421));
#38659=CARTESIAN_POINT('Ctrl Pts',(-31.0692099500079,-8.5,136.051268237865));
#38660=CARTESIAN_POINT('Ctrl Pts',(-31.0325673132895,-8.5,136.024927669793));
#38661=CARTESIAN_POINT('Ctrl Pts',(-30.9949874371066,-8.5,136.));
#38662=CARTESIAN_POINT('Origin',(-30.,-8.5,137.5));
#38663=CARTESIAN_POINT('Origin',(-30.,-8.95,142.5));
#38664=CARTESIAN_POINT('',(-29.19613123823,-8.9,144.110526315789));
#38665=CARTESIAN_POINT('',(-29.1514718625761,-9.,144.2));
#38666=CARTESIAN_POINT('',(-31.8,-8.9,142.5));
#38667=CARTESIAN_POINT('Origin',(-30.,-8.9,142.5));
#38668=CARTESIAN_POINT('',(-30.80386876177,-8.9,144.110526315789));
#38669=CARTESIAN_POINT('Origin',(-30.,-8.9,142.5));
#38670=CARTESIAN_POINT('',(-30.80386876177,-8.9,144.110526315789));
#38671=CARTESIAN_POINT('Ctrl Pts',(-30.62442393624,-8.99442305443429,144.29429745799));
#38672=CARTESIAN_POINT('Ctrl Pts',(-30.5471210576335,-8.99125209441902,
144.321011685441));
#38673=CARTESIAN_POINT('Ctrl Pts',(-30.3890975283267,-8.98340931878656,
144.364446023987));
#38674=CARTESIAN_POINT('Ctrl Pts',(-30.1466727558104,-8.97528496697549,
144.397455998416));
#38675=CARTESIAN_POINT('Ctrl Pts',(-29.917310908637,-8.97429943254969,144.401048817597));
#38676=CARTESIAN_POINT('Ctrl Pts',(-29.6784757526138,-8.98055560583611,
144.37677095198));
#38677=CARTESIAN_POINT('Ctrl Pts',(-29.5181405190621,-8.98818372075475,
144.339120021515));
#38678=CARTESIAN_POINT('Ctrl Pts',(-29.4183151210873,-8.99261764548661,
144.308633020031));
#38679=CARTESIAN_POINT('Ctrl Pts',(-29.3968663992163,-8.99354972599348,
144.301654944207));
#38680=CARTESIAN_POINT('Ctrl Pts',(-29.37557606376,-8.99442305443429,144.29429745799));
#38681=CARTESIAN_POINT('Ctrl Pts',(-30.6134852835967,-8.96294870295619,
144.262864971993));
#38682=CARTESIAN_POINT('Ctrl Pts',(-30.537876135733,-8.960832400444,144.289055422042));
#38683=CARTESIAN_POINT('Ctrl Pts',(-30.3829031149238,-8.95481445077649,
144.331914740378));
#38684=CARTESIAN_POINT('Ctrl Pts',(-30.1444415014392,-8.94813920653503,
144.364709891608));
#38685=CARTESIAN_POINT('Ctrl Pts',(-29.9185623382477,-8.94731537891439,
144.36828875045));
#38686=CARTESIAN_POINT('Ctrl Pts',(-29.6835143198945,-8.95249912929929,
144.344141487335));
#38687=CARTESIAN_POINT('Ctrl Pts',(-29.5261156183802,-8.95851695974801,
144.306903693678));
#38688=CARTESIAN_POINT('Ctrl Pts',(-29.4283364833029,-8.96171515071183,
144.276929968692));
#38689=CARTESIAN_POINT('Ctrl Pts',(-29.4073412881907,-8.96236610430249,
144.27007827294));
#38690=CARTESIAN_POINT('Ctrl Pts',(-29.3865147164033,-8.96294870295619,
144.262864971993));
#38691=CARTESIAN_POINT('Ctrl Pts',(-30.6025466309533,-8.9314743514781,144.231432485997));
#38692=CARTESIAN_POINT('Ctrl Pts',(-30.5286044265584,-8.93041969397501,
144.257099071301));
#38693=CARTESIAN_POINT('Ctrl Pts',(-30.3767148747571,-8.9262174145652,144.29938163169));
#38694=CARTESIAN_POINT('Ctrl Pts',(-30.1421910885359,-8.92099903862342,
144.331963749486));
#38695=CARTESIAN_POINT('Ctrl Pts',(-29.9198243048248,-8.9203341020548,144.335531895016));
#38696=CARTESIAN_POINT('Ctrl Pts',(-29.6885516308557,-8.92443685309091,
144.311509099425));
#38697=CARTESIAN_POINT('Ctrl Pts',(-29.5340873690899,-8.92885561901168,
144.274685263127));
#38698=CARTESIAN_POINT('Ctrl Pts',(-29.4383588129063,-8.93081117793894,
144.24522727937));
#38699=CARTESIAN_POINT('Ctrl Pts',(-29.4178154116412,-8.93118362169099,
144.238501365718));
#38700=CARTESIAN_POINT('Ctrl Pts',(-29.3974533690467,-8.9314743514781,144.231432485997));
#38701=CARTESIAN_POINT('Ctrl Pts',(-30.59160797831,-8.9,144.2));
#38702=CARTESIAN_POINT('Ctrl Pts',(-30.5193595046579,-8.9,144.225142807902));
#38703=CARTESIAN_POINT('Ctrl Pts',(-30.3705204613541,-8.89762254655513,
144.266850348081));
#38704=CARTESIAN_POINT('Ctrl Pts',(-30.1399598341647,-8.89385327818296,
144.299217642678));
#38705=CARTESIAN_POINT('Ctrl Pts',(-29.9210757344354,-8.8933500484195,144.302771827868));
#38706=CARTESIAN_POINT('Ctrl Pts',(-29.6935901981364,-8.89638037655408,
144.27887963478));
#38707=CARTESIAN_POINT('Ctrl Pts',(-29.542062468408,-8.89918885800494,144.242468935291));
#38708=CARTESIAN_POINT('Ctrl Pts',(-29.448380175122,-8.89990868316417,144.213524228031));
#38709=CARTESIAN_POINT('Ctrl Pts',(-29.4282903006156,-8.9,144.206924694451));
#38710=CARTESIAN_POINT('Ctrl Pts',(-29.40839202169,-8.9,144.2));
#38711=CARTESIAN_POINT('',(-29.40839202169,-8.9,144.2));
#38712=CARTESIAN_POINT('',(-29.40839202169,-8.9,144.2));
#38713=CARTESIAN_POINT('',(-30.59160797831,-8.9,144.2));
#38714=CARTESIAN_POINT('',(-30.62442393624,-8.99442305443429,144.29429745799));
#38715=CARTESIAN_POINT('Ctrl Pts',(-30.59160797831,-8.9,144.2));
#38716=CARTESIAN_POINT('Ctrl Pts',(-30.5193595046579,-8.9,144.225142807902));
#38717=CARTESIAN_POINT('Ctrl Pts',(-30.3705204613541,-8.89762254655513,
144.266850348081));
#38718=CARTESIAN_POINT('Ctrl Pts',(-30.1399598341647,-8.89385327818296,
144.299217642678));
#38719=CARTESIAN_POINT('Ctrl Pts',(-29.9210757344354,-8.8933500484195,144.302771827868));
#38720=CARTESIAN_POINT('Ctrl Pts',(-29.6935901981364,-8.89638037655408,
144.27887963478));
#38721=CARTESIAN_POINT('Ctrl Pts',(-29.542062468408,-8.89918885800494,144.242468935291));
#38722=CARTESIAN_POINT('Ctrl Pts',(-29.448380175122,-8.89990868316417,144.213524228031));
#38723=CARTESIAN_POINT('Ctrl Pts',(-29.4282903006156,-8.9,144.206924694451));
#38724=CARTESIAN_POINT('Ctrl Pts',(-29.40839202169,-8.9,144.2));
#38725=CARTESIAN_POINT('Ctrl Pts',(-30.8485281374239,-9.,144.2));
#38726=CARTESIAN_POINT('Ctrl Pts',(-30.7759616147067,-9.,144.236220433153));
#38727=CARTESIAN_POINT('Ctrl Pts',(-30.7010733797628,-8.99756721057679,
144.267809043778));
#38728=CARTESIAN_POINT('Ctrl Pts',(-30.62442393624,-8.99442305443429,144.29429745799));
#38729=CARTESIAN_POINT('Ctrl Pts',(-30.8336416788726,-8.96666666666667,
144.170175438596));
#38730=CARTESIAN_POINT('Ctrl Pts',(-30.7623482530451,-8.96666666666667,
144.205760425554));
#38731=CARTESIAN_POINT('Ctrl Pts',(-30.6887737535176,-8.96504480705119,
144.236788199029));
#38732=CARTESIAN_POINT('Ctrl Pts',(-30.6134852835966,-8.96294870295619,
144.262864971993));
#38733=CARTESIAN_POINT('Ctrl Pts',(-30.8187552203213,-8.93333333333333,
144.140350877193));
#38734=CARTESIAN_POINT('Ctrl Pts',(-30.7487348913836,-8.93333333333333,
144.175300417955));
#38735=CARTESIAN_POINT('Ctrl Pts',(-30.6764741272724,-8.9325224035256,144.20576735428));
#38736=CARTESIAN_POINT('Ctrl Pts',(-30.6025466309533,-8.9314743514781,144.231432485997));
#38737=CARTESIAN_POINT('Ctrl Pts',(-30.80386876177,-8.9,144.110526315789));
#38738=CARTESIAN_POINT('Ctrl Pts',(-30.7351215297221,-8.9,144.144840410356));
#38739=CARTESIAN_POINT('Ctrl Pts',(-30.6641745010272,-8.9,144.174746509531));
#38740=CARTESIAN_POINT('Ctrl Pts',(-30.59160797831,-8.9,144.2));
#38741=CARTESIAN_POINT('Ctrl Pts',(-30.80386876177,-8.9,144.110526315789));
#38742=CARTESIAN_POINT('Ctrl Pts',(-30.7351215297221,-8.9,144.144840410356));
#38743=CARTESIAN_POINT('Ctrl Pts',(-30.6641745010272,-8.9,144.174746509531));
#38744=CARTESIAN_POINT('Ctrl Pts',(-30.59160797831,-8.9,144.2));
#38745=CARTESIAN_POINT('Ctrl Pts',(-29.37557606376,-8.99442305443429,144.29429745799));
#38746=CARTESIAN_POINT('Ctrl Pts',(-29.2989266202368,-8.99756721057681,
144.267809043778));
#38747=CARTESIAN_POINT('Ctrl Pts',(-29.2240383852925,-9.00000000000003,
144.236220433153));
#38748=CARTESIAN_POINT('Ctrl Pts',(-29.1514718625749,-9.,144.199999999999));
#38749=CARTESIAN_POINT('Ctrl Pts',(-29.3865147164033,-8.96294870295619,
144.262864971993));
#38750=CARTESIAN_POINT('Ctrl Pts',(-29.311226246482,-8.96504480705121,144.236788199029));
#38751=CARTESIAN_POINT('Ctrl Pts',(-29.237651746954,-8.96666666666669,144.205760425554));
#38752=CARTESIAN_POINT('Ctrl Pts',(-29.1663583211262,-8.96666666666667,
144.170175438596));
#38753=CARTESIAN_POINT('Ctrl Pts',(-29.3974533690467,-8.9314743514781,144.231432485997));
#38754=CARTESIAN_POINT('Ctrl Pts',(-29.3235258727272,-8.9325224035256,144.20576735428));
#38755=CARTESIAN_POINT('Ctrl Pts',(-29.2512651086155,-8.93333333333334,
144.175300417955));
#38756=CARTESIAN_POINT('Ctrl Pts',(-29.1812447796775,-8.93333333333333,
144.140350877192));
#38757=CARTESIAN_POINT('Ctrl Pts',(-29.40839202169,-8.9,144.2));
#38758=CARTESIAN_POINT('Ctrl Pts',(-29.3358254989724,-8.9,144.174746509531));
#38759=CARTESIAN_POINT('Ctrl Pts',(-29.2648784702771,-8.9,144.144840410355));
#38760=CARTESIAN_POINT('Ctrl Pts',(-29.1961312382288,-8.9,144.110526315789));
#38761=CARTESIAN_POINT('Ctrl Pts',(-29.40839202169,-8.9,144.2));
#38762=CARTESIAN_POINT('Ctrl Pts',(-29.3358254989724,-8.9,144.174746509531));
#38763=CARTESIAN_POINT('Ctrl Pts',(-29.2648784702771,-8.9,144.144840410355));
#38764=CARTESIAN_POINT('Ctrl Pts',(-29.1961312382288,-8.9,144.110526315789));
#38765=CARTESIAN_POINT('Origin',(-30.,-9.1,142.5));
#38766=CARTESIAN_POINT('',(-31.8,-8.5,142.5));
#38767=CARTESIAN_POINT('',(-31.8,-9.1,142.5));
#38768=CARTESIAN_POINT('',(-31.1048119379707,-8.5,143.921052631579));
#38769=CARTESIAN_POINT('Origin',(-30.,-8.5,142.5));
#38770=CARTESIAN_POINT('',(-30.9949874371066,-8.5,144.));
#38771=CARTESIAN_POINT('Ctrl Pts',(-30.9949874371066,-8.5,144.));
#38772=CARTESIAN_POINT('Ctrl Pts',(-31.0325673132895,-8.5,143.975072330207));
#38773=CARTESIAN_POINT('Ctrl Pts',(-31.0692099500079,-8.5,143.948731762135));
#38774=CARTESIAN_POINT('Ctrl Pts',(-31.1048119379707,-8.5,143.921052631579));
#38775=CARTESIAN_POINT('',(-29.0050125628934,-8.5,144.));
#38776=CARTESIAN_POINT('Ctrl Pts',(-29.0050125628934,-8.5,144.));
#38777=CARTESIAN_POINT('Ctrl Pts',(-29.0135741934101,-8.5,144.005679143204));
#38778=CARTESIAN_POINT('Ctrl Pts',(-29.0221619253429,-8.4998882739462,144.011270538495));
#38779=CARTESIAN_POINT('Ctrl Pts',(-29.0307753006606,-8.49967147839431,
144.016774290117));
#38780=CARTESIAN_POINT('Ctrl Pts',(-29.0424877148706,-8.49937668115061,
144.024258257358));
#38781=CARTESIAN_POINT('Ctrl Pts',(-29.054233030776,-8.49890414205457,144.031576926818));
#38782=CARTESIAN_POINT('Ctrl Pts',(-29.0660434123263,-8.49823289869332,
144.038740617387));
#38783=CARTESIAN_POINT('Ctrl Pts',(-29.277590700997,-8.48620960270521,144.167056481715));
#38784=CARTESIAN_POINT('Ctrl Pts',(-29.5004115805678,-8.42327948228293,
144.243514249585));
#38785=CARTESIAN_POINT('Ctrl Pts',(-29.7197482645007,-8.38872354766437,
144.278132830397));
#38786=CARTESIAN_POINT('Ctrl Pts',(-29.7712146119589,-8.38061515600853,
144.286255921694));
#38787=CARTESIAN_POINT('Ctrl Pts',(-29.8223406852117,-8.37404368722705,
144.292034257043));
#38788=CARTESIAN_POINT('Ctrl Pts',(-29.8735668070041,-8.36986017962019,
144.295641194803));
#38789=CARTESIAN_POINT('Ctrl Pts',(-29.8964405677882,-8.36799213751804,
144.297251783865));
#38790=CARTESIAN_POINT('Ctrl Pts',(-29.9192352880058,-8.36659893094219,
144.298417568824));
#38791=CARTESIAN_POINT('Ctrl Pts',(-29.942070594606,-8.36571923963916,144.299151535527));
#38792=CARTESIAN_POINT('Ctrl Pts',(-29.95307553038,-8.36529529322757,144.299505253415));
#38793=CARTESIAN_POINT('Ctrl Pts',(-29.9640684060312,-8.36499139205626,
144.299757367469));
#38794=CARTESIAN_POINT('Ctrl Pts',(-29.9750704969496,-8.36480784914122,
144.299909021531));
#38795=CARTESIAN_POINT('Ctrl Pts',(-30.0210346080518,-8.36404105062979,
144.300542596022));
#38796=CARTESIAN_POINT('Ctrl Pts',(-30.0669049083367,-8.36543824175049,
144.299429100544));
#38797=CARTESIAN_POINT('Ctrl Pts',(-30.1129265755806,-8.36883370635998,
144.296534555326));
#38798=CARTESIAN_POINT('Ctrl Pts',(-30.1467375029954,-8.37132826629937,
144.294408007895));
#38799=CARTESIAN_POINT('Ctrl Pts',(-30.1805106645095,-8.37487119501038,
144.291330477666));
#38800=CARTESIAN_POINT('Ctrl Pts',(-30.2144446411448,-8.37927237236399,
144.287258125721));
#38801=CARTESIAN_POINT('Ctrl Pts',(-30.2556816511839,-8.384620740363,144.282309350639));
#38802=CARTESIAN_POINT('Ctrl Pts',(-30.2969770291942,-8.39120800293779,
144.275903976857));
#38803=CARTESIAN_POINT('Ctrl Pts',(-30.3383389567193,-8.39854217138171,
144.267993613037));
#38804=CARTESIAN_POINT('Ctrl Pts',(-30.4505209105317,-8.41843392679202,
144.246539098663));
#38805=CARTESIAN_POINT('Ctrl Pts',(-30.5643728486618,-8.4439522552059,144.21351409447));
#38806=CARTESIAN_POINT('Ctrl Pts',(-30.6753972898983,-8.46431943599457,
144.168549294019));
#38807=CARTESIAN_POINT('Ctrl Pts',(-30.7309095105166,-8.4745030263889,144.146066893794));
#38808=CARTESIAN_POINT('Ctrl Pts',(-30.7857148569115,-8.48339882987693,
144.120599544504));
#38809=CARTESIAN_POINT('Ctrl Pts',(-30.8389884141093,-8.4897730732797,144.092537510857));
#38810=CARTESIAN_POINT('Ctrl Pts',(-30.8922619713072,-8.49614731668247,
144.064475477209));
#38811=CARTESIAN_POINT('Ctrl Pts',(-30.9440037393079,-8.5,144.033818759205));
#38812=CARTESIAN_POINT('Ctrl Pts',(-30.9949874371066,-8.5,144.));
#38813=CARTESIAN_POINT('',(-28.8951880620293,-8.5,143.921052631579));
#38814=CARTESIAN_POINT('Ctrl Pts',(-28.8951880620293,-8.5,143.921052631579));
#38815=CARTESIAN_POINT('Ctrl Pts',(-28.9307900499921,-8.5,143.948731762135));
#38816=CARTESIAN_POINT('Ctrl Pts',(-28.9674326867105,-8.5,143.975072330207));
#38817=CARTESIAN_POINT('Ctrl Pts',(-29.0050125628934,-8.5,144.));
#38818=CARTESIAN_POINT('Origin',(-30.,-8.5,142.5));
#38819=CARTESIAN_POINT('Origin',(-37.95,-8.45,137.8));
#38820=CARTESIAN_POINT('',(-37.9,-8.4,144.));
#38821=CARTESIAN_POINT('',(-38.,-8.5,144.));
#38822=CARTESIAN_POINT('',(-37.9,-8.4,136.));
#38823=CARTESIAN_POINT('',(-37.9,-8.4,137.8));
#38824=CARTESIAN_POINT('',(-37.9,-8.4,136.));
#38825=CARTESIAN_POINT('Origin',(-37.95,-8.,144.));
#38826=CARTESIAN_POINT('',(-37.9,-8.,144.4));
#38827=CARTESIAN_POINT('',(-38.,-8.,144.5));
#38828=CARTESIAN_POINT('Origin',(-37.9,-8.,144.));
#38829=CARTESIAN_POINT('Origin',(-37.95,-7.45,144.45));
#38830=CARTESIAN_POINT('',(-37.9,-5.,144.4));
#38831=CARTESIAN_POINT('',(-38.,-5.,144.5));
#38832=CARTESIAN_POINT('',(-37.9,-7.45,144.4));
#38833=CARTESIAN_POINT('Origin',(-37.95,-5.,144.));
#38834=CARTESIAN_POINT('',(-38.,-4.50000000000002,144.));
#38835=CARTESIAN_POINT('Origin',(-37.9,-5.,144.));
#38836=CARTESIAN_POINT('Origin',(-37.95,-4.55,142.2));
#38837=CARTESIAN_POINT('',(-38.,-4.5,136.));
#38838=CARTESIAN_POINT('Origin',(-37.95,-5.,136.));
#38839=CARTESIAN_POINT('',(-37.9,-5.,135.6));
#38840=CARTESIAN_POINT('',(-38.,-5.,135.5));
#38841=CARTESIAN_POINT('Origin',(-37.9,-5.,136.));
#38842=CARTESIAN_POINT('Origin',(-37.95,-5.55,135.55));
#38843=CARTESIAN_POINT('',(-37.9,-8.,135.6));
#38844=CARTESIAN_POINT('',(-38.,-8.,135.5));
#38845=CARTESIAN_POINT('',(-37.9,-5.55,135.6));
#38846=CARTESIAN_POINT('Origin',(-37.95,-8.,136.));
#38847=CARTESIAN_POINT('Origin',(-37.9,-8.,136.));
#38848=CARTESIAN_POINT('Origin',(-38.,-5.,136.));
#38849=CARTESIAN_POINT('',(37.9,-5.,135.6));
#38850=CARTESIAN_POINT('',(-38.,-5.,135.6));
#38851=CARTESIAN_POINT('Origin',(37.9,-5.,136.));
#38852=CARTESIAN_POINT('Origin',(-38.,-4.6,135.6));
#38853=CARTESIAN_POINT('',(37.9,-8.,135.6));
#38854=CARTESIAN_POINT('',(-38.,-8.,135.6));
#38855=CARTESIAN_POINT('',(37.9,-5.55,135.6));
#38856=CARTESIAN_POINT('Origin',(-38.,-8.,136.));
#38857=CARTESIAN_POINT('',(-31.1661903789691,-8.4,136.));
#38858=CARTESIAN_POINT('',(-38.,-8.4,136.));
#38859=CARTESIAN_POINT('',(-31.0500544632573,-8.39129047171135,135.916983334517));
#38860=CARTESIAN_POINT('Ctrl Pts',(-31.0500544632573,-8.39129047171135,
135.916983334517));
#38861=CARTESIAN_POINT('Ctrl Pts',(-31.0899798045429,-8.39678689624297,
135.942890163407));
#38862=CARTESIAN_POINT('Ctrl Pts',(-31.1286105027861,-8.4,135.970783139968));
#38863=CARTESIAN_POINT('Ctrl Pts',(-31.166190378969,-8.4,136.));
#38864=CARTESIAN_POINT('',(-30.6614250203353,-8.29999999989176,135.735424868771));
#38865=CARTESIAN_POINT('Ctrl Pts',(-30.6618330135182,-8.30010233118054,
135.73532232755));
#38866=CARTESIAN_POINT('Ctrl Pts',(-30.7752047623485,-8.33157740613288,
135.770950841461));
#38867=CARTESIAN_POINT('Ctrl Pts',(-30.884493794383,-8.3621158090145,135.818341931664));
#38868=CARTESIAN_POINT('Ctrl Pts',(-30.9900545348086,-8.38157398223887,
135.880001956661));
#38869=CARTESIAN_POINT('Ctrl Pts',(-31.0016998407262,-8.38372057934385,
135.886804200101));
#38870=CARTESIAN_POINT('Ctrl Pts',(-31.013252101184,-8.38570733772648,135.893774692507));
#38871=CARTESIAN_POINT('Ctrl Pts',(-31.024762336812,-8.38753570208381,135.900923965067));
#38872=CARTESIAN_POINT('Ctrl Pts',(-31.0332270288628,-8.3888802915207,135.906181580337));
#38873=CARTESIAN_POINT('Ctrl Pts',(-31.0416572725171,-8.39013445090618,
135.911534549944));
#38874=CARTESIAN_POINT('Ctrl Pts',(-31.0500544632573,-8.39129047171137,
135.916983334517));
#38875=CARTESIAN_POINT('',(-29.338574981678,-8.29999999933447,135.735424868139));
#38876=CARTESIAN_POINT('Ctrl Pts',(-29.3385596675635,-8.29990288566524,
135.735450246581));
#38877=CARTESIAN_POINT('Ctrl Pts',(-29.4711775868139,-8.26307573905372,
135.693849975405));
#38878=CARTESIAN_POINT('Ctrl Pts',(-29.611005553036,-8.22475878909839,135.667443669536));
#38879=CARTESIAN_POINT('Ctrl Pts',(-29.7931525647518,-8.19595429131125,
135.651012005817));
#38880=CARTESIAN_POINT('Ctrl Pts',(-29.8314984033175,-8.19115568892357,
135.648342005979));
#38881=CARTESIAN_POINT('Ctrl Pts',(-29.9227100335579,-8.1831020607658,135.644103777034));
#38882=CARTESIAN_POINT('Ctrl Pts',(-29.9758741206228,-8.181174644247,135.64315190657));
#38883=CARTESIAN_POINT('Ctrl Pts',(-30.0416997940909,-8.18248038026117,
135.64382121028));
#38884=CARTESIAN_POINT('Ctrl Pts',(-30.0543921192683,-8.18289720095008,
135.644034674493));
#38885=CARTESIAN_POINT('Ctrl Pts',(-30.0933973998097,-8.18468277370442,
135.644958149228));
#38886=CARTESIAN_POINT('Ctrl Pts',(-30.1195781812265,-8.18659342326112,
135.64594828709));
#38887=CARTESIAN_POINT('Ctrl Pts',(-30.222494885632,-8.19662294325124,135.651344091598));
#38888=CARTESIAN_POINT('Ctrl Pts',(-30.3995380489843,-8.22753019248229,
135.668504490131));
#38889=CARTESIAN_POINT('Ctrl Pts',(-30.5675222793608,-8.27391945427504,
135.705706123533));
#38890=CARTESIAN_POINT('Ctrl Pts',(-30.6614853063865,-8.30000579887016,
135.73521309706));
#38891=CARTESIAN_POINT('',(-28.9499455367427,-8.39129047171135,135.916983334517));
#38892=CARTESIAN_POINT('Ctrl Pts',(-28.9499455367427,-8.39129047171135,
135.916983334517));
#38893=CARTESIAN_POINT('Ctrl Pts',(-29.0091684344659,-8.38313739956724,
135.878554671711));
#38894=CARTESIAN_POINT('Ctrl Pts',(-29.1339653847047,-8.35700091284832,
135.8092868271));
#38895=CARTESIAN_POINT('Ctrl Pts',(-29.2681120801237,-8.31946572940262,
135.757548608233));
#38896=CARTESIAN_POINT('Ctrl Pts',(-29.3385596675635,-8.29990288566524,
135.735450246581));
#38897=CARTESIAN_POINT('',(-28.9245839795016,-8.39448466110874,135.933804440104));
#38898=CARTESIAN_POINT('Ctrl Pts',(-28.9245903551729,-8.3944848309362,135.933813086825));
#38899=CARTESIAN_POINT('Ctrl Pts',(-28.9329848414562,-8.39352977637814,
135.928117215014));
#38900=CARTESIAN_POINT('Ctrl Pts',(-28.9414357816817,-8.39246198897255,
135.922505160033));
#38901=CARTESIAN_POINT('Ctrl Pts',(-28.9499455367427,-8.39129047171135,
135.916983334517));
#38902=CARTESIAN_POINT('',(-28.8338096210309,-8.4,136.));
#38903=CARTESIAN_POINT('Ctrl Pts',(-28.8338096210309,-8.4,136.));
#38904=CARTESIAN_POINT('Ctrl Pts',(-28.8633796585678,-8.39999999999971,
135.977010471143));
#38905=CARTESIAN_POINT('Ctrl Pts',(-28.8936003083676,-8.39801061970484,
135.954840619426));
#38906=CARTESIAN_POINT('Ctrl Pts',(-28.9245903551729,-8.3944848309362,135.933813086825));
#38907=CARTESIAN_POINT('',(28.8338096210309,-8.4,136.));
#38908=CARTESIAN_POINT('',(-38.,-8.4,136.));
#38909=CARTESIAN_POINT('',(28.9499455367427,-8.39129047171135,135.916983334517));
#38910=CARTESIAN_POINT('Ctrl Pts',(28.9499455367427,-8.39129047171135,135.916983334517));
#38911=CARTESIAN_POINT('Ctrl Pts',(28.9100201954571,-8.39678689624297,135.942890163407));
#38912=CARTESIAN_POINT('Ctrl Pts',(28.8713894972139,-8.4,135.970783139968));
#38913=CARTESIAN_POINT('Ctrl Pts',(28.833809621031,-8.4,136.));
#38914=CARTESIAN_POINT('',(29.3385749796647,-8.29999999989174,135.735424868771));
#38915=CARTESIAN_POINT('Ctrl Pts',(29.3382719538198,-8.30022274522941,135.735429427059));
#38916=CARTESIAN_POINT('Ctrl Pts',(29.2248680044857,-8.33165798240388,135.771014610257));
#38917=CARTESIAN_POINT('Ctrl Pts',(29.1154899444758,-8.36206527659851,135.81832752607));
#38918=CARTESIAN_POINT('Ctrl Pts',(29.009946342934,-8.3815714458719,135.880001863018));
#38919=CARTESIAN_POINT('Ctrl Pts',(28.9983029277528,-8.38372333783055,135.886805685331));
#38920=CARTESIAN_POINT('Ctrl Pts',(28.9867484811824,-8.38570649135595,135.893774768811));
#38921=CARTESIAN_POINT('Ctrl Pts',(28.9752381881508,-8.38753539124472,135.900924108674));
#38922=CARTESIAN_POINT('Ctrl Pts',(28.966773453885,-8.38888037451444,135.90618177344));
#38923=CARTESIAN_POINT('Ctrl Pts',(28.9583427274828,-8.39013445090615,135.911534549944));
#38924=CARTESIAN_POINT('Ctrl Pts',(28.9499455367427,-8.39129047171135,135.916983334517));
#38925=CARTESIAN_POINT('',(30.6614250183219,-8.29999999933448,135.735424868139));
#38926=CARTESIAN_POINT('Ctrl Pts',(30.661439935235,-8.29988734177344,135.735464277796));
#38927=CARTESIAN_POINT('Ctrl Pts',(30.4942644053416,-8.25334841832887,135.683085800293));
#38928=CARTESIAN_POINT('Ctrl Pts',(30.3161740152865,-8.20438420621798,135.655279343636));
#38929=CARTESIAN_POINT('Ctrl Pts',(30.0774858946058,-8.1831094502482,135.644290152174));
#38930=CARTESIAN_POINT('Ctrl Pts',(30.0242680337758,-8.18121722147009,135.643309689515));
#38931=CARTESIAN_POINT('Ctrl Pts',(29.9584452353951,-8.1825139216413,135.643982887837));
#38932=CARTESIAN_POINT('Ctrl Pts',(29.9457556588889,-8.18293453051425,135.644194467675));
#38933=CARTESIAN_POINT('Ctrl Pts',(29.8489117254301,-8.18734058685009,135.646496412784));
#38934=CARTESIAN_POINT('Ctrl Pts',(29.6834526291903,-8.20996395514133,135.657893063385));
#38935=CARTESIAN_POINT('Ctrl Pts',(29.4880416126676,-8.25873808016239,135.692585803548));
#38936=CARTESIAN_POINT('Ctrl Pts',(29.3751527057733,-8.28999956547834,135.723864269662));
#38937=CARTESIAN_POINT('Ctrl Pts',(29.3385835586903,-8.30013636951601,135.735331680823));
#38938=CARTESIAN_POINT('',(31.0500544632573,-8.39129047171135,135.916983334517));
#38939=CARTESIAN_POINT('Ctrl Pts',(31.0500544632573,-8.39129047171135,135.916983334517));
#38940=CARTESIAN_POINT('Ctrl Pts',(31.0166500895793,-8.38669177291417,135.895307843082));
#38941=CARTESIAN_POINT('Ctrl Pts',(30.9494673877353,-8.37449857575747,135.855365180714));
#38942=CARTESIAN_POINT('Ctrl Pts',(30.8206580127449,-8.34434635533052,135.791526200842));
#38943=CARTESIAN_POINT('Ctrl Pts',(30.7231771409772,-8.31707396647592,135.754807424752));
#38944=CARTESIAN_POINT('Ctrl Pts',(30.661439935235,-8.29988734177344,135.735464277796));
#38945=CARTESIAN_POINT('',(31.0754160204892,-8.3944846611077,135.933804440098));
#38946=CARTESIAN_POINT('Ctrl Pts',(31.0754096448179,-8.39448483093516,135.933813086818));
#38947=CARTESIAN_POINT('Ctrl Pts',(31.0670151585377,-8.39352977637736,135.92811721501));
#38948=CARTESIAN_POINT('Ctrl Pts',(31.0585642183152,-8.39246198897212,135.922505160031));
#38949=CARTESIAN_POINT('Ctrl Pts',(31.0500544632573,-8.39129047171135,135.916983334517));
#38950=CARTESIAN_POINT('',(31.1661903789691,-8.4,136.));
#38951=CARTESIAN_POINT('Ctrl Pts',(31.1661903789691,-8.4,136.));
#38952=CARTESIAN_POINT('Ctrl Pts',(31.1366203414292,-8.39999999999971,135.977010471141));
#38953=CARTESIAN_POINT('Ctrl Pts',(31.1063996916264,-8.39801061970445,135.954840619422));
#38954=CARTESIAN_POINT('Ctrl Pts',(31.0754096448179,-8.39448483093516,135.933813086818));
#38955=CARTESIAN_POINT('',(37.9,-8.4,136.));
#38956=CARTESIAN_POINT('',(-38.,-8.4,136.));
#38957=CARTESIAN_POINT('Origin',(37.9,-8.,136.));
#38958=CARTESIAN_POINT('Origin',(-38.,-8.4,135.6));
#38959=CARTESIAN_POINT('',(-31.1661903789691,-8.4,144.));
#38960=CARTESIAN_POINT('',(-38.,-8.4,144.));
#38961=CARTESIAN_POINT('',(-28.8338096210309,-8.4,144.));
#38962=CARTESIAN_POINT('Origin',(-30.,-8.4,142.5));
#38963=CARTESIAN_POINT('',(28.8338096210309,-8.4,144.));
#38964=CARTESIAN_POINT('',(-38.,-8.4,144.));
#38965=CARTESIAN_POINT('',(31.1661903789691,-8.4,144.));
#38966=CARTESIAN_POINT('Origin',(30.,-8.4,142.5));
#38967=CARTESIAN_POINT('',(37.9,-8.4,144.));
#38968=CARTESIAN_POINT('',(-38.,-8.4,144.));
#38969=CARTESIAN_POINT('',(37.9,-8.4,137.8));
#38970=CARTESIAN_POINT('Origin',(30.,-8.4,137.5));
#38971=CARTESIAN_POINT('Origin',(-30.,-8.4,137.5));
#38972=CARTESIAN_POINT('Ctrl Pts',(-31.0500544632573,-8.39129047171135,
135.916983334517));
#38973=CARTESIAN_POINT('Ctrl Pts',(-31.0416572725172,-8.39013445090615,
135.911534549944));
#38974=CARTESIAN_POINT('Ctrl Pts',(-31.0332270288628,-8.38888029152067,
135.906181580337));
#38975=CARTESIAN_POINT('Ctrl Pts',(-31.013252101184,-8.38570733772645,135.893774692507));
#38976=CARTESIAN_POINT('Ctrl Pts',(-31.0016998407262,-8.38372057934382,
135.8868042001));
#38977=CARTESIAN_POINT('Ctrl Pts',(-30.7969030955286,-8.34597008112092,
135.767178547824));
#38978=CARTESIAN_POINT('Ctrl Pts',(-30.522724535098,-8.24903543084407,135.680444681186));
#38979=CARTESIAN_POINT('Ctrl Pts',(-30.222494885632,-8.19662294325124,135.651344091598));
#38980=CARTESIAN_POINT('Ctrl Pts',(-30.1195781812265,-8.18659342326112,
135.64594828709));
#38981=CARTESIAN_POINT('Ctrl Pts',(-30.0933973998097,-8.18468277370442,
135.644958149228));
#38982=CARTESIAN_POINT('Ctrl Pts',(-30.0543921192683,-8.18289720095008,
135.644034674493));
#38983=CARTESIAN_POINT('Ctrl Pts',(-30.0416997940909,-8.18248038026117,
135.64382121028));
#38984=CARTESIAN_POINT('Ctrl Pts',(-29.9758741206228,-8.181174644247,135.64315190657));
#38985=CARTESIAN_POINT('Ctrl Pts',(-29.9227100335579,-8.1831020607658,135.644103777034));
#38986=CARTESIAN_POINT('Ctrl Pts',(-29.8314984033175,-8.19115568892357,
135.648342005979));
#38987=CARTESIAN_POINT('Ctrl Pts',(-29.7931525647518,-8.19595429131125,
135.651012005817));
#38988=CARTESIAN_POINT('Ctrl Pts',(-29.5343055319322,-8.23688803331351,
135.67436285499));
#38989=CARTESIAN_POINT('Ctrl Pts',(-29.2537770277665,-8.33190850945494,
135.742786049171));
#38990=CARTESIAN_POINT('Ctrl Pts',(-29.0091684344659,-8.38313739956724,
135.878554671711));
#38991=CARTESIAN_POINT('Ctrl Pts',(-28.9499455367427,-8.39129047171135,
135.916983334517));
#38992=CARTESIAN_POINT('Ctrl Pts',(-31.0316987878737,-8.4275269811409,135.944655556345));
#38993=CARTESIAN_POINT('Ctrl Pts',(-31.0232517541167,-8.42675447068797,
135.939129772415));
#38994=CARTESIAN_POINT('Ctrl Pts',(-31.0147571834097,-8.42588545326909,
135.933697780808));
#38995=CARTESIAN_POINT('Ctrl Pts',(-30.9946844630235,-8.42359293603059,
135.921096409853));
#38996=CARTESIAN_POINT('Ctrl Pts',(-30.9830404840594,-8.42211931541815,
135.914010922128));
#38997=CARTESIAN_POINT('Ctrl Pts',(-30.7774143949989,-8.39302212150258,
135.792260131074));
#38998=CARTESIAN_POINT('Ctrl Pts',(-30.5031878030179,-8.3040138295315,135.701370817207));
#38999=CARTESIAN_POINT('Ctrl Pts',(-30.2129394147106,-8.25623003142082,
135.670553593881));
#39000=CARTESIAN_POINT('Ctrl Pts',(-30.1143200141462,-8.24706050714476,
135.66484117304));
#39001=CARTESIAN_POINT('Ctrl Pts',(-30.0892414365264,-8.24533390764359,
135.663791948758));
#39002=CARTESIAN_POINT('Ctrl Pts',(-30.0519718185279,-8.24370245708564,
135.662813622192));
#39003=CARTESIAN_POINT('Ctrl Pts',(-30.0398405940584,-8.24332623806909,
135.662587713749));
#39004=CARTESIAN_POINT('Ctrl Pts',(-29.9769739071425,-8.24213517042753,
135.66187745256));
#39005=CARTESIAN_POINT('Ctrl Pts',(-29.9262337381129,-8.24389460327267,
135.662889336926));
#39006=CARTESIAN_POINT('Ctrl Pts',(-29.8388361258893,-8.25121736432484,
135.667375770243));
#39007=CARTESIAN_POINT('Ctrl Pts',(-29.8019759732395,-8.25561494071629,
135.670207472664));
#39008=CARTESIAN_POINT('Ctrl Pts',(-29.552197652623,-8.29287747645484,135.69488233382));
#39009=CARTESIAN_POINT('Ctrl Pts',(-29.2735131217218,-8.38080329713423,
135.767194847034));
#39010=CARTESIAN_POINT('Ctrl Pts',(-29.0279258537172,-8.42207265865228,
135.90569558041));
#39011=CARTESIAN_POINT('Ctrl Pts',(-28.9683012121262,-8.4275269811409,135.944655556345));
#39012=CARTESIAN_POINT('Ctrl Pts',(-31.0133431124902,-8.46376349057045,
135.972327778172));
#39013=CARTESIAN_POINT('Ctrl Pts',(-31.0048313249904,-8.46337998021818,
135.966725634326));
#39014=CARTESIAN_POINT('Ctrl Pts',(-30.996307968523,-8.46288297234629,135.961213070326));
#39015=CARTESIAN_POINT('Ctrl Pts',(-30.9760819259681,-8.46149122158306,
135.948419567118));
#39016=CARTESIAN_POINT('Ctrl Pts',(-30.9644219148336,-8.46050386249282,
135.941215807521));
#39017=CARTESIAN_POINT('Ctrl Pts',(-30.7577276599546,-8.44008395869097,
135.817350883126));
#39018=CARTESIAN_POINT('Ctrl Pts',(-30.4835228973095,-8.3590711140171,135.722284002991));
#39019=CARTESIAN_POINT('Ctrl Pts',(-30.2034244047578,-8.31578082809446,
135.6897528233));
#39020=CARTESIAN_POINT('Ctrl Pts',(-30.1089398725528,-8.30755126516961,
135.683719880602));
#39021=CARTESIAN_POINT('Ctrl Pts',(-30.0850294746744,-8.30597389738886,
135.682612214976));
#39022=CARTESIAN_POINT('Ctrl Pts',(-30.0494583878705,-8.30451621696662,
135.681578940764));
#39023=CARTESIAN_POINT('Ctrl Pts',(-30.0379032525606,-8.30417201489962,
135.681339763716));
#39024=CARTESIAN_POINT('Ctrl Pts',(-29.9779830147398,-8.30310560712257,
135.68059196657));
#39025=CARTESIAN_POINT('Ctrl Pts',(-29.9296772515286,-8.30467251192379,
135.681655985758));
#39026=CARTESIAN_POINT('Ctrl Pts',(-29.846092258766,-8.31129493668671,135.686399274144));
#39027=CARTESIAN_POINT('Ctrl Pts',(-29.8107266215916,-8.31524006098973,
135.689377589036));
#39028=CARTESIAN_POINT('Ctrl Pts',(-29.5699143091109,-8.34907703619935,
135.71544499358));
#39029=CARTESIAN_POINT('Ctrl Pts',(-29.2933633974204,-8.42964542252681,
135.791591053793));
#39030=CARTESIAN_POINT('Ctrl Pts',(-29.0466377863763,-8.46106474091497,
135.93280577734));
#39031=CARTESIAN_POINT('Ctrl Pts',(-28.9866568875098,-8.46376349057045,
135.972327778172));
#39032=CARTESIAN_POINT('Ctrl Pts',(-30.9949874371066,-8.5,136.));
#39033=CARTESIAN_POINT('Ctrl Pts',(-30.9864258065899,-8.5,135.994320856796));
#39034=CARTESIAN_POINT('Ctrl Pts',(-30.9778381230699,-8.4998881340947,135.988729270797));
#39035=CARTESIAN_POINT('Ctrl Pts',(-30.9575142878075,-8.4993768198872,135.975741284465));
#39036=CARTESIAN_POINT('Ctrl Pts',(-30.9457625581667,-8.49890259856716,
135.968422529549));
#39037=CARTESIAN_POINT('Ctrl Pts',(-30.7382389594249,-8.48713599907263,
135.842432466377));
#39038=CARTESIAN_POINT('Ctrl Pts',(-30.4639861652294,-8.41404951270454,
135.743210139011));
#39039=CARTESIAN_POINT('Ctrl Pts',(-30.1938689338364,-8.37538791626404,
135.708962325583));
#39040=CARTESIAN_POINT('Ctrl Pts',(-30.1036817054724,-8.36801834905326,
135.702612766552));
#39041=CARTESIAN_POINT('Ctrl Pts',(-30.0808735113911,-8.36662503132804,
135.701446014506));
#39042=CARTESIAN_POINT('Ctrl Pts',(-30.0470380871301,-8.36532147310218,
135.700357888462));
#39043=CARTESIAN_POINT('Ctrl Pts',(-30.0360440525282,-8.36501787270754,
135.700106267186));
#39044=CARTESIAN_POINT('Ctrl Pts',(-29.9790828012595,-8.3640661333031,135.699317512559));
#39045=CARTESIAN_POINT('Ctrl Pts',(-29.9332009560837,-8.36546505443066,
135.700441545649));
#39046=CARTESIAN_POINT('Ctrl Pts',(-29.8534299813378,-8.37135661208798,
135.705433038408));
#39047=CARTESIAN_POINT('Ctrl Pts',(-29.8195500300793,-8.37490071039478,
135.708573055883));
#39048=CARTESIAN_POINT('Ctrl Pts',(-29.5878064298017,-8.40506647934067,
135.73596447241));
#39049=CARTESIAN_POINT('Ctrl Pts',(-29.3130994913757,-8.4785402102061,135.815999851656));
#39050=CARTESIAN_POINT('Ctrl Pts',(-29.0653952056276,-8.5,135.95994668604));
#39051=CARTESIAN_POINT('Ctrl Pts',(-29.0050125628934,-8.5,136.));
#39052=CARTESIAN_POINT('',(-31.0500544632573,-8.39129047171135,135.916983334517));
#39053=CARTESIAN_POINT('',(-29.0050125628934,-8.5,136.));
#39054=CARTESIAN_POINT('Origin',(-30.,-8.45,137.5));
#39055=CARTESIAN_POINT('',(-28.8338096210309,-8.4,136.));
#39056=CARTESIAN_POINT('',(-31.1048119379707,-8.5,136.078947368421));
#39057=CARTESIAN_POINT('Ctrl Pts',(-28.9499455367427,-8.39129047171135,
135.916983334517));
#39058=CARTESIAN_POINT('Ctrl Pts',(-28.9100201948423,-8.39678689632762,
135.942890163806));
#39059=CARTESIAN_POINT('Ctrl Pts',(-28.8713894960226,-8.40000000009859,
135.970783140825));
#39060=CARTESIAN_POINT('Ctrl Pts',(-28.8338096192947,-8.4,136.00000000135));
#39061=CARTESIAN_POINT('Ctrl Pts',(-28.9683012121262,-8.4275269811409,135.944655556345));
#39062=CARTESIAN_POINT('Ctrl Pts',(-28.9291576919387,-8.43119126421841,
135.970235999263));
#39063=CARTESIAN_POINT('Ctrl Pts',(-28.8911896803029,-8.43333333339906,
135.997611506775));
#39064=CARTESIAN_POINT('Ctrl Pts',(-28.854269099658,-8.43333333333333,136.0263157908));
#39065=CARTESIAN_POINT('Ctrl Pts',(-28.9866568875098,-8.46376349057045,
135.972327778172));
#39066=CARTESIAN_POINT('Ctrl Pts',(-28.9482951890352,-8.46559563210921,
135.99758183472));
#39067=CARTESIAN_POINT('Ctrl Pts',(-28.9109898645832,-8.46666666669953,
136.024439872726));
#39068=CARTESIAN_POINT('Ctrl Pts',(-28.8747285800212,-8.46666666666667,
136.05263158025));
#39069=CARTESIAN_POINT('Ctrl Pts',(-29.0050125628934,-8.5,136.));
#39070=CARTESIAN_POINT('Ctrl Pts',(-28.9674326861317,-8.5,136.024927670177));
#39071=CARTESIAN_POINT('Ctrl Pts',(-28.9307900488635,-8.5,136.051268238676));
#39072=CARTESIAN_POINT('Ctrl Pts',(-28.8951880603845,-8.5,136.0789473697));
#39073=CARTESIAN_POINT('Ctrl Pts',(-31.166190378969,-8.4,136.));
#39074=CARTESIAN_POINT('Ctrl Pts',(-31.1286105027861,-8.4,135.970783139968));
#39075=CARTESIAN_POINT('Ctrl Pts',(-31.0899798045429,-8.39678689624297,
135.942890163407));
#39076=CARTESIAN_POINT('Ctrl Pts',(-31.0500544632573,-8.39129047171135,
135.916983334517));
#39077=CARTESIAN_POINT('Ctrl Pts',(-31.1457308986363,-8.43333333333333,
136.026315789474));
#39078=CARTESIAN_POINT('Ctrl Pts',(-31.1088103185267,-8.43333333333333,
135.997611505934));
#39079=CARTESIAN_POINT('Ctrl Pts',(-31.0708423074584,-8.43119126416198,
135.970235998869));
#39080=CARTESIAN_POINT('Ctrl Pts',(-31.0316987878737,-8.4275269811409,135.944655556345));
#39081=CARTESIAN_POINT('Ctrl Pts',(-31.1252714183035,-8.46666666666667,
136.052631578947));
#39082=CARTESIAN_POINT('Ctrl Pts',(-31.0890101342673,-8.46666666666667,
136.024439871899));
#39083=CARTESIAN_POINT('Ctrl Pts',(-31.051704810374,-8.46559563208099,135.997581834331));
#39084=CARTESIAN_POINT('Ctrl Pts',(-31.0133431124902,-8.46376349057045,
135.972327778172));
#39085=CARTESIAN_POINT('Ctrl Pts',(-31.1048119379707,-8.5,136.078947368421));
#39086=CARTESIAN_POINT('Ctrl Pts',(-31.0692099500079,-8.5,136.051268237865));
#39087=CARTESIAN_POINT('Ctrl Pts',(-31.0325673132895,-8.5,136.024927669793));
#39088=CARTESIAN_POINT('Ctrl Pts',(-30.9949874371066,-8.5,136.));
#39089=CARTESIAN_POINT('Origin',(37.95,-8.45,137.8));
#39090=CARTESIAN_POINT('',(37.9,-8.4,144.));
#39091=CARTESIAN_POINT('',(38.,-8.5,136.));
#39092=CARTESIAN_POINT('Origin',(37.95,-8.,144.));
#39093=CARTESIAN_POINT('',(37.9,-8.,144.4));
#39094=CARTESIAN_POINT('Origin',(37.9,-8.,144.));
#39095=CARTESIAN_POINT('',(37.9,-8.,144.4));
#39096=CARTESIAN_POINT('Origin',(37.95,-7.45,144.45));
#39097=CARTESIAN_POINT('',(37.9,-5.,144.4));
#39098=CARTESIAN_POINT('',(37.9,-5.,144.4));
#39099=CARTESIAN_POINT('',(37.9,-7.45,144.4));
#39100=CARTESIAN_POINT('Origin',(37.95,-5.,144.));
#39101=CARTESIAN_POINT('Origin',(37.9,-5.,144.));
#39102=CARTESIAN_POINT('',(37.9,-4.6,144.));
#39103=CARTESIAN_POINT('Origin',(37.95,-4.55,142.2));
#39104=CARTESIAN_POINT('',(37.9,-4.6,136.));
#39105=CARTESIAN_POINT('Origin',(37.95,-5.,136.));
#39106=CARTESIAN_POINT('',(37.9,-5.,135.6));
#39107=CARTESIAN_POINT('Origin',(37.95,-5.55,135.55));
#39108=CARTESIAN_POINT('',(37.9,-8.,135.6));
#39109=CARTESIAN_POINT('Origin',(37.95,-8.,136.));
#39110=CARTESIAN_POINT('Origin',(-38.,-5.,144.));
#39111=CARTESIAN_POINT('',(-38.,-5.,144.4));
#39112=CARTESIAN_POINT('Origin',(-38.,-8.4,144.4));
#39113=CARTESIAN_POINT('',(-38.,-8.,144.4));
#39114=CARTESIAN_POINT('Origin',(-38.,-8.,144.));
#39115=CARTESIAN_POINT('',(31.0500544632573,-8.39129047171135,144.083016665483));
#39116=CARTESIAN_POINT('Ctrl Pts',(31.0500544632573,-8.39129047171134,144.083016665483));
#39117=CARTESIAN_POINT('Ctrl Pts',(31.0899798045429,-8.39678689624297,144.057109836593));
#39118=CARTESIAN_POINT('Ctrl Pts',(31.1286105027861,-8.4,144.029216860032));
#39119=CARTESIAN_POINT('Ctrl Pts',(31.166190378969,-8.4,144.));
#39120=CARTESIAN_POINT('',(30.6614250203353,-8.29999999989175,144.264575131229));
#39121=CARTESIAN_POINT('Ctrl Pts',(30.6618125705925,-8.30021236907056,144.264595259035));
#39122=CARTESIAN_POINT('Ctrl Pts',(30.7752011548794,-8.33164973325584,144.228998875671));
#39123=CARTESIAN_POINT('Ctrl Pts',(30.8844471797781,-8.36205371033993,144.18170673564));
#39124=CARTESIAN_POINT('Ctrl Pts',(30.990050453113,-8.38157059509137,144.120000581026));
#39125=CARTESIAN_POINT('Ctrl Pts',(31.0017004511988,-8.38372366916582,144.113193248635));
#39126=CARTESIAN_POINT('Ctrl Pts',(31.0132504414343,-8.38570616125813,144.106226170536));
#39127=CARTESIAN_POINT('Ctrl Pts',(31.0247614073442,-8.38753522038424,144.099076369329));
#39128=CARTESIAN_POINT('Ctrl Pts',(31.0332266364484,-8.38888032075799,144.093818365289));
#39129=CARTESIAN_POINT('Ctrl Pts',(31.0416572725171,-8.39013445090616,144.088465450056));
#39130=CARTESIAN_POINT('Ctrl Pts',(31.0500544632573,-8.39129047171136,144.083016665483));
#39131=CARTESIAN_POINT('',(29.338574981678,-8.29999999933449,144.264575131861));
#39132=CARTESIAN_POINT('Ctrl Pts',(29.3385708495646,-8.29992765643484,144.264531198596));
#39133=CARTESIAN_POINT('Ctrl Pts',(29.4712387553426,-8.2631077339495,144.306139218458));
#39134=CARTESIAN_POINT('Ctrl Pts',(29.61111819365,-8.22479704106424,144.332544752617));
#39135=CARTESIAN_POINT('Ctrl Pts',(29.7743380762458,-8.1989686017083,144.347220946225));
#39136=CARTESIAN_POINT('Ctrl Pts',(29.8124450528999,-8.19359284366967,144.350292014722));
#39137=CARTESIAN_POINT('Ctrl Pts',(29.8508694789328,-8.18947694445684,144.352489515548));
#39138=CARTESIAN_POINT('Ctrl Pts',(29.8965215329261,-8.18546023959715,144.35462295684));
#39139=CARTESIAN_POINT('Ctrl Pts',(29.949327590037,-8.18215812697606,144.356319671809));
#39140=CARTESIAN_POINT('Ctrl Pts',(30.0025425983683,-8.18173837270729,144.356528098816));
#39141=CARTESIAN_POINT('Ctrl Pts',(30.0386195894541,-8.18245156556629,144.356161937062));
#39142=CARTESIAN_POINT('Ctrl Pts',(30.0513226380827,-8.18282772898188,144.355968145438));
#39143=CARTESIAN_POINT('Ctrl Pts',(30.0640055623709,-8.18336746578261,144.355691316105));
#39144=CARTESIAN_POINT('Ctrl Pts',(30.2356236626453,-8.19124684145658,144.351553122611));
#39145=CARTESIAN_POINT('Ctrl Pts',(30.4360870224364,-8.23769662979138,144.328510834346));
#39146=CARTESIAN_POINT('Ctrl Pts',(30.6248943138717,-8.28997674496655,144.276175839712));
#39147=CARTESIAN_POINT('Ctrl Pts',(30.6614381003711,-8.30010854638129,144.264712770237));
#39148=CARTESIAN_POINT('',(28.9499455367427,-8.39129047171135,144.083016665483));
#39149=CARTESIAN_POINT('Ctrl Pts',(28.9499455367427,-8.39129047171135,144.083016665483));
#39150=CARTESIAN_POINT('Ctrl Pts',(29.0091684344659,-8.38313739956724,144.121445328289));
#39151=CARTESIAN_POINT('Ctrl Pts',(29.1339413896373,-8.35700182937075,144.190695469215));
#39152=CARTESIAN_POINT('Ctrl Pts',(29.2681157510772,-8.31948137780997,144.242434692888));
#39153=CARTESIAN_POINT('Ctrl Pts',(29.3385708495646,-8.29992765643484,144.264531198596));
#39154=CARTESIAN_POINT('',(28.9245839794983,-8.39448466110912,144.066195559894));
#39155=CARTESIAN_POINT('Ctrl Pts',(28.9245903551696,-8.39448483093658,144.066186913173));
#39156=CARTESIAN_POINT('Ctrl Pts',(28.932984841454,-8.39352977637842,144.071882784984));
#39157=CARTESIAN_POINT('Ctrl Pts',(28.9414357816806,-8.39246198897271,144.077494839966));
#39158=CARTESIAN_POINT('Ctrl Pts',(28.9499455367427,-8.39129047171135,144.083016665483));
#39159=CARTESIAN_POINT('Ctrl Pts',(28.8338096210309,-8.4,144.));
#39160=CARTESIAN_POINT('Ctrl Pts',(28.8633796585668,-8.39999999999971,144.022989528856));
#39161=CARTESIAN_POINT('Ctrl Pts',(28.8936003083654,-8.39801061970499,144.045159380572));
#39162=CARTESIAN_POINT('Ctrl Pts',(28.9245903551696,-8.39448483093658,144.066186913173));
#39163=CARTESIAN_POINT('',(-28.9499455367427,-8.39129047171135,144.083016665483));
#39164=CARTESIAN_POINT('Ctrl Pts',(-28.9499455367427,-8.39129047171135,
144.083016665483));
#39165=CARTESIAN_POINT('Ctrl Pts',(-28.9100201954571,-8.39678689624297,
144.057109836593));
#39166=CARTESIAN_POINT('Ctrl Pts',(-28.8713894972139,-8.4,144.029216860032));
#39167=CARTESIAN_POINT('Ctrl Pts',(-28.833809621031,-8.4,144.));
#39168=CARTESIAN_POINT('',(-29.3385749796646,-8.29999999989175,144.264575131229));
#39169=CARTESIAN_POINT('Ctrl Pts',(-29.3383110933769,-8.30003007418734,
144.264639748776));
#39170=CARTESIAN_POINT('Ctrl Pts',(-29.2249006798342,-8.33151072678332,
144.229030421918));
#39171=CARTESIAN_POINT('Ctrl Pts',(-29.1155604606526,-8.36207385241182,
144.181653095174));
#39172=CARTESIAN_POINT('Ctrl Pts',(-29.009948502526,-8.38157138568459,144.119997209092));
#39173=CARTESIAN_POINT('Ctrl Pts',(-28.9982975463468,-8.38372232493232,
144.113195422252));
#39174=CARTESIAN_POINT('Ctrl Pts',(-28.9867489659987,-8.38570638741796,
144.10622492921));
#39175=CARTESIAN_POINT('Ctrl Pts',(-28.9752381128004,-8.38753526296663,
144.099075788646));
#39176=CARTESIAN_POINT('Ctrl Pts',(-28.9667729665849,-8.38888022833652,
144.093818270446));
#39177=CARTESIAN_POINT('Ctrl Pts',(-28.9583427274829,-8.39013445090614,
144.088465450056));
#39178=CARTESIAN_POINT('Ctrl Pts',(-28.9499455367427,-8.39129047171134,
144.083016665483));
#39179=CARTESIAN_POINT('',(-30.6614250183219,-8.29999999933447,144.264575131861));
#39180=CARTESIAN_POINT('Ctrl Pts',(-30.6614343690749,-8.30004553356604,
144.264645137541));
#39181=CARTESIAN_POINT('Ctrl Pts',(-30.5707184122875,-8.27491838180028,
144.293105800203));
#39182=CARTESIAN_POINT('Ctrl Pts',(-30.4769220075146,-8.24904042442226,
144.314236285244));
#39183=CARTESIAN_POINT('Ctrl Pts',(-30.3362573241971,-8.21797318024007,
144.335720743413));
#39184=CARTESIAN_POINT('Ctrl Pts',(-30.2909203211106,-8.20912670855604,
144.341198190437));
#39185=CARTESIAN_POINT('Ctrl Pts',(-30.2069857608087,-8.19595190722736,
144.348893235529));
#39186=CARTESIAN_POINT('Ctrl Pts',(-30.1687494835259,-8.19113640094687,
144.351508081756));
#39187=CARTESIAN_POINT('Ctrl Pts',(-30.0774739256815,-8.18309698929938,
144.355772172055));
#39188=CARTESIAN_POINT('Ctrl Pts',(-30.0243207374447,-8.18117200076953,
144.35671442715));
#39189=CARTESIAN_POINT('Ctrl Pts',(-29.9584929581617,-8.18247823187435,
144.356048044385));
#39190=CARTESIAN_POINT('Ctrl Pts',(-29.945800622645,-8.18289510415931,144.355834150072));
#39191=CARTESIAN_POINT('Ctrl Pts',(-29.9067939860508,-8.18468265252138,
144.354910990812));
#39192=CARTESIAN_POINT('Ctrl Pts',(-29.8806159996987,-8.18658920666495,
144.35392173636));
#39193=CARTESIAN_POINT('Ctrl Pts',(-29.7961080426536,-8.19484695032281,
144.349486882414));
#39194=CARTESIAN_POINT('Ctrl Pts',(-29.7387539667785,-8.2037212977524,144.344577795757));
#39195=CARTESIAN_POINT('Ctrl Pts',(-29.5636487905334,-8.23768920458241,
144.322949985584));
#39196=CARTESIAN_POINT('Ctrl Pts',(-29.4491527367723,-8.26926273488951,
144.29942619088));
#39197=CARTESIAN_POINT('Ctrl Pts',(-29.3385291537654,-8.29996954488366,
144.264708200695));
#39198=CARTESIAN_POINT('',(-31.0500544632573,-8.39129047171135,144.083016665483));
#39199=CARTESIAN_POINT('Ctrl Pts',(-31.0500544632573,-8.39129047171135,
144.083016665483));
#39200=CARTESIAN_POINT('Ctrl Pts',(-31.0000499887335,-8.38440647744572,
144.115463660888));
#39201=CARTESIAN_POINT('Ctrl Pts',(-30.8980141119118,-8.36393098595595,
144.173469870658));
#39202=CARTESIAN_POINT('Ctrl Pts',(-30.7654955980711,-8.32889312403532,
144.230056244874));
#39203=CARTESIAN_POINT('Ctrl Pts',(-30.6852039930454,-8.3066294132943,144.257187802874));
#39204=CARTESIAN_POINT('Ctrl Pts',(-30.6614343690749,-8.30004553356604,
144.264645137541));
#39205=CARTESIAN_POINT('',(-31.0754160204959,-8.39448466110846,144.066195559898));
#39206=CARTESIAN_POINT('Ctrl Pts',(-31.0754096448245,-8.39448483093591,
144.066186913177));
#39207=CARTESIAN_POINT('Ctrl Pts',(-31.0670151585421,-8.39352977637793,
144.071882784987));
#39208=CARTESIAN_POINT('Ctrl Pts',(-31.0585642183174,-8.39246198897244,
144.077494839967));
#39209=CARTESIAN_POINT('Ctrl Pts',(-31.0500544632573,-8.39129047171135,
144.083016665483));
#39210=CARTESIAN_POINT('Ctrl Pts',(-31.1661903789691,-8.4,144.));
#39211=CARTESIAN_POINT('Ctrl Pts',(-31.1366203414314,-8.3999999999997,144.022989528858));
#39212=CARTESIAN_POINT('Ctrl Pts',(-31.1063996916308,-8.39801061970473,
144.045159380575));
#39213=CARTESIAN_POINT('Ctrl Pts',(-31.0754096448245,-8.39448483093591,
144.066186913177));
#39214=CARTESIAN_POINT('Ctrl Pts',(31.0500544632573,-8.39129047171135,144.083016665483));
#39215=CARTESIAN_POINT('Ctrl Pts',(31.0416572725172,-8.39013445090615,144.088465450056));
#39216=CARTESIAN_POINT('Ctrl Pts',(31.0332266364484,-8.38888032075798,144.093818365289));
#39217=CARTESIAN_POINT('Ctrl Pts',(31.0132504414343,-8.38570616125812,144.106226170536));
#39218=CARTESIAN_POINT('Ctrl Pts',(31.0017004511988,-8.38372366916581,144.113193248635));
#39219=CARTESIAN_POINT('Ctrl Pts',(30.8502989952168,-8.35574267317688,144.201660218991));
#39220=CARTESIAN_POINT('Ctrl Pts',(30.558037054575,-8.2659539292109,144.314493271249));
#39221=CARTESIAN_POINT('Ctrl Pts',(30.2356236626453,-8.19124684145658,144.351553122611));
#39222=CARTESIAN_POINT('Ctrl Pts',(30.0640055623709,-8.18336746578261,144.355691316105));
#39223=CARTESIAN_POINT('Ctrl Pts',(30.0513226380827,-8.18282772898188,144.355968145438));
#39224=CARTESIAN_POINT('Ctrl Pts',(30.0386195894541,-8.18245156556629,144.356161937062));
#39225=CARTESIAN_POINT('Ctrl Pts',(30.0025425983683,-8.18173837270729,144.356528098816));
#39226=CARTESIAN_POINT('Ctrl Pts',(29.949327590037,-8.18215812697606,144.356319671809));
#39227=CARTESIAN_POINT('Ctrl Pts',(29.8965215329261,-8.18546023959715,144.35462295684));
#39228=CARTESIAN_POINT('Ctrl Pts',(29.8508694789328,-8.18947694445684,144.352489515548));
#39229=CARTESIAN_POINT('Ctrl Pts',(29.8124450528999,-8.19359284366967,144.350292014722));
#39230=CARTESIAN_POINT('Ctrl Pts',(29.7743380762458,-8.1989686017083,144.347220946225));
#39231=CARTESIAN_POINT('Ctrl Pts',(29.5344604689754,-8.23692760605077,144.325651942801));
#39232=CARTESIAN_POINT('Ctrl Pts',(29.2537520091736,-8.33190569493299,144.257191468094));
#39233=CARTESIAN_POINT('Ctrl Pts',(29.0091684344659,-8.38313739956724,144.121445328289));
#39234=CARTESIAN_POINT('Ctrl Pts',(28.9499455367427,-8.39129047171135,144.083016665483));
#39235=CARTESIAN_POINT('Ctrl Pts',(31.0316987878737,-8.4275269811409,144.055344443655));
#39236=CARTESIAN_POINT('Ctrl Pts',(31.0232527754724,-8.42675875494622,144.060869589794));
#39237=CARTESIAN_POINT('Ctrl Pts',(31.0147553444553,-8.42587943776685,144.066303064911));
#39238=CARTESIAN_POINT('Ctrl Pts',(30.9946853864034,-8.42360243871762,144.07890286189));
#39239=CARTESIAN_POINT('Ctrl Pts',(30.9830372481524,-8.42210831653301,144.085988643756));
#39240=CARTESIAN_POINT('Ctrl Pts',(30.8310662630449,-8.40062314502122,144.176010199841));
#39241=CARTESIAN_POINT('Ctrl Pts',(30.5383283564013,-8.32003419197623,144.292952674175));
#39242=CARTESIAN_POINT('Ctrl Pts',(30.2247435582948,-8.25116314278318,144.33256898185));
#39243=CARTESIAN_POINT('Ctrl Pts',(30.0611760154067,-8.24414097291916,144.336897172084));
#39244=CARTESIAN_POINT('Ctrl Pts',(30.0490244691322,-8.24363821830494,144.337194280782));
#39245=CARTESIAN_POINT('Ctrl Pts',(30.0369088739531,-8.24330388773372,144.337397022135));
#39246=CARTESIAN_POINT('Ctrl Pts',(30.0024432035511,-8.24265189581713,144.337786084088));
#39247=CARTESIAN_POINT('Ctrl Pts',(29.9516451181674,-8.24303779805442,144.337563550915));
#39248=CARTESIAN_POINT('Ctrl Pts',(29.9011427210787,-8.24603722149251,144.335767184191));
#39249=CARTESIAN_POINT('Ctrl Pts',(29.857399378596,-8.2497015555049,144.333505775426));
#39250=CARTESIAN_POINT('Ctrl Pts',(29.8205273527128,-8.25344039474353,144.331181766681));
#39251=CARTESIAN_POINT('Ctrl Pts',(29.7838223086098,-8.25836498371357,144.327927772113));
#39252=CARTESIAN_POINT('Ctrl Pts',(29.5523533776709,-8.29291263025922,144.305133904073));
#39253=CARTESIAN_POINT('Ctrl Pts',(29.2734876151046,-8.38080321331592,144.232781780034));
#39254=CARTESIAN_POINT('Ctrl Pts',(29.0279259955364,-8.42207186623694,144.094304677965));
#39255=CARTESIAN_POINT('Ctrl Pts',(28.9683012121263,-8.4275269811409,144.055344443655));
#39256=CARTESIAN_POINT('Ctrl Pts',(31.0133431124902,-8.46376349057045,144.027672221828));
#39257=CARTESIAN_POINT('Ctrl Pts',(31.0048303036347,-8.46337569595993,144.033275003465));
#39258=CARTESIAN_POINT('Ctrl Pts',(30.9963094453813,-8.4628889223465,144.038785971762));
#39259=CARTESIAN_POINT('Ctrl Pts',(30.9760797687839,-8.46148171290697,144.051582436227));
#39260=CARTESIAN_POINT('Ctrl Pts',(30.9644249961142,-8.46051430961044,144.058780581885));
#39261=CARTESIAN_POINT('Ctrl Pts',(30.811663986886,-8.44541570746616,144.150365816204));
#39262=CARTESIAN_POINT('Ctrl Pts',(30.5184370781297,-8.37405874016662,144.271435163949));
#39263=CARTESIAN_POINT('Ctrl Pts',(30.2145450560986,-8.31126754234417,144.313519514008));
#39264=CARTESIAN_POINT('Ctrl Pts',(30.0580521168044,-8.30480713431659,144.318143569817));
#39265=CARTESIAN_POINT('Ctrl Pts',(30.0465137000413,-8.30437370070772,144.318450715706));
#39266=CARTESIAN_POINT('Ctrl Pts',(30.034933916069,-8.30406014627328,144.318669166289));
#39267=CARTESIAN_POINT('Ctrl Pts',(30.0020987157711,-8.30347844330574,144.31907802629));
#39268=CARTESIAN_POINT('Ctrl Pts',(29.9537071077953,-8.30381904774098,144.318845302261));
#39269=CARTESIAN_POINT('Ctrl Pts',(29.9055195030814,-8.30653012524895,144.316944860243));
#39270=CARTESIAN_POINT('Ctrl Pts',(29.8636848030784,-8.30982716472501,144.3145602471));
#39271=CARTESIAN_POINT('Ctrl Pts',(29.8283694070157,-8.31322211431118,144.31209976428));
#39272=CARTESIAN_POINT('Ctrl Pts',(29.7930638488286,-8.31764796375963,144.308677235497));
#39273=CARTESIAN_POINT('Ctrl Pts',(29.5699541610066,-8.3490326254289,144.284592127057));
#39274=CARTESIAN_POINT('Ctrl Pts',(29.2933240301876,-8.42964020165404,144.20838609147));
#39275=CARTESIAN_POINT('Ctrl Pts',(29.0466376445571,-8.4610655333303,144.067193964284));
#39276=CARTESIAN_POINT('Ctrl Pts',(28.9866568875098,-8.46376349057045,144.027672221828));
#39277=CARTESIAN_POINT('Ctrl Pts',(30.9949874371066,-8.5,144.));
#39278=CARTESIAN_POINT('Ctrl Pts',(30.9864258065899,-8.5,144.005679143204));
#39279=CARTESIAN_POINT('Ctrl Pts',(30.9778381533882,-8.49988803935537,144.011270671384));
#39280=CARTESIAN_POINT('Ctrl Pts',(30.957514713753,-8.49937799036647,144.024259127581));
#39281=CARTESIAN_POINT('Ctrl Pts',(30.9457617930679,-8.49889895697764,144.031575977005));
#39282=CARTESIAN_POINT('Ctrl Pts',(30.7924312547142,-8.4902961793105,144.124715797054));
#39283=CARTESIAN_POINT('Ctrl Pts',(30.4987283799559,-8.42813900293195,144.249894566875));
#39284=CARTESIAN_POINT('Ctrl Pts',(30.203664951748,-8.37118384367076,144.294535373247));
#39285=CARTESIAN_POINT('Ctrl Pts',(30.0552225698401,-8.36558064145315,144.299349425796));
#39286=CARTESIAN_POINT('Ctrl Pts',(30.0442155310909,-8.36518419003078,144.29967685105));
#39287=CARTESIAN_POINT('Ctrl Pts',(30.033223200568,-8.36491246844071,144.299904251363));
#39288=CARTESIAN_POINT('Ctrl Pts',(30.0019993209539,-8.36439196641558,144.300336011563));
#39289=CARTESIAN_POINT('Ctrl Pts',(29.9560246359257,-8.36469871881934,144.300089181366));
#39290=CARTESIAN_POINT('Ctrl Pts',(29.910140691234,-8.36710710714431,144.298089087593));
#39291=CARTESIAN_POINT('Ctrl Pts',(29.8702147027416,-8.37005177577307,144.295576506978));
#39292=CARTESIAN_POINT('Ctrl Pts',(29.8364517068287,-8.37306966538504,144.29298951624));
#39293=CARTESIAN_POINT('Ctrl Pts',(29.8025480811926,-8.3770443457649,144.289384061385));
#39294=CARTESIAN_POINT('Ctrl Pts',(29.5878470697021,-8.40501764963735,144.264074088329));
#39295=CARTESIAN_POINT('Ctrl Pts',(29.3130596361187,-8.47853772003697,144.18397640341));
#39296=CARTESIAN_POINT('Ctrl Pts',(29.0653952056276,-8.5,144.04005331396));
#39297=CARTESIAN_POINT('Ctrl Pts',(29.0050125628934,-8.5,144.));
#39298=CARTESIAN_POINT('',(31.0500544632573,-8.39129047171135,144.083016665483));
#39299=CARTESIAN_POINT('',(29.0050125628934,-8.5,144.));
#39300=CARTESIAN_POINT('Origin',(30.,-8.45,142.5));
#39301=CARTESIAN_POINT('',(28.8338096210309,-8.4,144.));
#39302=CARTESIAN_POINT('',(31.1048119379707,-8.5,143.921052631579));
#39303=CARTESIAN_POINT('Ctrl Pts',(28.9499455367427,-8.39129047171135,144.083016665483));
#39304=CARTESIAN_POINT('Ctrl Pts',(28.9100201948423,-8.39678689632762,144.057109836194));
#39305=CARTESIAN_POINT('Ctrl Pts',(28.8713894960226,-8.40000000009859,144.029216859175));
#39306=CARTESIAN_POINT('Ctrl Pts',(28.8338096192948,-8.4,143.99999999865));
#39307=CARTESIAN_POINT('Ctrl Pts',(28.9683012121263,-8.4275269811409,144.055344443655));
#39308=CARTESIAN_POINT('Ctrl Pts',(28.9291576919388,-8.43119126421841,144.029764000737));
#39309=CARTESIAN_POINT('Ctrl Pts',(28.8911896803029,-8.43333333339906,144.002388493225));
#39310=CARTESIAN_POINT('Ctrl Pts',(28.854269099658,-8.43333333333333,143.9736842092));
#39311=CARTESIAN_POINT('Ctrl Pts',(28.9866568875098,-8.46376349057045,144.027672221828));
#39312=CARTESIAN_POINT('Ctrl Pts',(28.9482951890352,-8.46559563210921,144.00241816528));
#39313=CARTESIAN_POINT('Ctrl Pts',(28.9109898645832,-8.46666666669953,143.975560127274));
#39314=CARTESIAN_POINT('Ctrl Pts',(28.8747285800213,-8.46666666666667,143.94736841975));
#39315=CARTESIAN_POINT('Ctrl Pts',(29.0050125628934,-8.5,144.));
#39316=CARTESIAN_POINT('Ctrl Pts',(28.9674326861317,-8.5,143.975072329823));
#39317=CARTESIAN_POINT('Ctrl Pts',(28.9307900488635,-8.5,143.948731761324));
#39318=CARTESIAN_POINT('Ctrl Pts',(28.8951880603845,-8.5,143.9210526303));
#39319=CARTESIAN_POINT('Ctrl Pts',(31.166190378969,-8.4,144.));
#39320=CARTESIAN_POINT('Ctrl Pts',(31.1286105027861,-8.4,144.029216860032));
#39321=CARTESIAN_POINT('Ctrl Pts',(31.0899798045429,-8.39678689624297,144.057109836593));
#39322=CARTESIAN_POINT('Ctrl Pts',(31.0500544632573,-8.39129047171134,144.083016665483));
#39323=CARTESIAN_POINT('Ctrl Pts',(31.1457308986363,-8.43333333333333,143.973684210526));
#39324=CARTESIAN_POINT('Ctrl Pts',(31.1088103185267,-8.43333333333333,144.002388494066));
#39325=CARTESIAN_POINT('Ctrl Pts',(31.0708423074584,-8.43119126416198,144.029764001131));
#39326=CARTESIAN_POINT('Ctrl Pts',(31.0316987878737,-8.4275269811409,144.055344443655));
#39327=CARTESIAN_POINT('Ctrl Pts',(31.1252714183035,-8.46666666666667,143.947368421053));
#39328=CARTESIAN_POINT('Ctrl Pts',(31.0890101342673,-8.46666666666667,143.975560128101));
#39329=CARTESIAN_POINT('Ctrl Pts',(31.051704810374,-8.46559563208099,144.002418165669));
#39330=CARTESIAN_POINT('Ctrl Pts',(31.0133431124902,-8.46376349057045,144.027672221828));
#39331=CARTESIAN_POINT('Ctrl Pts',(31.1048119379707,-8.5,143.921052631579));
#39332=CARTESIAN_POINT('Ctrl Pts',(31.0692099500079,-8.5,143.948731762135));
#39333=CARTESIAN_POINT('Ctrl Pts',(31.0325673132895,-8.5,143.975072330207));
#39334=CARTESIAN_POINT('Ctrl Pts',(30.9949874371066,-8.5,144.));
#39335=CARTESIAN_POINT('Ctrl Pts',(-28.9499455367427,-8.39129047171135,
144.083016665483));
#39336=CARTESIAN_POINT('Ctrl Pts',(-28.9583427274828,-8.39013445090614,
144.088465450056));
#39337=CARTESIAN_POINT('Ctrl Pts',(-28.9667729665848,-8.38888022833652,
144.093818270446));
#39338=CARTESIAN_POINT('Ctrl Pts',(-28.9867489659987,-8.38570638741796,
144.10622492921));
#39339=CARTESIAN_POINT('Ctrl Pts',(-28.9982975463468,-8.38372232493232,
144.113195422252));
#39340=CARTESIAN_POINT('Ctrl Pts',(-29.2186401675363,-8.34304381026164,
144.241830661973));
#39341=CARTESIAN_POINT('Ctrl Pts',(-29.4418894510009,-8.26130877991199,
144.30791109331));
#39342=CARTESIAN_POINT('Ctrl Pts',(-29.7387539667785,-8.2037212977524,144.344577795757));
#39343=CARTESIAN_POINT('Ctrl Pts',(-29.7961080426536,-8.19484695032281,
144.349486882414));
#39344=CARTESIAN_POINT('Ctrl Pts',(-29.8806159996987,-8.18658920666495,
144.35392173636));
#39345=CARTESIAN_POINT('Ctrl Pts',(-29.9067939860508,-8.18468265252138,
144.354910990812));
#39346=CARTESIAN_POINT('Ctrl Pts',(-29.945800622645,-8.18289510415931,144.355834150072));
#39347=CARTESIAN_POINT('Ctrl Pts',(-29.9584929581617,-8.18247823187435,
144.356048044385));
#39348=CARTESIAN_POINT('Ctrl Pts',(-30.0243207374447,-8.18117200076953,
144.35671442715));
#39349=CARTESIAN_POINT('Ctrl Pts',(-30.0774739256815,-8.18309698929938,
144.355772172055));
#39350=CARTESIAN_POINT('Ctrl Pts',(-30.1687494835259,-8.19113640094687,
144.351508081756));
#39351=CARTESIAN_POINT('Ctrl Pts',(-30.2069857608087,-8.19595190722736,
144.348893235529));
#39352=CARTESIAN_POINT('Ctrl Pts',(-30.2909203211106,-8.20912670855604,
144.341198190437));
#39353=CARTESIAN_POINT('Ctrl Pts',(-30.3362573241971,-8.21797318024007,
144.335720743413));
#39354=CARTESIAN_POINT('Ctrl Pts',(-30.5020752162372,-8.25459576965121,
144.310394503157));
#39355=CARTESIAN_POINT('Ctrl Pts',(-30.6785437628854,-8.30590308055624,
144.267185314179));
#39356=CARTESIAN_POINT('Ctrl Pts',(-30.8980141119118,-8.36393098595595,
144.173469870658));
#39357=CARTESIAN_POINT('Ctrl Pts',(-31.0000499887335,-8.38440647744572,
144.115463660888));
#39358=CARTESIAN_POINT('Ctrl Pts',(-31.0500544632573,-8.39129047171135,
144.083016665483));
#39359=CARTESIAN_POINT('Ctrl Pts',(-28.9683012121262,-8.4275269811409,144.055344443655));
#39360=CARTESIAN_POINT('Ctrl Pts',(-28.9767493819959,-8.42675549228855,
144.060870258443));
#39361=CARTESIAN_POINT('Ctrl Pts',(-28.9852412077866,-8.42588395004709,
144.066302026648));
#39362=CARTESIAN_POINT('Ctrl Pts',(-29.0053194448347,-8.42359452300562,
144.078903287352));
#39363=CARTESIAN_POINT('Ctrl Pts',(-29.0169530524388,-8.42211782206045,
144.085988617456));
#39364=CARTESIAN_POINT('Ctrl Pts',(-29.2382331610903,-8.39077316976861,
144.216909192503));
#39365=CARTESIAN_POINT('Ctrl Pts',(-29.461356759406,-8.31521293772752,144.286451078415));
#39366=CARTESIAN_POINT('Ctrl Pts',(-29.749585494796,-8.26271593529331,144.325132711801));
#39367=CARTESIAN_POINT('Ctrl Pts',(-29.8048435404432,-8.25457093527495,
144.330334839234));
#39368=CARTESIAN_POINT('Ctrl Pts',(-29.8858928226077,-8.24707060474715,
144.335028465043));
#39369=CARTESIAN_POINT('Ctrl Pts',(-29.9109385934974,-8.24532469917957,
144.336077514689));
#39370=CARTESIAN_POINT('Ctrl Pts',(-29.948225057183,-8.2437038171456,144.337055022579));
#39371=CARTESIAN_POINT('Ctrl Pts',(-29.9603509120841,-8.24332251105181,
144.337281796721));
#39372=CARTESIAN_POINT('Ctrl Pts',(-30.0232223452457,-8.24213657114161,
144.337987844979));
#39373=CARTESIAN_POINT('Ctrl Pts',(-30.073949242754,-8.24388416139077,144.336988263353));
#39374=CARTESIAN_POINT('Ctrl Pts',(-30.1614126316311,-8.25120466871815,
144.332472186435));
#39375=CARTESIAN_POINT('Ctrl Pts',(-30.1981600720549,-8.25559824756781,
144.329702532905));
#39376=CARTESIAN_POINT('Ctrl Pts',(-30.2791744174637,-8.26762595023983,
144.32156645137));
#39377=CARTESIAN_POINT('Ctrl Pts',(-30.323163151243,-8.27572554982767,144.315778125701));
#39378=CARTESIAN_POINT('Ctrl Pts',(-30.4848913781063,-8.30919937251611,
144.289109186482));
#39379=CARTESIAN_POINT('Ctrl Pts',(-30.6594654545242,-8.35615409386017,
144.243787223357));
#39380=CARTESIAN_POINT('Ctrl Pts',(-30.87884927204,-8.40671689444657,144.147356675181));
#39381=CARTESIAN_POINT('Ctrl Pts',(-30.9813729272218,-8.4229080086506,144.088243385872));
#39382=CARTESIAN_POINT('Ctrl Pts',(-31.0316987878737,-8.4275269811409,144.055344443655));
#39383=CARTESIAN_POINT('Ctrl Pts',(-28.9866568875098,-8.46376349057045,
144.027672221828));
#39384=CARTESIAN_POINT('Ctrl Pts',(-28.995167538897,-8.46337895861759,144.033274334817));
#39385=CARTESIAN_POINT('Ctrl Pts',(-29.0036936841412,-8.46288455223563,
144.038786782293));
#39386=CARTESIAN_POINT('Ctrl Pts',(-29.0239172360346,-8.46148854556296,
144.051579899216));
#39387=CARTESIAN_POINT('Ctrl Pts',(-29.035577524684,-8.46050864492644,144.058783731614));
#39388=CARTESIAN_POINT('Ctrl Pts',(-29.257997707443,-8.43848024319824,144.191977951185));
#39389=CARTESIAN_POINT('Ctrl Pts',(-29.4809442721626,-8.3693753244674,144.26497426448));
#39390=CARTESIAN_POINT('Ctrl Pts',(-29.7603830839415,-8.32162051846762,
144.305701005651));
#39391=CARTESIAN_POINT('Ctrl Pts',(-29.8136051874221,-8.31431970227491,
144.311186300222));
#39392=CARTESIAN_POINT('Ctrl Pts',(-29.8911637448792,-8.30751073943584,
144.316145055182));
#39393=CARTESIAN_POINT('Ctrl Pts',(-29.9150906805591,-8.30595688428399,
144.317251044948));
#39394=CARTESIAN_POINT('Ctrl Pts',(-29.950651095842,-8.30448658024128,144.318284380908));
#39395=CARTESIAN_POINT('Ctrl Pts',(-29.9622104521088,-8.3041471128788,144.318523615133));
#39396=CARTESIAN_POINT('Ctrl Pts',(-30.0221330002508,-8.30307648025771,
144.319269178193));
#39397=CARTESIAN_POINT('Ctrl Pts',(-30.0704295912641,-8.3046510696591,144.318213009246));
#39398=CARTESIAN_POINT('Ctrl Pts',(-30.1540743548903,-8.31125999852809,
144.313443903216));
#39399=CARTESIAN_POINT('Ctrl Pts',(-30.1893363532634,-8.31522485466993,
144.310521180289));
#39400=CARTESIAN_POINT('Ctrl Pts',(-30.2674275548308,-8.32612149867921,
144.301941089706));
#39401=CARTESIAN_POINT('Ctrl Pts',(-30.3100712021484,-8.3334556333502,144.295846594569));
#39402=CARTESIAN_POINT('Ctrl Pts',(-30.4677047486626,-8.36383032392711,
144.267824415337));
#39403=CARTESIAN_POINT('Ctrl Pts',(-30.640377126088,-8.40646040610892,144.220399683195));
#39404=CARTESIAN_POINT('Ctrl Pts',(-30.8596850431782,-8.44950872487433,
144.121245390691));
#39405=CARTESIAN_POINT('Ctrl Pts',(-30.9626808008196,-8.46149846879512,
144.061039034221));
#39406=CARTESIAN_POINT('Ctrl Pts',(-31.0133431124902,-8.46376349057045,
144.027672221828));
#39407=CARTESIAN_POINT('Ctrl Pts',(-29.0050125628934,-8.5,144.));
#39408=CARTESIAN_POINT('Ctrl Pts',(-29.0135741934101,-8.5,144.005679143204));
#39409=CARTESIAN_POINT('Ctrl Pts',(-29.0221619253429,-8.4998882739462,144.011270538495));
#39410=CARTESIAN_POINT('Ctrl Pts',(-29.0424877148706,-8.49937668115061,
144.024258257358));
#39411=CARTESIAN_POINT('Ctrl Pts',(-29.054233030776,-8.49890414205457,144.031576926818));
#39412=CARTESIAN_POINT('Ctrl Pts',(-29.277590700997,-8.48620960270521,144.167056481715));
#39413=CARTESIAN_POINT('Ctrl Pts',(-29.5004115805678,-8.42327948228293,
144.243514249585));
#39414=CARTESIAN_POINT('Ctrl Pts',(-29.7712146119589,-8.38061515600853,
144.286255921694));
#39415=CARTESIAN_POINT('Ctrl Pts',(-29.8223406852117,-8.37404368722705,
144.292034257043));
#39416=CARTESIAN_POINT('Ctrl Pts',(-29.8964405677882,-8.36799213751804,
144.297251783865));
#39417=CARTESIAN_POINT('Ctrl Pts',(-29.9192352880058,-8.36659893094219,
144.298417568824));
#39418=CARTESIAN_POINT('Ctrl Pts',(-29.95307553038,-8.36529529322757,144.299505253415));
#39419=CARTESIAN_POINT('Ctrl Pts',(-29.9640684060312,-8.36499139205626,
144.299757367469));
#39420=CARTESIAN_POINT('Ctrl Pts',(-30.0210346080518,-8.36404105062979,
144.300542596022));
#39421=CARTESIAN_POINT('Ctrl Pts',(-30.0669049083367,-8.36543824175049,
144.299429100544));
#39422=CARTESIAN_POINT('Ctrl Pts',(-30.1467375029954,-8.37132826629937,
144.294408007895));
#39423=CARTESIAN_POINT('Ctrl Pts',(-30.1805106645095,-8.37487119501038,
144.291330477666));
#39424=CARTESIAN_POINT('Ctrl Pts',(-30.2556816511839,-8.384620740363,144.282309350639));
#39425=CARTESIAN_POINT('Ctrl Pts',(-30.2969770291942,-8.39120800293779,
144.275903976857));
#39426=CARTESIAN_POINT('Ctrl Pts',(-30.4505209105317,-8.41843392679202,
144.246539098663));
#39427=CARTESIAN_POINT('Ctrl Pts',(-30.6212988177268,-8.45671141941285,
144.197001592374));
#39428=CARTESIAN_POINT('Ctrl Pts',(-30.8405202033064,-8.49229463336495,
144.095132195214));
#39429=CARTESIAN_POINT('Ctrl Pts',(-30.9440037393079,-8.5,144.033818759205));
#39430=CARTESIAN_POINT('Ctrl Pts',(-30.9949874371066,-8.5,144.));
#39431=CARTESIAN_POINT('',(-28.9499455367427,-8.39129047171135,144.083016665483));
#39432=CARTESIAN_POINT('',(-30.9949874371066,-8.5,144.));
#39433=CARTESIAN_POINT('Origin',(-30.,-8.45,142.5));
#39434=CARTESIAN_POINT('',(-31.1661903789691,-8.4,144.));
#39435=CARTESIAN_POINT('',(-28.8951880620293,-8.5,143.921052631579));
#39436=CARTESIAN_POINT('Ctrl Pts',(-31.0500544632573,-8.39129047171135,
144.083016665483));
#39437=CARTESIAN_POINT('Ctrl Pts',(-31.0899798051577,-8.39678689632762,
144.057109836194));
#39438=CARTESIAN_POINT('Ctrl Pts',(-31.1286105039774,-8.40000000009859,
144.029216859175));
#39439=CARTESIAN_POINT('Ctrl Pts',(-31.1661903807052,-8.4,143.99999999865));
#39440=CARTESIAN_POINT('Ctrl Pts',(-31.0316987878738,-8.4275269811409,144.055344443655));
#39441=CARTESIAN_POINT('Ctrl Pts',(-31.0708423080613,-8.43119126421841,
144.029764000737));
#39442=CARTESIAN_POINT('Ctrl Pts',(-31.1088103196971,-8.43333333339906,
144.002388493225));
#39443=CARTESIAN_POINT('Ctrl Pts',(-31.145730900342,-8.43333333333333,143.9736842092));
#39444=CARTESIAN_POINT('Ctrl Pts',(-31.0133431124902,-8.46376349057045,
144.027672221828));
#39445=CARTESIAN_POINT('Ctrl Pts',(-31.0517048109648,-8.46559563210921,
144.00241816528));
#39446=CARTESIAN_POINT('Ctrl Pts',(-31.0890101354168,-8.46666666669953,
143.975560127274));
#39447=CARTESIAN_POINT('Ctrl Pts',(-31.1252714199787,-8.46666666666667,
143.94736841975));
#39448=CARTESIAN_POINT('Ctrl Pts',(-30.9949874371066,-8.5,144.));
#39449=CARTESIAN_POINT('Ctrl Pts',(-31.0325673138683,-8.5,143.975072329823));
#39450=CARTESIAN_POINT('Ctrl Pts',(-31.0692099511365,-8.5,143.948731761324));
#39451=CARTESIAN_POINT('Ctrl Pts',(-31.1048119396155,-8.5,143.9210526303));
#39452=CARTESIAN_POINT('Ctrl Pts',(-28.833809621031,-8.4,144.));
#39453=CARTESIAN_POINT('Ctrl Pts',(-28.8713894972139,-8.4,144.029216860032));
#39454=CARTESIAN_POINT('Ctrl Pts',(-28.9100201954571,-8.39678689624297,
144.057109836593));
#39455=CARTESIAN_POINT('Ctrl Pts',(-28.9499455367427,-8.39129047171135,
144.083016665483));
#39456=CARTESIAN_POINT('Ctrl Pts',(-28.8542691013637,-8.43333333333333,
143.973684210526));
#39457=CARTESIAN_POINT('Ctrl Pts',(-28.8911896814733,-8.43333333333333,
144.002388494066));
#39458=CARTESIAN_POINT('Ctrl Pts',(-28.9291576925416,-8.43119126416198,
144.029764001131));
#39459=CARTESIAN_POINT('Ctrl Pts',(-28.9683012121263,-8.4275269811409,144.055344443655));
#39460=CARTESIAN_POINT('Ctrl Pts',(-28.8747285816965,-8.46666666666667,
143.947368421053));
#39461=CARTESIAN_POINT('Ctrl Pts',(-28.9109898657327,-8.46666666666667,
143.975560128101));
#39462=CARTESIAN_POINT('Ctrl Pts',(-28.948295189626,-8.46559563208099,144.002418165669));
#39463=CARTESIAN_POINT('Ctrl Pts',(-28.9866568875098,-8.46376349057045,
144.027672221828));
#39464=CARTESIAN_POINT('Ctrl Pts',(-28.8951880620293,-8.5,143.921052631579));
#39465=CARTESIAN_POINT('Ctrl Pts',(-28.9307900499921,-8.5,143.948731762135));
#39466=CARTESIAN_POINT('Ctrl Pts',(-28.9674326867105,-8.5,143.975072330207));
#39467=CARTESIAN_POINT('Ctrl Pts',(-29.0050125628934,-8.5,144.));
#39468=CARTESIAN_POINT('Origin',(30.,-8.95,137.5));
#39469=CARTESIAN_POINT('',(29.19613123823,-8.9,135.889473684211));
#39470=CARTESIAN_POINT('',(29.1514718625761,-9.,135.8));
#39471=CARTESIAN_POINT('',(28.2,-8.9,137.5));
#39472=CARTESIAN_POINT('Origin',(30.,-8.9,137.5));
#39473=CARTESIAN_POINT('',(30.80386876177,-8.9,135.889473684211));
#39474=CARTESIAN_POINT('Origin',(30.,-8.9,137.5));
#39475=CARTESIAN_POINT('',(30.80386876177,-8.9,135.889473684211));
#39476=CARTESIAN_POINT('Ctrl Pts',(30.62442393624,-8.99442305443429,135.70570254201));
#39477=CARTESIAN_POINT('Ctrl Pts',(30.6031336007837,-8.99354972599348,135.698345055793));
#39478=CARTESIAN_POINT('Ctrl Pts',(30.5816752394099,-8.9926310079646,135.691382689721));
#39479=CARTESIAN_POINT('Ctrl Pts',(30.4123094665995,-8.98495128128084,135.639444028187));
#39480=CARTESIAN_POINT('Ctrl Pts',(30.1802232821902,-8.97487183787893,135.600774173325));
#39481=CARTESIAN_POINT('Ctrl Pts',(29.8198774693528,-8.97481364719588,135.600649477793));
#39482=CARTESIAN_POINT('Ctrl Pts',(29.5876626138109,-8.9849459908676,135.639432675438));
#39483=CARTESIAN_POINT('Ctrl Pts',(29.418327451187,-8.9926309002887,135.69138245992));
#39484=CARTESIAN_POINT('Ctrl Pts',(29.3968663992163,-8.99354972599348,135.698345055793));
#39485=CARTESIAN_POINT('Ctrl Pts',(29.37557606376,-8.99442305443429,135.70570254201));
#39486=CARTESIAN_POINT('Ctrl Pts',(30.6134852835967,-8.96294870295619,135.737135028007));
#39487=CARTESIAN_POINT('Ctrl Pts',(30.5926585146851,-8.96237089086999,135.729918298573));
#39488=CARTESIAN_POINT('Ctrl Pts',(30.5716540370928,-8.96172231480688,135.723090172466));
#39489=CARTESIAN_POINT('Ctrl Pts',(30.4057627068959,-8.95618694003155,135.671989821309));
#39490=CARTESIAN_POINT('Ctrl Pts',(30.1774809150283,-8.94781763959254,135.633524301555));
#39491=CARTESIAN_POINT('Ctrl Pts',(29.8226191720034,-8.94775803303614,135.63340083736));
#39492=CARTESIAN_POINT('Ctrl Pts',(29.5942099936947,-8.9561825817824,135.671977657887));
#39493=CARTESIAN_POINT('Ctrl Pts',(29.4283485325563,-8.96172203669287,135.723090090889));
#39494=CARTESIAN_POINT('Ctrl Pts',(29.4073415857357,-8.96237102991341,135.729918177652));
#39495=CARTESIAN_POINT('Ctrl Pts',(29.3865147164033,-8.96294870295619,135.737135028007));
#39496=CARTESIAN_POINT('Ctrl Pts',(30.6025466309533,-8.9314743514781,135.768567514004));
#39497=CARTESIAN_POINT('Ctrl Pts',(30.582184785483,-8.93117883512348,135.761502062769));
#39498=CARTESIAN_POINT('Ctrl Pts',(30.5616314866267,-8.93082738428349,135.754786613407));
#39499=CARTESIAN_POINT('Ctrl Pts',(30.3992200288979,-8.92734716856885,135.704598391766));
#39500=CARTESIAN_POINT('Ctrl Pts',(30.1747360509691,-8.92072266060556,135.666303758425));
#39501=CARTESIAN_POINT('Ctrl Pts',(29.8253607851682,-8.92068624425422,135.666171804744));
#39502=CARTESIAN_POINT('Ctrl Pts',(29.6007527034052,-8.9273427984036,135.704587303278));
#39503=CARTESIAN_POINT('Ctrl Pts',(29.4383712024403,-8.93082748462833,135.75478622414));
#39504=CARTESIAN_POINT('Ctrl Pts',(29.4178151140962,-8.93117869608006,135.761502183691));
#39505=CARTESIAN_POINT('Ctrl Pts',(29.3974533690467,-8.9314743514781,135.768567514004));
#39506=CARTESIAN_POINT('Ctrl Pts',(30.59160797831,-8.9,135.8));
#39507=CARTESIAN_POINT('Ctrl Pts',(30.5717096993844,-8.9,135.793075305549));
#39508=CARTESIAN_POINT('Ctrl Pts',(30.5516102843096,-8.89991869112576,135.786494096152));
#39509=CARTESIAN_POINT('Ctrl Pts',(30.3926732691942,-8.89858282731956,135.737144184887));
#39510=CARTESIAN_POINT('Ctrl Pts',(30.1719936838072,-8.89366846231917,135.699053886655));
#39511=CARTESIAN_POINT('Ctrl Pts',(29.8281024878188,-8.89363063009448,135.698923164311));
#39512=CARTESIAN_POINT('Ctrl Pts',(29.607300083289,-8.8985793893184,135.737132285728));
#39513=CARTESIAN_POINT('Ctrl Pts',(29.4483922838095,-8.8999186210325,135.78649385511));
#39514=CARTESIAN_POINT('Ctrl Pts',(29.4282903006156,-8.9,135.793075305549));
#39515=CARTESIAN_POINT('Ctrl Pts',(29.40839202169,-8.9,135.8));
#39516=CARTESIAN_POINT('',(29.40839202169,-8.9,135.8));
#39517=CARTESIAN_POINT('',(29.40839202169,-8.9,135.8));
#39518=CARTESIAN_POINT('',(30.59160797831,-8.9,135.8));
#39519=CARTESIAN_POINT('',(30.62442393624,-8.99442305443429,135.70570254201));
#39520=CARTESIAN_POINT('Ctrl Pts',(30.59160797831,-8.9,135.8));
#39521=CARTESIAN_POINT('Ctrl Pts',(30.5717096993844,-8.9,135.793075305549));
#39522=CARTESIAN_POINT('Ctrl Pts',(30.5516102843096,-8.89991869112576,135.786494096152));
#39523=CARTESIAN_POINT('Ctrl Pts',(30.3926732691942,-8.89858282731956,135.737144184887));
#39524=CARTESIAN_POINT('Ctrl Pts',(30.1719936838072,-8.89366846231917,135.699053886655));
#39525=CARTESIAN_POINT('Ctrl Pts',(29.8281024878188,-8.89363063009448,135.698923164311));
#39526=CARTESIAN_POINT('Ctrl Pts',(29.607300083289,-8.8985793893184,135.737132285728));
#39527=CARTESIAN_POINT('Ctrl Pts',(29.4483922838095,-8.8999186210325,135.78649385511));
#39528=CARTESIAN_POINT('Ctrl Pts',(29.4282903006156,-8.9,135.793075305549));
#39529=CARTESIAN_POINT('Ctrl Pts',(29.40839202169,-8.9,135.8));
#39530=CARTESIAN_POINT('Ctrl Pts',(30.8485281374239,-9.,135.8));
#39531=CARTESIAN_POINT('Ctrl Pts',(30.7759616147067,-9.,135.763779566847));
#39532=CARTESIAN_POINT('Ctrl Pts',(30.7010733797628,-8.99756721057679,135.732190956222));
#39533=CARTESIAN_POINT('Ctrl Pts',(30.62442393624,-8.99442305443429,135.70570254201));
#39534=CARTESIAN_POINT('Ctrl Pts',(30.8336416788726,-8.96666666666667,135.829824561404));
#39535=CARTESIAN_POINT('Ctrl Pts',(30.7623482530451,-8.96666666666667,135.794239574446));
#39536=CARTESIAN_POINT('Ctrl Pts',(30.6887737535176,-8.96504480705119,135.763211800971));
#39537=CARTESIAN_POINT('Ctrl Pts',(30.6134852835966,-8.96294870295619,135.737135028007));
#39538=CARTESIAN_POINT('Ctrl Pts',(30.8187552203213,-8.93333333333333,135.859649122807));
#39539=CARTESIAN_POINT('Ctrl Pts',(30.7487348913836,-8.93333333333333,135.824699582045));
#39540=CARTESIAN_POINT('Ctrl Pts',(30.6764741272724,-8.9325224035256,135.79423264572));
#39541=CARTESIAN_POINT('Ctrl Pts',(30.6025466309533,-8.9314743514781,135.768567514003));
#39542=CARTESIAN_POINT('Ctrl Pts',(30.80386876177,-8.9,135.889473684211));
#39543=CARTESIAN_POINT('Ctrl Pts',(30.7351215297221,-8.9,135.855159589644));
#39544=CARTESIAN_POINT('Ctrl Pts',(30.6641745010272,-8.9,135.825253490469));
#39545=CARTESIAN_POINT('Ctrl Pts',(30.59160797831,-8.9,135.8));
#39546=CARTESIAN_POINT('Ctrl Pts',(30.80386876177,-8.9,135.889473684211));
#39547=CARTESIAN_POINT('Ctrl Pts',(30.7351215297221,-8.9,135.855159589644));
#39548=CARTESIAN_POINT('Ctrl Pts',(30.6641745010272,-8.9,135.825253490469));
#39549=CARTESIAN_POINT('Ctrl Pts',(30.59160797831,-8.9,135.8));
#39550=CARTESIAN_POINT('Ctrl Pts',(29.37557606376,-8.99442305443429,135.70570254201));
#39551=CARTESIAN_POINT('Ctrl Pts',(29.2989266202368,-8.99756721057681,135.732190956222));
#39552=CARTESIAN_POINT('Ctrl Pts',(29.2240383852925,-9.00000000000003,135.763779566847));
#39553=CARTESIAN_POINT('Ctrl Pts',(29.1514718625748,-9.,135.800000000001));
#39554=CARTESIAN_POINT('Ctrl Pts',(29.3865147164033,-8.96294870295619,135.737135028007));
#39555=CARTESIAN_POINT('Ctrl Pts',(29.311226246482,-8.96504480705121,135.763211800971));
#39556=CARTESIAN_POINT('Ctrl Pts',(29.237651746954,-8.96666666666669,135.794239574446));
#39557=CARTESIAN_POINT('Ctrl Pts',(29.1663583211262,-8.96666666666667,135.829824561404));
#39558=CARTESIAN_POINT('Ctrl Pts',(29.3974533690467,-8.9314743514781,135.768567514003));
#39559=CARTESIAN_POINT('Ctrl Pts',(29.3235258727272,-8.9325224035256,135.79423264572));
#39560=CARTESIAN_POINT('Ctrl Pts',(29.2512651086155,-8.93333333333334,135.824699582045));
#39561=CARTESIAN_POINT('Ctrl Pts',(29.1812447796775,-8.93333333333333,135.859649122808));
#39562=CARTESIAN_POINT('Ctrl Pts',(29.40839202169,-8.9,135.8));
#39563=CARTESIAN_POINT('Ctrl Pts',(29.3358254989724,-8.9,135.825253490469));
#39564=CARTESIAN_POINT('Ctrl Pts',(29.2648784702771,-8.9,135.855159589645));
#39565=CARTESIAN_POINT('Ctrl Pts',(29.1961312382288,-8.9,135.889473684211));
#39566=CARTESIAN_POINT('Ctrl Pts',(29.40839202169,-8.9,135.8));
#39567=CARTESIAN_POINT('Ctrl Pts',(29.3358254989724,-8.9,135.825253490469));
#39568=CARTESIAN_POINT('Ctrl Pts',(29.2648784702771,-8.9,135.855159589645));
#39569=CARTESIAN_POINT('Ctrl Pts',(29.1961312382288,-8.9,135.889473684211));
#39570=CARTESIAN_POINT('Origin',(30.,-9.1,137.5));
#39571=CARTESIAN_POINT('',(28.2,-8.5,137.5));
#39572=CARTESIAN_POINT('',(28.2,-9.1,137.5));
#39573=CARTESIAN_POINT('',(31.1048119379707,-8.5,136.078947368421));
#39574=CARTESIAN_POINT('Origin',(30.,-8.5,137.5));
#39575=CARTESIAN_POINT('',(30.9949874371066,-8.5,136.));
#39576=CARTESIAN_POINT('Ctrl Pts',(30.9949874371066,-8.5,136.));
#39577=CARTESIAN_POINT('Ctrl Pts',(31.0325673132895,-8.5,136.024927669793));
#39578=CARTESIAN_POINT('Ctrl Pts',(31.0692099500079,-8.5,136.051268237865));
#39579=CARTESIAN_POINT('Ctrl Pts',(31.1048119379707,-8.5,136.078947368421));
#39580=CARTESIAN_POINT('',(29.0050125628934,-8.5,136.));
#39581=CARTESIAN_POINT('Ctrl Pts',(29.0050125628934,-8.5,136.));
#39582=CARTESIAN_POINT('Ctrl Pts',(29.0135741934101,-8.5,135.994320856796));
#39583=CARTESIAN_POINT('Ctrl Pts',(29.0221618811589,-8.49988793030325,135.988729425776));
#39584=CARTESIAN_POINT('Ctrl Pts',(29.0307750735035,-8.49967127651924,135.983225511632));
#39585=CARTESIAN_POINT('Ctrl Pts',(29.0424872389076,-8.49937667205062,135.975741323395));
#39586=CARTESIAN_POINT('Ctrl Pts',(29.0542337966699,-8.49890119353724,135.968423775377));
#39587=CARTESIAN_POINT('Ctrl Pts',(29.066042131988,-8.49823342511236,135.961258249725));
#39588=CARTESIAN_POINT('Ctrl Pts',(29.2076929772396,-8.49022298509104,135.875301784412));
#39589=CARTESIAN_POINT('Ctrl Pts',(29.3542317404519,-8.45928673703359,135.812713237712));
#39590=CARTESIAN_POINT('Ctrl Pts',(29.5016114139668,-8.42940336594084,135.770275800662));
#39591=CARTESIAN_POINT('Ctrl Pts',(29.5753012507243,-8.41446168039446,135.749057082136));
#39592=CARTESIAN_POINT('Ctrl Pts',(29.6492013150574,-8.39978321408925,135.732876141023));
#39593=CARTESIAN_POINT('Ctrl Pts',(29.7226173155667,-8.38828909107063,135.721416376084));
#39594=CARTESIAN_POINT('Ctrl Pts',(29.7960333160761,-8.37679496805201,135.709956611145));
#39595=CARTESIAN_POINT('Ctrl Pts',(29.8689652527616,-8.36848518831997,135.70321802238));
#39596=CARTESIAN_POINT('Ctrl Pts',(29.9419406646202,-8.36568846720679,135.700861053488));
#39597=CARTESIAN_POINT('Ctrl Pts',(29.9529448634599,-8.36526674056701,135.700505638511));
#39598=CARTESIAN_POINT('Ctrl Pts',(29.9639419471384,-8.36496215917836,135.700256622351));
#39599=CARTESIAN_POINT('Ctrl Pts',(29.9749386829878,-8.36477724654198,135.700102740572));
#39600=CARTESIAN_POINT('Ctrl Pts',(30.0208804218919,-8.3640047256615,135.699459859213));
#39601=CARTESIAN_POINT('Ctrl Pts',(30.0668878418323,-8.36543091711432,135.700630195523));
#39602=CARTESIAN_POINT('Ctrl Pts',(30.1127314030004,-8.36878946104138,135.703461047636));
#39603=CARTESIAN_POINT('Ctrl Pts',(30.3351972997306,-8.3850875292412,135.717198376017));
#39604=CARTESIAN_POINT('Ctrl Pts',(30.5671516888088,-8.45070494455055,135.774596783944));
#39605=CARTESIAN_POINT('Ctrl Pts',(30.7847295199563,-8.4825308206938,135.880027800313));
#39606=CARTESIAN_POINT('Ctrl Pts',(30.8209924918142,-8.48783513338434,135.897599636374));
#39607=CARTESIAN_POINT('Ctrl Pts',(30.8568561148407,-8.49220079220915,135.916505711559));
#39608=CARTESIAN_POINT('Ctrl Pts',(30.8918402206784,-8.49524200886307,135.936457835556));
#39609=CARTESIAN_POINT('Ctrl Pts',(30.9268243265161,-8.49828322551699,135.956409959553));
#39610=CARTESIAN_POINT('Ctrl Pts',(30.9609289151649,-8.5,135.977408132361));
#39611=CARTESIAN_POINT('Ctrl Pts',(30.9949874371066,-8.5,136.));
#39612=CARTESIAN_POINT('',(28.8951880620293,-8.5,136.078947368421));
#39613=CARTESIAN_POINT('Ctrl Pts',(28.8951880620293,-8.5,136.078947368421));
#39614=CARTESIAN_POINT('Ctrl Pts',(28.9307900499921,-8.5,136.051268237865));
#39615=CARTESIAN_POINT('Ctrl Pts',(28.9674326867105,-8.5,136.024927669793));
#39616=CARTESIAN_POINT('Ctrl Pts',(29.0050125628934,-8.5,136.));
#39617=CARTESIAN_POINT('Origin',(30.,-8.5,137.5));
#39618=CARTESIAN_POINT('Ctrl Pts',(28.9499455367427,-8.39129047171135,135.916983334517));
#39619=CARTESIAN_POINT('Ctrl Pts',(28.9583427274828,-8.39013445090615,135.911534549944));
#39620=CARTESIAN_POINT('Ctrl Pts',(28.966773453885,-8.38888037451443,135.90618177344));
#39621=CARTESIAN_POINT('Ctrl Pts',(28.9867484811824,-8.38570649135595,135.893774768811));
#39622=CARTESIAN_POINT('Ctrl Pts',(28.9983029277528,-8.38372333783055,135.886805685331));
#39623=CARTESIAN_POINT('Ctrl Pts',(29.1496188333912,-8.35575770442387,135.798384331373));
#39624=CARTESIAN_POINT('Ctrl Pts',(29.3692004391356,-8.28840055446218,135.713684542132));
#39625=CARTESIAN_POINT('Ctrl Pts',(29.6834526291903,-8.20996395514133,135.657893063385));
#39626=CARTESIAN_POINT('Ctrl Pts',(29.8489117254301,-8.18734058685009,135.646496412784));
#39627=CARTESIAN_POINT('Ctrl Pts',(29.9457556588889,-8.18293453051425,135.644194467675));
#39628=CARTESIAN_POINT('Ctrl Pts',(29.9584452353951,-8.1825139216413,135.643982887837));
#39629=CARTESIAN_POINT('Ctrl Pts',(30.0242680337758,-8.18121722147009,135.643309689515));
#39630=CARTESIAN_POINT('Ctrl Pts',(30.0774858946058,-8.1831094502482,135.644290152174));
#39631=CARTESIAN_POINT('Ctrl Pts',(30.384921872483,-8.21051184206819,135.658444492213));
#39632=CARTESIAN_POINT('Ctrl Pts',(30.6646630172529,-8.30783041470181,135.714213805079));
#39633=CARTESIAN_POINT('Ctrl Pts',(30.9494673877353,-8.37449857575747,135.855365180714));
#39634=CARTESIAN_POINT('Ctrl Pts',(31.0166500895793,-8.38669177291417,135.895307843082));
#39635=CARTESIAN_POINT('Ctrl Pts',(31.0500544632573,-8.39129047171135,135.916983334517));
#39636=CARTESIAN_POINT('Ctrl Pts',(28.9683012121263,-8.4275269811409,135.944655556345));
#39637=CARTESIAN_POINT('Ctrl Pts',(28.9767512906506,-8.42675709109451,135.939129896694));
#39638=CARTESIAN_POINT('Ctrl Pts',(28.9852390066968,-8.4258818399906,135.933697798623));
#39639=CARTESIAN_POINT('Ctrl Pts',(29.0053236866455,-8.42359861525567,135.921096795532));
#39640=CARTESIAN_POINT('Ctrl Pts',(29.0169525628858,-8.42211353739763,135.914012004032));
#39641=CARTESIAN_POINT('Ctrl Pts',(29.1689418008863,-8.40060124330269,135.824022942103));
#39642=CARTESIAN_POINT('Ctrl Pts',(29.3886577290161,-8.34023513638336,135.736269283873));
#39643=CARTESIAN_POINT('Ctrl Pts',(29.6966772130805,-8.26836461579283,135.677498762874));
#39644=CARTESIAN_POINT('Ctrl Pts',(29.8556490282664,-8.24775662303134,135.66541162577));
#39645=CARTESIAN_POINT('Ctrl Pts',(29.948172947781,-8.2437387547405,135.662972846865));
#39646=CARTESIAN_POINT('Ctrl Pts',(29.9603137751968,-8.24336666009415,135.662751533393));
#39647=CARTESIAN_POINT('Ctrl Pts',(30.0231268608963,-8.24214649464565,135.662025763747));
#39648=CARTESIAN_POINT('Ctrl Pts',(30.0740271395939,-8.24394907919365,135.66308988012));
#39649=CARTESIAN_POINT('Ctrl Pts',(30.3681174445248,-8.26856605876248,135.677985805289));
#39650=CARTESIAN_POINT('Ctrl Pts',(30.645085372046,-8.35906005048207,135.737526267015));
#39651=CARTESIAN_POINT('Ctrl Pts',(30.9305485522613,-8.41521263899238,135.882055224341));
#39652=CARTESIAN_POINT('Ctrl Pts',(30.9980718670533,-8.42441502706281,135.922670002529));
#39653=CARTESIAN_POINT('Ctrl Pts',(31.0316987878737,-8.4275269811409,135.944655556345));
#39654=CARTESIAN_POINT('Ctrl Pts',(28.9866568875098,-8.46376349057045,135.972327778172));
#39655=CARTESIAN_POINT('Ctrl Pts',(28.9951656302423,-8.46337735981164,135.966725510047));
#39656=CARTESIAN_POINT('Ctrl Pts',(29.0036963283471,-8.46288646482709,135.961213400593));
#39657=CARTESIAN_POINT('Ctrl Pts',(29.0239120334445,-8.4614845481509,135.948419296674));
#39658=CARTESIAN_POINT('Ctrl Pts',(29.0355841615369,-8.46051099397016,135.941217456675));
#39659=CARTESIAN_POINT('Ctrl Pts',(29.1883700097445,-8.44537944621221,135.849663173682));
#39660=CARTESIAN_POINT('Ctrl Pts',(29.4080438321775,-8.39198403108369,135.758834222622));
#39661=CARTESIAN_POINT('Ctrl Pts',(29.7098767955004,-8.32670408713254,135.697089500421));
#39662=CARTESIAN_POINT('Ctrl Pts',(29.8622279499253,-8.30806915213872,135.684302809393));
#39663=CARTESIAN_POINT('Ctrl Pts',(29.9505275745679,-8.30446251634076,135.681727259321));
#39664=CARTESIAN_POINT('Ctrl Pts',(29.9620734073366,-8.30410942072552,135.681487976795));
#39665=CARTESIAN_POINT('Ctrl Pts',(30.0220215947714,-8.30307545248594,135.680743784981));
#39666=CARTESIAN_POINT('Ctrl Pts',(30.0703465968442,-8.30459128816887,135.681830467577));
#39667=CARTESIAN_POINT('Ctrl Pts',(30.3520017276888,-8.32703331254691,135.69765706294));
#39668=CARTESIAN_POINT('Ctrl Pts',(30.6253883988622,-8.41041154465518,135.760850723329));
#39669=CARTESIAN_POINT('Ctrl Pts',(30.9116385733412,-8.45585238779906,135.908721743118));
#39670=CARTESIAN_POINT('Ctrl Pts',(30.9795071376909,-8.46227674585136,135.950045972915));
#39671=CARTESIAN_POINT('Ctrl Pts',(31.0133431124902,-8.46376349057045,135.972327778172));
#39672=CARTESIAN_POINT('Ctrl Pts',(29.0050125628934,-8.5,136.));
#39673=CARTESIAN_POINT('Ctrl Pts',(29.0135741934101,-8.5,135.994320856796));
#39674=CARTESIAN_POINT('Ctrl Pts',(29.0221618811589,-8.49988793030325,135.988729425776));
#39675=CARTESIAN_POINT('Ctrl Pts',(29.0424872389076,-8.49937667205062,135.975741323395));
#39676=CARTESIAN_POINT('Ctrl Pts',(29.0542337966699,-8.49890119353724,135.968423775377));
#39677=CARTESIAN_POINT('Ctrl Pts',(29.2076929772396,-8.49022298509104,135.875301784412));
#39678=CARTESIAN_POINT('Ctrl Pts',(29.4275011220581,-8.44381861300487,135.781418964363));
#39679=CARTESIAN_POINT('Ctrl Pts',(29.7231013793905,-8.38510474778405,135.71669519991));
#39680=CARTESIAN_POINT('Ctrl Pts',(29.8689652527616,-8.36848518831997,135.70321802238));
#39681=CARTESIAN_POINT('Ctrl Pts',(29.9529448634599,-8.36526674056701,135.700505638511));
#39682=CARTESIAN_POINT('Ctrl Pts',(29.9639419471384,-8.36496215917836,135.700256622351));
#39683=CARTESIAN_POINT('Ctrl Pts',(30.0208804218919,-8.3640047256615,135.699459859213));
#39684=CARTESIAN_POINT('Ctrl Pts',(30.0668878418323,-8.36543091711432,135.700630195523));
#39685=CARTESIAN_POINT('Ctrl Pts',(30.3351972997306,-8.3850875292412,135.717198376017));
#39686=CARTESIAN_POINT('Ctrl Pts',(30.6058107536552,-8.46164118043544,135.784163185266));
#39687=CARTESIAN_POINT('Ctrl Pts',(30.8927197378672,-8.49656645103397,135.935411786744));
#39688=CARTESIAN_POINT('Ctrl Pts',(30.9609289151649,-8.5,135.977408132361));
#39689=CARTESIAN_POINT('Ctrl Pts',(30.9949874371066,-8.5,136.));
#39690=CARTESIAN_POINT('',(28.9499455367427,-8.39129047171135,135.916983334517));
#39691=CARTESIAN_POINT('',(30.9949874371066,-8.5,136.));
#39692=CARTESIAN_POINT('Origin',(30.,-8.45,137.5));
#39693=CARTESIAN_POINT('',(31.1661903789691,-8.4,136.));
#39694=CARTESIAN_POINT('',(28.8951880620293,-8.5,136.078947368421));
#39695=CARTESIAN_POINT('Ctrl Pts',(31.0500544632573,-8.39129047171135,135.916983334517));
#39696=CARTESIAN_POINT('Ctrl Pts',(31.0899798051577,-8.39678689632762,135.942890163806));
#39697=CARTESIAN_POINT('Ctrl Pts',(31.1286105039774,-8.40000000009859,135.970783140825));
#39698=CARTESIAN_POINT('Ctrl Pts',(31.1661903807052,-8.4,136.00000000135));
#39699=CARTESIAN_POINT('Ctrl Pts',(31.0316987878737,-8.4275269811409,135.944655556345));
#39700=CARTESIAN_POINT('Ctrl Pts',(31.0708423080612,-8.43119126421841,135.970235999263));
#39701=CARTESIAN_POINT('Ctrl Pts',(31.1088103196971,-8.43333333339906,135.997611506775));
#39702=CARTESIAN_POINT('Ctrl Pts',(31.145730900342,-8.43333333333333,136.0263157908));
#39703=CARTESIAN_POINT('Ctrl Pts',(31.0133431124902,-8.46376349057045,135.972327778172));
#39704=CARTESIAN_POINT('Ctrl Pts',(31.0517048109648,-8.46559563210921,135.99758183472));
#39705=CARTESIAN_POINT('Ctrl Pts',(31.0890101354168,-8.46666666669953,136.024439872726));
#39706=CARTESIAN_POINT('Ctrl Pts',(31.1252714199787,-8.46666666666667,136.05263158025));
#39707=CARTESIAN_POINT('Ctrl Pts',(30.9949874371066,-8.5,136.));
#39708=CARTESIAN_POINT('Ctrl Pts',(31.0325673138683,-8.5,136.024927670177));
#39709=CARTESIAN_POINT('Ctrl Pts',(31.0692099511365,-8.5,136.051268238676));
#39710=CARTESIAN_POINT('Ctrl Pts',(31.1048119396155,-8.5,136.0789473697));
#39711=CARTESIAN_POINT('Ctrl Pts',(28.833809621031,-8.4,136.));
#39712=CARTESIAN_POINT('Ctrl Pts',(28.8713894972139,-8.4,135.970783139968));
#39713=CARTESIAN_POINT('Ctrl Pts',(28.9100201954571,-8.39678689624297,135.942890163407));
#39714=CARTESIAN_POINT('Ctrl Pts',(28.9499455367427,-8.39129047171135,135.916983334517));
#39715=CARTESIAN_POINT('Ctrl Pts',(28.8542691013637,-8.43333333333333,136.026315789474));
#39716=CARTESIAN_POINT('Ctrl Pts',(28.8911896814733,-8.43333333333333,135.997611505934));
#39717=CARTESIAN_POINT('Ctrl Pts',(28.9291576925416,-8.43119126416198,135.970235998869));
#39718=CARTESIAN_POINT('Ctrl Pts',(28.9683012121263,-8.4275269811409,135.944655556345));
#39719=CARTESIAN_POINT('Ctrl Pts',(28.8747285816965,-8.46666666666667,136.052631578947));
#39720=CARTESIAN_POINT('Ctrl Pts',(28.9109898657327,-8.46666666666667,136.024439871899));
#39721=CARTESIAN_POINT('Ctrl Pts',(28.948295189626,-8.46559563208099,135.997581834331));
#39722=CARTESIAN_POINT('Ctrl Pts',(28.9866568875098,-8.46376349057045,135.972327778172));
#39723=CARTESIAN_POINT('Ctrl Pts',(28.8951880620293,-8.5,136.078947368421));
#39724=CARTESIAN_POINT('Ctrl Pts',(28.9307900499921,-8.5,136.051268237865));
#39725=CARTESIAN_POINT('Ctrl Pts',(28.9674326867105,-8.5,136.024927669793));
#39726=CARTESIAN_POINT('Ctrl Pts',(29.0050125628934,-8.5,136.));
#39727=CARTESIAN_POINT('Origin',(-37.95,8.2,135.8));
#39728=CARTESIAN_POINT('',(-38.,8.90000000000001,135.8));
#39729=CARTESIAN_POINT('',(-37.9,9.,135.8));
#39730=CARTESIAN_POINT('',(-38.,8.90000000000001,135.8));
#39731=CARTESIAN_POINT('',(-37.9,8.2,135.));
#39732=CARTESIAN_POINT('Origin',(-37.9,8.2,135.8));
#39733=CARTESIAN_POINT('',(-38.,8.2,135.1));
#39734=CARTESIAN_POINT('',(-37.9,8.2,135.));
#39735=CARTESIAN_POINT('Origin',(-38.,8.2,135.8));
#39736=CARTESIAN_POINT('Origin',(-37.95,8.95,137.5));
#39737=CARTESIAN_POINT('',(-38.,8.9,144.2));
#39738=CARTESIAN_POINT('',(-37.9,9.,144.2));
#39739=CARTESIAN_POINT('',(-38.,8.9,144.2));
#39740=CARTESIAN_POINT('',(-37.9,9.,137.5));
#39741=CARTESIAN_POINT('',(-38.,8.9,137.5));
#39742=CARTESIAN_POINT('Origin',(-37.95,8.2,144.2));
#39743=CARTESIAN_POINT('',(-38.,8.2,144.9));
#39744=CARTESIAN_POINT('',(-37.9,8.2,145.));
#39745=CARTESIAN_POINT('',(-38.,8.2,144.9));
#39746=CARTESIAN_POINT('Origin',(-37.9,8.2,144.2));
#39747=CARTESIAN_POINT('Origin',(-38.,8.2,144.2));
#39748=CARTESIAN_POINT('Origin',(-37.95,7.75,144.95));
#39749=CARTESIAN_POINT('',(-38.,4.8,144.9));
#39750=CARTESIAN_POINT('',(-37.9,4.8,145.));
#39751=CARTESIAN_POINT('',(-38.,4.8,144.9));
#39752=CARTESIAN_POINT('',(-37.9,7.75,145.));
#39753=CARTESIAN_POINT('',(-38.,7.75,144.9));
#39754=CARTESIAN_POINT('Origin',(-37.95,4.8,144.2));
#39755=CARTESIAN_POINT('',(-38.,4.09999999999999,144.2));
#39756=CARTESIAN_POINT('',(-38.,4.09999999999999,144.2));
#39757=CARTESIAN_POINT('Origin',(-37.9,4.8,144.2));
#39758=CARTESIAN_POINT('Origin',(-38.,4.8,144.2));
#39759=CARTESIAN_POINT('Origin',(-37.95,4.05,142.5));
#39760=CARTESIAN_POINT('',(-38.,4.1,135.8));
#39761=CARTESIAN_POINT('',(-38.,4.1,135.8));
#39762=CARTESIAN_POINT('',(-38.,4.1,142.5));
#39763=CARTESIAN_POINT('Origin',(-37.95,4.8,135.8));
#39764=CARTESIAN_POINT('',(-38.,4.8,135.1));
#39765=CARTESIAN_POINT('',(-37.9,4.8,135.));
#39766=CARTESIAN_POINT('',(-38.,4.8,135.1));
#39767=CARTESIAN_POINT('Origin',(-37.9,4.8,135.8));
#39768=CARTESIAN_POINT('Origin',(-38.,4.8,135.8));
#39769=CARTESIAN_POINT('Origin',(-37.95,5.25,135.05));
#39770=CARTESIAN_POINT('',(-37.9,5.25,135.));
#39771=CARTESIAN_POINT('',(-38.,5.25,135.1));
#39772=CARTESIAN_POINT('Origin',(-38.,4.8,135.8));
#39773=CARTESIAN_POINT('',(-25.8,4.8,135.));
#39774=CARTESIAN_POINT('',(-38.,4.8,135.));
#39775=CARTESIAN_POINT('',(-38.,4.8,135.));
#39776=CARTESIAN_POINT('',(37.9,4.8,135.));
#39777=CARTESIAN_POINT('',(-38.,4.8,135.));
#39778=CARTESIAN_POINT('Origin',(37.9,4.8,135.8));
#39779=CARTESIAN_POINT('Origin',(-38.,4.,135.));
#39780=CARTESIAN_POINT('',(-25.8,8.2,135.));
#39781=CARTESIAN_POINT('',(-38.,8.2,135.));
#39782=CARTESIAN_POINT('',(-25.8,6.5,135.));
#39783=CARTESIAN_POINT('Origin',(-38.,8.2,135.8));
#39784=CARTESIAN_POINT('',(-30.8485281374239,9.,135.8));
#39785=CARTESIAN_POINT('',(-38.,9.,135.8));
#39786=CARTESIAN_POINT('',(-30.62442393624,8.99442305443429,135.70570254201));
#39787=CARTESIAN_POINT('Ctrl Pts',(-30.62442393624,8.99442305443429,135.70570254201));
#39788=CARTESIAN_POINT('Ctrl Pts',(-30.7010733797628,8.99756721057679,135.732190956222));
#39789=CARTESIAN_POINT('Ctrl Pts',(-30.7759616147067,9.,135.763779566847));
#39790=CARTESIAN_POINT('Ctrl Pts',(-30.8485281374239,9.,135.8));
#39791=CARTESIAN_POINT('',(-29.37557606376,8.99442305443429,135.70570254201));
#39792=CARTESIAN_POINT('Ctrl Pts',(-29.37557606376,8.99442305443429,135.70570254201));
#39793=CARTESIAN_POINT('Ctrl Pts',(-29.3968663992163,8.99354972599348,135.698345055793));
#39794=CARTESIAN_POINT('Ctrl Pts',(-29.418327451187,8.9926309002887,135.691382459919));
#39795=CARTESIAN_POINT('Ctrl Pts',(-29.5876626138109,8.9849459908676,135.639432675438));
#39796=CARTESIAN_POINT('Ctrl Pts',(-29.8198774693527,8.97481364719588,135.600649477793));
#39797=CARTESIAN_POINT('Ctrl Pts',(-30.1802232821902,8.97487183787893,135.600774173325));
#39798=CARTESIAN_POINT('Ctrl Pts',(-30.4123094665995,8.98495128128084,135.639444028187));
#39799=CARTESIAN_POINT('Ctrl Pts',(-30.5816752394099,8.99263100796461,135.691382689721));
#39800=CARTESIAN_POINT('Ctrl Pts',(-30.6031336007837,8.99354972599348,135.698345055793));
#39801=CARTESIAN_POINT('Ctrl Pts',(-30.62442393624,8.99442305443429,135.70570254201));
#39802=CARTESIAN_POINT('',(-29.1514718625761,9.,135.8));
#39803=CARTESIAN_POINT('Ctrl Pts',(-29.1514718625749,9.,135.800000000001));
#39804=CARTESIAN_POINT('Ctrl Pts',(-29.2240383852925,9.00000000000003,135.763779566847));
#39805=CARTESIAN_POINT('Ctrl Pts',(-29.2989266202368,8.99756721057681,135.732190956222));
#39806=CARTESIAN_POINT('Ctrl Pts',(-29.37557606376,8.99442305443429,135.70570254201));
#39807=CARTESIAN_POINT('',(29.1514718625761,9.,135.8));
#39808=CARTESIAN_POINT('',(-38.,9.,135.8));
#39809=CARTESIAN_POINT('',(29.37557606376,8.99442305443429,135.70570254201));
#39810=CARTESIAN_POINT('Ctrl Pts',(29.37557606376,8.99442305443429,135.70570254201));
#39811=CARTESIAN_POINT('Ctrl Pts',(29.2989266202372,8.99756721057679,135.732190956222));
#39812=CARTESIAN_POINT('Ctrl Pts',(29.2240383852933,9.,135.763779566847));
#39813=CARTESIAN_POINT('Ctrl Pts',(29.1514718625761,9.,135.8));
#39814=CARTESIAN_POINT('',(30.62442393624,8.99442305443429,135.70570254201));
#39815=CARTESIAN_POINT('Ctrl Pts',(30.62442393624,8.99442305443429,135.70570254201));
#39816=CARTESIAN_POINT('Ctrl Pts',(30.6031336007837,8.99354972599348,135.698345055793));
#39817=CARTESIAN_POINT('Ctrl Pts',(30.581672548813,8.99263090028869,135.69138245992));
#39818=CARTESIAN_POINT('Ctrl Pts',(30.4123373861891,8.9849459908676,135.639432675438));
#39819=CARTESIAN_POINT('Ctrl Pts',(30.1801225306472,8.97481364719588,135.600649477793));
#39820=CARTESIAN_POINT('Ctrl Pts',(29.8197767178098,8.97487183787893,135.600774173325));
#39821=CARTESIAN_POINT('Ctrl Pts',(29.5876905334005,8.98495128128084,135.639444028187));
#39822=CARTESIAN_POINT('Ctrl Pts',(29.4183247605901,8.99263100796461,135.691382689721));
#39823=CARTESIAN_POINT('Ctrl Pts',(29.3968663992163,8.99354972599348,135.698345055793));
#39824=CARTESIAN_POINT('Ctrl Pts',(29.37557606376,8.99442305443429,135.70570254201));
#39825=CARTESIAN_POINT('',(30.8485281374239,9.,135.8));
#39826=CARTESIAN_POINT('Ctrl Pts',(30.8485281374252,9.,135.800000000001));
#39827=CARTESIAN_POINT('Ctrl Pts',(30.7759616147075,9.00000000000003,135.763779566847));
#39828=CARTESIAN_POINT('Ctrl Pts',(30.7010733797633,8.99756721057681,135.732190956222));
#39829=CARTESIAN_POINT('Ctrl Pts',(30.62442393624,8.99442305443429,135.70570254201));
#39830=CARTESIAN_POINT('',(37.9,9.,135.8));
#39831=CARTESIAN_POINT('',(-38.,9.,135.8));
#39832=CARTESIAN_POINT('',(37.9,8.2,135.));
#39833=CARTESIAN_POINT('Origin',(37.9,8.2,135.8));
#39834=CARTESIAN_POINT('',(-38.,8.2,135.));
#39835=CARTESIAN_POINT('',(-38.,8.2,135.));
#39836=CARTESIAN_POINT('Origin',(-38.,6.5,140.));
#39837=CARTESIAN_POINT('',(-38.,8.5,144.));
#39838=CARTESIAN_POINT('',(-38.,8.5,136.));
#39839=CARTESIAN_POINT('',(-38.,8.5,142.2));
#39840=CARTESIAN_POINT('',(-38.,8.,144.5));
#39841=CARTESIAN_POINT('Origin',(-38.,8.,144.));
#39842=CARTESIAN_POINT('',(-38.,5.,144.5));
#39843=CARTESIAN_POINT('',(-38.,5.55,144.5));
#39844=CARTESIAN_POINT('',(-38.,4.5,144.));
#39845=CARTESIAN_POINT('Origin',(-38.,5.,144.));
#39846=CARTESIAN_POINT('',(-38.,4.50000000000002,136.));
#39847=CARTESIAN_POINT('',(-38.,4.5,137.8));
#39848=CARTESIAN_POINT('',(-38.,5.,135.5));
#39849=CARTESIAN_POINT('Origin',(-38.,5.,136.));
#39850=CARTESIAN_POINT('',(-38.,8.,135.5));
#39851=CARTESIAN_POINT('',(-38.,7.45,135.5));
#39852=CARTESIAN_POINT('Origin',(-38.,8.,136.));
#39853=CARTESIAN_POINT('Origin',(37.95,8.2,135.8));
#39854=CARTESIAN_POINT('',(38.,8.2,135.1));
#39855=CARTESIAN_POINT('',(38.,8.2,135.1));
#39856=CARTESIAN_POINT('',(38.,8.90000000000001,135.8));
#39857=CARTESIAN_POINT('',(37.9,9.,135.8));
#39858=CARTESIAN_POINT('Origin',(38.,8.2,135.8));
#39859=CARTESIAN_POINT('Origin',(37.95,5.25,135.05));
#39860=CARTESIAN_POINT('',(38.,4.8,135.1));
#39861=CARTESIAN_POINT('',(38.,5.25,135.1));
#39862=CARTESIAN_POINT('',(38.,4.8,135.1));
#39863=CARTESIAN_POINT('',(37.9,5.25,135.));
#39864=CARTESIAN_POINT('Origin',(37.95,4.8,135.8));
#39865=CARTESIAN_POINT('',(38.,4.09999999999999,135.8));
#39866=CARTESIAN_POINT('',(38.,4.09999999999999,135.8));
#39867=CARTESIAN_POINT('Origin',(38.,4.8,135.8));
#39868=CARTESIAN_POINT('Origin',(37.95,4.05,142.5));
#39869=CARTESIAN_POINT('',(38.,4.1,144.2));
#39870=CARTESIAN_POINT('',(38.,4.1,142.5));
#39871=CARTESIAN_POINT('',(38.,4.1,144.2));
#39872=CARTESIAN_POINT('Origin',(37.95,4.8,144.2));
#39873=CARTESIAN_POINT('',(38.,4.8,144.9));
#39874=CARTESIAN_POINT('',(37.9,4.8,145.));
#39875=CARTESIAN_POINT('',(38.,4.8,144.9));
#39876=CARTESIAN_POINT('Origin',(37.9,4.8,144.2));
#39877=CARTESIAN_POINT('Origin',(38.,4.8,144.2));
#39878=CARTESIAN_POINT('Origin',(37.95,7.75,144.95));
#39879=CARTESIAN_POINT('',(38.,8.2,144.9));
#39880=CARTESIAN_POINT('',(38.,7.75,144.9));
#39881=CARTESIAN_POINT('',(37.9,8.2,145.));
#39882=CARTESIAN_POINT('',(38.,8.2,144.9));
#39883=CARTESIAN_POINT('',(37.9,7.75,145.));
#39884=CARTESIAN_POINT('Origin',(37.95,8.2,144.2));
#39885=CARTESIAN_POINT('',(38.,8.90000000000001,144.2));
#39886=CARTESIAN_POINT('',(37.9,9.,144.2));
#39887=CARTESIAN_POINT('',(38.,8.90000000000001,144.2));
#39888=CARTESIAN_POINT('Origin',(37.9,8.2,144.2));
#39889=CARTESIAN_POINT('Origin',(38.,8.2,144.2));
#39890=CARTESIAN_POINT('Origin',(37.95,8.95,137.5));
#39891=CARTESIAN_POINT('',(38.,8.9,137.5));
#39892=CARTESIAN_POINT('',(37.9,9.,137.5));
#39893=CARTESIAN_POINT('Origin',(-38.,9.,145.));
#39894=CARTESIAN_POINT('',(-38.,4.8,145.));
#39895=CARTESIAN_POINT('',(-38.,8.2,145.));
#39896=CARTESIAN_POINT('Origin',(-38.,8.2,144.2));
#39897=CARTESIAN_POINT('',(30.8485281374239,9.,144.2));
#39898=CARTESIAN_POINT('',(-38.,9.,144.2));
#39899=CARTESIAN_POINT('',(30.62442393624,8.99442305443429,144.29429745799));
#39900=CARTESIAN_POINT('Ctrl Pts',(30.62442393624,8.99442305443429,144.29429745799));
#39901=CARTESIAN_POINT('Ctrl Pts',(30.7010733797628,8.99756721057679,144.267809043778));
#39902=CARTESIAN_POINT('Ctrl Pts',(30.7759616147067,9.,144.236220433153));
#39903=CARTESIAN_POINT('Ctrl Pts',(30.8485281374239,9.,144.2));
#39904=CARTESIAN_POINT('',(29.37557606376,8.99442305443429,144.29429745799));
#39905=CARTESIAN_POINT('Ctrl Pts',(29.37557606376,8.99442305443429,144.29429745799));
#39906=CARTESIAN_POINT('Ctrl Pts',(29.3968663992163,8.99354972599348,144.301654944207));
#39907=CARTESIAN_POINT('Ctrl Pts',(29.418327449872,8.99263089654327,144.308617544038));
#39908=CARTESIAN_POINT('Ctrl Pts',(29.587662650504,8.98494611755363,144.360567193318));
#39909=CARTESIAN_POINT('Ctrl Pts',(29.8198775424307,8.97481395248941,144.39935020957));
#39910=CARTESIAN_POINT('Ctrl Pts',(30.180223294947,8.97487213269987,144.399225510548));
#39911=CARTESIAN_POINT('Ctrl Pts',(30.4123094590021,8.98495141076798,144.360555832908));
#39912=CARTESIAN_POINT('Ctrl Pts',(30.5816752399674,8.99263100404222,144.308617314527));
#39913=CARTESIAN_POINT('Ctrl Pts',(30.6031336007836,8.99354972599347,144.301654944207));
#39914=CARTESIAN_POINT('Ctrl Pts',(30.62442393624,8.99442305443429,144.29429745799));
#39915=CARTESIAN_POINT('',(29.1514718625761,9.,144.2));
#39916=CARTESIAN_POINT('Ctrl Pts',(29.1514718625749,9.,144.199999999999));
#39917=CARTESIAN_POINT('Ctrl Pts',(29.2240383852925,9.00000000000003,144.236220433153));
#39918=CARTESIAN_POINT('Ctrl Pts',(29.2989266202368,8.99756721057681,144.267809043778));
#39919=CARTESIAN_POINT('Ctrl Pts',(29.37557606376,8.99442305443429,144.29429745799));
#39920=CARTESIAN_POINT('',(-29.1514718625761,9.,144.2));
#39921=CARTESIAN_POINT('',(-38.,9.,144.2));
#39922=CARTESIAN_POINT('',(-29.37557606376,8.99442305443429,144.29429745799));
#39923=CARTESIAN_POINT('Ctrl Pts',(-29.37557606376,8.99442305443429,144.29429745799));
#39924=CARTESIAN_POINT('Ctrl Pts',(-29.2989266202372,8.99756721057679,144.267809043778));
#39925=CARTESIAN_POINT('Ctrl Pts',(-29.2240383852933,9.,144.236220433153));
#39926=CARTESIAN_POINT('Ctrl Pts',(-29.1514718625761,9.,144.2));
#39927=CARTESIAN_POINT('',(-30.62442393624,8.99442305443429,144.29429745799));
#39928=CARTESIAN_POINT('Ctrl Pts',(-30.62442393624,8.99442305443429,144.29429745799));
#39929=CARTESIAN_POINT('Ctrl Pts',(-30.6031336007837,8.99354972599348,144.301654944207));
#39930=CARTESIAN_POINT('Ctrl Pts',(-30.5816983343123,8.99261835182926,144.308632644433));
#39931=CARTESIAN_POINT('Ctrl Pts',(-30.4860772057434,8.98837707594693,144.337802199667));
#39932=CARTESIAN_POINT('Ctrl Pts',(-30.3737546351539,8.98306099714656,144.364880756376));
#39933=CARTESIAN_POINT('Ctrl Pts',(-30.1448589551985,8.97549033242365,144.39734513884));
#39934=CARTESIAN_POINT('Ctrl Pts',(-29.8570704543082,8.97294630891696,144.405692333025));
#39935=CARTESIAN_POINT('Ctrl Pts',(-29.5879618888624,8.98495073555583,144.36060019061));
#39936=CARTESIAN_POINT('Ctrl Pts',(-29.4183017778428,8.99262938553082,144.308615224025));
#39937=CARTESIAN_POINT('Ctrl Pts',(-29.3968663992163,8.99354972599348,144.301654944207));
#39938=CARTESIAN_POINT('Ctrl Pts',(-29.37557606376,8.99442305443429,144.29429745799));
#39939=CARTESIAN_POINT('',(-30.8485281374239,9.,144.2));
#39940=CARTESIAN_POINT('Ctrl Pts',(-30.8485281374251,9.,144.199999999999));
#39941=CARTESIAN_POINT('Ctrl Pts',(-30.7759616147075,9.00000000000003,144.236220433153));
#39942=CARTESIAN_POINT('Ctrl Pts',(-30.7010733797632,8.99756721057681,144.267809043778));
#39943=CARTESIAN_POINT('Ctrl Pts',(-30.62442393624,8.99442305443429,144.29429745799));
#39944=CARTESIAN_POINT('',(-38.,9.,144.2));
#39945=CARTESIAN_POINT('Origin',(-38.,9.,135.));
#39946=CARTESIAN_POINT('Origin',(-30.,9.,142.5));
#39947=CARTESIAN_POINT('Origin',(30.,9.,142.5));
#39948=CARTESIAN_POINT('Origin',(30.,9.,137.5));
#39949=CARTESIAN_POINT('Origin',(-30.,9.,137.5));
#39950=CARTESIAN_POINT('Origin',(38.,6.5,140.));
#39951=CARTESIAN_POINT('',(38.,8.5,136.));
#39952=CARTESIAN_POINT('',(38.,8.5,144.));
#39953=CARTESIAN_POINT('',(38.,8.5,142.2));
#39954=CARTESIAN_POINT('',(38.,8.,135.5));
#39955=CARTESIAN_POINT('Origin',(38.,8.,136.));
#39956=CARTESIAN_POINT('',(38.,5.,135.5));
#39957=CARTESIAN_POINT('',(38.,7.45,135.5));
#39958=CARTESIAN_POINT('',(38.,4.50000000000002,136.));
#39959=CARTESIAN_POINT('Origin',(38.,5.,136.));
#39960=CARTESIAN_POINT('',(38.,4.5,144.));
#39961=CARTESIAN_POINT('',(38.,4.5,137.8));
#39962=CARTESIAN_POINT('',(38.,5.,144.5));
#39963=CARTESIAN_POINT('Origin',(38.,5.,144.));
#39964=CARTESIAN_POINT('',(38.,8.,144.5));
#39965=CARTESIAN_POINT('',(38.,5.55,144.5));
#39966=CARTESIAN_POINT('Origin',(38.,8.,144.));
#39967=CARTESIAN_POINT('Ctrl Pts',(30.62442393624,8.99442305443429,144.29429745799));
#39968=CARTESIAN_POINT('Ctrl Pts',(30.6031336007836,8.99354972599347,144.301654944207));
#39969=CARTESIAN_POINT('Ctrl Pts',(30.5816752399674,8.99263100404222,144.308617314527));
#39970=CARTESIAN_POINT('Ctrl Pts',(30.4123094590021,8.98495141076798,144.360555832908));
#39971=CARTESIAN_POINT('Ctrl Pts',(30.180223294947,8.97487213269987,144.399225510548));
#39972=CARTESIAN_POINT('Ctrl Pts',(29.8198775424307,8.97481395248941,144.39935020957));
#39973=CARTESIAN_POINT('Ctrl Pts',(29.587662650504,8.98494611755363,144.360567193318));
#39974=CARTESIAN_POINT('Ctrl Pts',(29.418327449872,8.99263089654327,144.308617544038));
#39975=CARTESIAN_POINT('Ctrl Pts',(29.3968663992163,8.99354972599348,144.301654944207));
#39976=CARTESIAN_POINT('Ctrl Pts',(29.37557606376,8.99442305443429,144.29429745799));
#39977=CARTESIAN_POINT('Ctrl Pts',(30.6134852835967,8.96294870295619,144.262864971993));
#39978=CARTESIAN_POINT('Ctrl Pts',(30.592658514685,8.96237089086999,144.270081701427));
#39979=CARTESIAN_POINT('Ctrl Pts',(30.5716540376503,8.96172231088449,144.276909831782));
#39980=CARTESIAN_POINT('Ctrl Pts',(30.4057626992984,8.95618706951869,144.328010039787));
#39981=CARTESIAN_POINT('Ctrl Pts',(30.177480927785,8.94781793441349,144.366475382318));
#39982=CARTESIAN_POINT('Ctrl Pts',(29.8226192450814,8.94775833832967,144.366598850003));
#39983=CARTESIAN_POINT('Ctrl Pts',(29.5942100303878,8.95618270846843,144.328022210868));
#39984=CARTESIAN_POINT('Ctrl Pts',(29.4283485312412,8.96172203294744,144.276909913069));
#39985=CARTESIAN_POINT('Ctrl Pts',(29.4073415857357,8.96237102991341,144.270081822348));
#39986=CARTESIAN_POINT('Ctrl Pts',(29.3865147164033,8.96294870295619,144.262864971993));
#39987=CARTESIAN_POINT('Ctrl Pts',(30.6025466309533,8.9314743514781,144.231432485997));
#39988=CARTESIAN_POINT('Ctrl Pts',(30.5821847854831,8.93117883512348,144.238497937231));
#39989=CARTESIAN_POINT('Ctrl Pts',(30.5616314871845,8.93082738132286,144.245213391643));
#39990=CARTESIAN_POINT('Ctrl Pts',(30.3992200209108,8.92734726636692,144.295401442766));
#39991=CARTESIAN_POINT('Ctrl Pts',(30.1747360622273,8.92072288323236,144.333695864957));
#39992=CARTESIAN_POINT('Ctrl Pts',(29.8253608556981,8.92068647619822,144.333827818585));
#39993=CARTESIAN_POINT('Ctrl Pts',(29.6007527390699,8.92734289454247,144.295412539047));
#39994=CARTESIAN_POINT('Ctrl Pts',(29.4383712011633,8.93082748179126,144.245213780592));
#39995=CARTESIAN_POINT('Ctrl Pts',(29.4178151140962,8.93117869608006,144.238497816309));
#39996=CARTESIAN_POINT('Ctrl Pts',(29.3974533690467,8.9314743514781,144.231432485996));
#39997=CARTESIAN_POINT('Ctrl Pts',(30.59160797831,8.9,144.2));
#39998=CARTESIAN_POINT('Ctrl Pts',(30.5717096993845,8.9,144.206924694451));
#39999=CARTESIAN_POINT('Ctrl Pts',(30.5516102848674,8.89991868816513,144.213505908897));
#40000=CARTESIAN_POINT('Ctrl Pts',(30.3926732612071,8.89858292511763,144.262855649644));
#40001=CARTESIAN_POINT('Ctrl Pts',(30.1719936950654,8.89366868494597,144.300945736727));
#40002=CARTESIAN_POINT('Ctrl Pts',(29.8281025583487,8.89363086203848,144.301076459018));
#40003=CARTESIAN_POINT('Ctrl Pts',(29.6073001189537,8.89857948545727,144.262867556597));
#40004=CARTESIAN_POINT('Ctrl Pts',(29.4483922825326,8.89991861819543,144.213506149622));
#40005=CARTESIAN_POINT('Ctrl Pts',(29.4282903006156,8.9,144.206924694451));
#40006=CARTESIAN_POINT('Ctrl Pts',(29.40839202169,8.9,144.2));
#40007=CARTESIAN_POINT('',(29.40839202169,8.9,144.2));
#40008=CARTESIAN_POINT('',(29.40839202169,8.9,144.2));
#40009=CARTESIAN_POINT('',(30.59160797831,8.9,144.2));
#40010=CARTESIAN_POINT('',(30.62442393624,8.99442305443429,144.29429745799));
#40011=CARTESIAN_POINT('Ctrl Pts',(30.59160797831,8.9,144.2));
#40012=CARTESIAN_POINT('Ctrl Pts',(30.5717096993845,8.9,144.206924694451));
#40013=CARTESIAN_POINT('Ctrl Pts',(30.5516102848674,8.89991868816513,144.213505908897));
#40014=CARTESIAN_POINT('Ctrl Pts',(30.3926732612071,8.89858292511763,144.262855649644));
#40015=CARTESIAN_POINT('Ctrl Pts',(30.1719936950654,8.89366868494597,144.300945736727));
#40016=CARTESIAN_POINT('Ctrl Pts',(29.8281025583487,8.89363086203848,144.301076459018));
#40017=CARTESIAN_POINT('Ctrl Pts',(29.6073001189537,8.89857948545727,144.262867556597));
#40018=CARTESIAN_POINT('Ctrl Pts',(29.4483922825326,8.89991861819543,144.213506149622));
#40019=CARTESIAN_POINT('Ctrl Pts',(29.4282903006156,8.9,144.206924694451));
#40020=CARTESIAN_POINT('Ctrl Pts',(29.40839202169,8.9,144.2));
#40021=CARTESIAN_POINT('Origin',(30.,8.95,142.5));
#40022=CARTESIAN_POINT('',(29.19613123823,8.9,144.110526315789));
#40023=CARTESIAN_POINT('',(29.1514718625761,9.,144.2));
#40024=CARTESIAN_POINT('',(28.2,8.9,142.5));
#40025=CARTESIAN_POINT('Origin',(30.,8.9,142.5));
#40026=CARTESIAN_POINT('',(30.80386876177,8.9,144.110526315789));
#40027=CARTESIAN_POINT('Origin',(30.,8.9,142.5));
#40028=CARTESIAN_POINT('',(30.80386876177,8.9,144.110526315789));
#40029=CARTESIAN_POINT('Ctrl Pts',(29.37557606376,8.99442305443429,144.29429745799));
#40030=CARTESIAN_POINT('Ctrl Pts',(29.2989266202368,8.99756721057681,144.267809043778));
#40031=CARTESIAN_POINT('Ctrl Pts',(29.2240383852925,9.00000000000003,144.236220433153));
#40032=CARTESIAN_POINT('Ctrl Pts',(29.1514718625749,9.,144.199999999999));
#40033=CARTESIAN_POINT('Ctrl Pts',(29.3865147164033,8.96294870295619,144.262864971993));
#40034=CARTESIAN_POINT('Ctrl Pts',(29.311226246482,8.96504480705121,144.236788199029));
#40035=CARTESIAN_POINT('Ctrl Pts',(29.237651746954,8.96666666666668,144.205760425554));
#40036=CARTESIAN_POINT('Ctrl Pts',(29.1663583211262,8.96666666666667,144.170175438596));
#40037=CARTESIAN_POINT('Ctrl Pts',(29.3974533690467,8.9314743514781,144.231432485997));
#40038=CARTESIAN_POINT('Ctrl Pts',(29.3235258727272,8.9325224035256,144.20576735428));
#40039=CARTESIAN_POINT('Ctrl Pts',(29.2512651086156,8.93333333333334,144.175300417955));
#40040=CARTESIAN_POINT('Ctrl Pts',(29.1812447796775,8.93333333333333,144.140350877192));
#40041=CARTESIAN_POINT('Ctrl Pts',(29.40839202169,8.9,144.2));
#40042=CARTESIAN_POINT('Ctrl Pts',(29.3358254989724,8.9,144.174746509531));
#40043=CARTESIAN_POINT('Ctrl Pts',(29.2648784702771,8.9,144.144840410355));
#40044=CARTESIAN_POINT('Ctrl Pts',(29.1961312382288,8.9,144.110526315789));
#40045=CARTESIAN_POINT('Ctrl Pts',(29.40839202169,8.9,144.2));
#40046=CARTESIAN_POINT('Ctrl Pts',(29.3358254989724,8.9,144.174746509531));
#40047=CARTESIAN_POINT('Ctrl Pts',(29.2648784702771,8.9,144.144840410355));
#40048=CARTESIAN_POINT('Ctrl Pts',(29.1961312382288,8.9,144.110526315789));
#40049=CARTESIAN_POINT('Ctrl Pts',(30.8485281374239,9.,144.2));
#40050=CARTESIAN_POINT('Ctrl Pts',(30.7759616147067,9.,144.236220433153));
#40051=CARTESIAN_POINT('Ctrl Pts',(30.7010733797628,8.99756721057679,144.267809043778));
#40052=CARTESIAN_POINT('Ctrl Pts',(30.62442393624,8.99442305443429,144.29429745799));
#40053=CARTESIAN_POINT('Ctrl Pts',(30.8336416788726,8.96666666666667,144.170175438596));
#40054=CARTESIAN_POINT('Ctrl Pts',(30.7623482530451,8.96666666666667,144.205760425554));
#40055=CARTESIAN_POINT('Ctrl Pts',(30.6887737535176,8.96504480705119,144.236788199029));
#40056=CARTESIAN_POINT('Ctrl Pts',(30.6134852835966,8.96294870295619,144.262864971993));
#40057=CARTESIAN_POINT('Ctrl Pts',(30.8187552203213,8.93333333333333,144.140350877193));
#40058=CARTESIAN_POINT('Ctrl Pts',(30.7487348913836,8.93333333333333,144.175300417955));
#40059=CARTESIAN_POINT('Ctrl Pts',(30.6764741272724,8.9325224035256,144.20576735428));
#40060=CARTESIAN_POINT('Ctrl Pts',(30.6025466309533,8.9314743514781,144.231432485997));
#40061=CARTESIAN_POINT('Ctrl Pts',(30.80386876177,8.9,144.110526315789));
#40062=CARTESIAN_POINT('Ctrl Pts',(30.7351215297221,8.9,144.144840410356));
#40063=CARTESIAN_POINT('Ctrl Pts',(30.6641745010272,8.9,144.174746509531));
#40064=CARTESIAN_POINT('Ctrl Pts',(30.59160797831,8.9,144.2));
#40065=CARTESIAN_POINT('Ctrl Pts',(30.80386876177,8.9,144.110526315789));
#40066=CARTESIAN_POINT('Ctrl Pts',(30.7351215297221,8.9,144.144840410356));
#40067=CARTESIAN_POINT('Ctrl Pts',(30.6641745010272,8.9,144.174746509531));
#40068=CARTESIAN_POINT('Ctrl Pts',(30.59160797831,8.9,144.2));
#40069=CARTESIAN_POINT('Origin',(30.,9.1,142.5));
#40070=CARTESIAN_POINT('',(28.2,8.5,142.5));
#40071=CARTESIAN_POINT('',(28.2,9.1,142.5));
#40072=CARTESIAN_POINT('',(31.1048119379707,8.5,143.921052631579));
#40073=CARTESIAN_POINT('Origin',(30.,8.5,142.5));
#40074=CARTESIAN_POINT('',(30.9949874371066,8.5,144.));
#40075=CARTESIAN_POINT('Ctrl Pts',(30.9949874371066,8.5,144.));
#40076=CARTESIAN_POINT('Ctrl Pts',(31.0325673132895,8.5,143.975072330207));
#40077=CARTESIAN_POINT('Ctrl Pts',(31.0692099500079,8.5,143.948731762135));
#40078=CARTESIAN_POINT('Ctrl Pts',(31.1048119379707,8.5,143.921052631579));
#40079=CARTESIAN_POINT('',(29.0050125628934,8.5,144.));
#40080=CARTESIAN_POINT('Ctrl Pts',(29.0050125628934,8.5,144.));
#40081=CARTESIAN_POINT('Ctrl Pts',(29.0135741934101,8.5,144.005679143204));
#40082=CARTESIAN_POINT('Ctrl Pts',(29.0221619009622,8.499887926188,144.011270571938));
#40083=CARTESIAN_POINT('Ctrl Pts',(29.0307751172111,8.49967126826958,144.016774482844));
#40084=CARTESIAN_POINT('Ctrl Pts',(29.0424873151203,8.49937665817902,144.024258666676));
#40085=CARTESIAN_POINT('Ctrl Pts',(29.0542337840516,8.49890119138507,144.031576228849));
#40086=CARTESIAN_POINT('Ctrl Pts',(29.0660423164974,8.49823339234552,144.038741725773));
#40087=CARTESIAN_POINT('Ctrl Pts',(29.2076955264615,8.4902225850757,144.12469784648));
#40088=CARTESIAN_POINT('Ctrl Pts',(29.3542371018997,8.45928538094257,144.187286288274));
#40089=CARTESIAN_POINT('Ctrl Pts',(29.5016183779968,8.4294021201831,144.229723268464));
#40090=CARTESIAN_POINT('Ctrl Pts',(29.5753090160454,8.41446048980336,144.250941758559));
#40091=CARTESIAN_POINT('Ctrl Pts',(29.6492095792586,8.39978234526704,144.267122383253));
#40092=CARTESIAN_POINT('Ctrl Pts',(29.7226256562424,8.38828793821598,144.278582306918));
#40093=CARTESIAN_POINT('Ctrl Pts',(29.7960417332263,8.37679353116492,144.290042230583));
#40094=CARTESIAN_POINT('Ctrl Pts',(29.8689733239806,8.36848286159913,144.296781453219));
#40095=CARTESIAN_POINT('Ctrl Pts',(29.94195145693,8.36568839991374,144.299136383465));
#40096=CARTESIAN_POINT('Ctrl Pts',(29.9529560660921,8.3652670139804,144.299491491028));
#40097=CARTESIAN_POINT('Ctrl Pts',(29.9639511678485,8.36496071281008,144.29974204166));
#40098=CARTESIAN_POINT('Ctrl Pts',(29.9749502142532,8.36477781319046,144.2998941289));
#40099=CARTESIAN_POINT('Ctrl Pts',(29.9964912242973,8.36441961463412,144.300191983155));
#40100=CARTESIAN_POINT('Ctrl Pts',(30.0180354039898,8.36453081890395,144.30009870167));
#40101=CARTESIAN_POINT('Ctrl Pts',(30.0395683094927,8.36510330880466,144.299626292527));
#40102=CARTESIAN_POINT('Ctrl Pts',(30.0639695071918,8.36575205726298,144.299090956091));
#40103=CARTESIAN_POINT('Ctrl Pts',(30.0884019395258,8.36701354869722,144.298029111375));
#40104=CARTESIAN_POINT('Ctrl Pts',(30.1127651425163,8.36879615201152,144.296524636117));
#40105=CARTESIAN_POINT('Ctrl Pts',(30.3353233320769,8.38508025745082,144.282781234235));
#40106=CARTESIAN_POINT('Ctrl Pts',(30.5671595347865,8.45070605233951,144.225400079081));
#40107=CARTESIAN_POINT('Ctrl Pts',(30.7847332434266,8.4825312867794,144.119970740243));
#40108=CARTESIAN_POINT('Ctrl Pts',(30.8209955281999,8.48783549251939,144.10239918377));
#40109=CARTESIAN_POINT('Ctrl Pts',(30.8568616325825,8.49220079380246,144.083492955528));
#40110=CARTESIAN_POINT('Ctrl Pts',(30.8918449793237,8.49524192067261,144.063541126495));
#40111=CARTESIAN_POINT('Ctrl Pts',(30.9268283260648,8.49828304754276,144.043589297463));
#40112=CARTESIAN_POINT('Ctrl Pts',(30.9609289151646,8.5,144.022591867639));
#40113=CARTESIAN_POINT('Ctrl Pts',(30.9949874371066,8.5,144.));
#40114=CARTESIAN_POINT('',(28.8951880620293,8.5,143.921052631579));
#40115=CARTESIAN_POINT('Ctrl Pts',(28.8951880620293,8.5,143.921052631579));
#40116=CARTESIAN_POINT('Ctrl Pts',(28.9307900499921,8.5,143.948731762135));
#40117=CARTESIAN_POINT('Ctrl Pts',(28.9674326867105,8.5,143.975072330207));
#40118=CARTESIAN_POINT('Ctrl Pts',(29.0050125628934,8.5,144.));
#40119=CARTESIAN_POINT('Origin',(30.,8.5,142.5));
#40120=CARTESIAN_POINT('Origin',(37.95,8.45,142.2));
#40121=CARTESIAN_POINT('',(37.9,8.4,136.));
#40122=CARTESIAN_POINT('',(37.9,8.4,136.));
#40123=CARTESIAN_POINT('',(37.9,8.4,144.));
#40124=CARTESIAN_POINT('',(38.,8.5,144.));
#40125=CARTESIAN_POINT('',(37.9,8.4,142.2));
#40126=CARTESIAN_POINT('Origin',(37.95,8.,136.));
#40127=CARTESIAN_POINT('',(37.9,8.,135.6));
#40128=CARTESIAN_POINT('Origin',(37.9,8.,136.));
#40129=CARTESIAN_POINT('',(37.9,8.,135.6));
#40130=CARTESIAN_POINT('Origin',(37.95,7.45,135.55));
#40131=CARTESIAN_POINT('',(37.9,5.,135.6));
#40132=CARTESIAN_POINT('',(37.9,5.,135.6));
#40133=CARTESIAN_POINT('',(37.9,7.45,135.6));
#40134=CARTESIAN_POINT('Origin',(37.95,5.,136.));
#40135=CARTESIAN_POINT('Origin',(37.9,5.,136.));
#40136=CARTESIAN_POINT('',(37.9,4.6,136.));
#40137=CARTESIAN_POINT('Origin',(37.95,4.55,137.8));
#40138=CARTESIAN_POINT('',(37.9,4.6,144.));
#40139=CARTESIAN_POINT('Origin',(37.95,5.,144.));
#40140=CARTESIAN_POINT('',(37.9,5.,144.4));
#40141=CARTESIAN_POINT('Origin',(37.9,5.,144.));
#40142=CARTESIAN_POINT('',(37.9,5.,144.4));
#40143=CARTESIAN_POINT('Origin',(37.95,5.55,144.45));
#40144=CARTESIAN_POINT('',(37.9,8.,144.4));
#40145=CARTESIAN_POINT('',(37.9,8.,144.4));
#40146=CARTESIAN_POINT('',(37.9,5.55,144.4));
#40147=CARTESIAN_POINT('Origin',(37.95,8.,144.));
#40148=CARTESIAN_POINT('Origin',(37.9,8.,144.));
#40149=CARTESIAN_POINT('Origin',(-38.,5.,136.));
#40150=CARTESIAN_POINT('',(-37.9,5.,135.6));
#40151=CARTESIAN_POINT('',(-38.,5.,135.6));
#40152=CARTESIAN_POINT('Origin',(-37.9,5.,136.));
#40153=CARTESIAN_POINT('Origin',(-38.,8.4,135.6));
#40154=CARTESIAN_POINT('',(-37.9,8.,135.6));
#40155=CARTESIAN_POINT('',(-38.,8.,135.6));
#40156=CARTESIAN_POINT('',(-37.9,7.45,135.6));
#40157=CARTESIAN_POINT('Origin',(-38.,8.,136.));
#40158=CARTESIAN_POINT('',(31.1661903789691,8.4,136.));
#40159=CARTESIAN_POINT('',(-38.,8.4,136.));
#40160=CARTESIAN_POINT('',(31.0500544632573,8.39129047171135,135.916983334517));
#40161=CARTESIAN_POINT('Ctrl Pts',(31.0500544632573,8.39129047171135,135.916983334517));
#40162=CARTESIAN_POINT('Ctrl Pts',(31.0899798045429,8.39678689624297,135.942890163407));
#40163=CARTESIAN_POINT('Ctrl Pts',(31.1286105027861,8.4,135.970783139968));
#40164=CARTESIAN_POINT('Ctrl Pts',(31.166190378969,8.4,136.));
#40165=CARTESIAN_POINT('',(30.6614250203353,8.29999999989174,135.735424868771));
#40166=CARTESIAN_POINT('Ctrl Pts',(30.6617871419909,8.29994622735324,135.735320177065));
#40167=CARTESIAN_POINT('Ctrl Pts',(30.775165618415,8.33151941969813,135.770967056611));
#40168=CARTESIAN_POINT('Ctrl Pts',(30.8844578418793,8.36220781029194,135.818396041882));
#40169=CARTESIAN_POINT('Ctrl Pts',(30.9900521410047,8.3815773300417,135.880004886115));
#40170=CARTESIAN_POINT('Ctrl Pts',(31.0017011490688,8.3837141470255,135.886801483368));
#40171=CARTESIAN_POINT('Ctrl Pts',(31.0132512017484,8.38570823783425,135.893775706518));
#40172=CARTESIAN_POINT('Ctrl Pts',(31.0247618982842,8.38753579942467,135.900924376673));
#40173=CARTESIAN_POINT('Ctrl Pts',(31.0332269292893,8.38887979850225,135.906181548932));
#40174=CARTESIAN_POINT('Ctrl Pts',(31.0416572725171,8.39013445090616,135.911534549944));
#40175=CARTESIAN_POINT('Ctrl Pts',(31.0500544632573,8.39129047171136,135.916983334517));
#40176=CARTESIAN_POINT('',(29.338574981678,8.29999999933449,135.735424868139));
#40177=CARTESIAN_POINT('Ctrl Pts',(29.3386278125038,8.30008257895501,135.735540389865));
#40178=CARTESIAN_POINT('Ctrl Pts',(29.5057955176886,8.2535712447323,135.683143176038));
#40179=CARTESIAN_POINT('Ctrl Pts',(29.6838689436387,8.20463519701964,135.655313450655));
#40180=CARTESIAN_POINT('Ctrl Pts',(29.8979263724968,8.18554671829636,135.64548462364));
#40181=CARTESIAN_POINT('Ctrl Pts',(29.9260016099788,8.18385989257095,135.644589352545));
#40182=CARTESIAN_POINT('Ctrl Pts',(29.9790456809631,8.18217256996548,135.643730808771));
#40183=CARTESIAN_POINT('Ctrl Pts',(30.0039642863029,8.18202261194883,135.643653901212));
#40184=CARTESIAN_POINT('Ctrl Pts',(30.0415622629051,8.18276540718812,135.644034960973));
#40185=CARTESIAN_POINT('Ctrl Pts',(30.0542548744622,8.18318172952025,135.644248321544));
#40186=CARTESIAN_POINT('Ctrl Pts',(30.0932530393102,8.1849725865134,135.645173639629));
#40187=CARTESIAN_POINT('Ctrl Pts',(30.1194351443769,8.1868501959716,135.646150752494));
#40188=CARTESIAN_POINT('Ctrl Pts',(30.3267044343054,8.20740656544723,135.657166656925));
#40189=CARTESIAN_POINT('Ctrl Pts',(30.4983000996812,8.25464044598778,135.68404798762));
#40190=CARTESIAN_POINT('Ctrl Pts',(30.6614428655482,8.3000552919959,135.735319109435));
#40191=CARTESIAN_POINT('',(28.9499455367427,8.39129047171135,135.916983334517));
#40192=CARTESIAN_POINT('Ctrl Pts',(28.9499455367427,8.39129047171135,135.916983334517));
#40193=CARTESIAN_POINT('Ctrl Pts',(28.9833499104208,8.38669177291416,135.895307843082));
#40194=CARTESIAN_POINT('Ctrl Pts',(29.0505321085055,8.3745011316311,135.855362112556));
#40195=CARTESIAN_POINT('Ctrl Pts',(29.1793447791299,8.34434708123645,135.791526380412));
#40196=CARTESIAN_POINT('Ctrl Pts',(29.2768237032497,8.31707963998262,135.754802014391));
#40197=CARTESIAN_POINT('Ctrl Pts',(29.3385595046862,8.29989676950243,135.735454721815));
#40198=CARTESIAN_POINT('',(28.8338096210309,8.4,136.));
#40199=CARTESIAN_POINT('Ctrl Pts',(28.8338096210309,8.4,136.));
#40200=CARTESIAN_POINT('Ctrl Pts',(28.8713894972124,8.39999999999963,135.970783139966));
#40201=CARTESIAN_POINT('Ctrl Pts',(28.9100201954571,8.39678689624297,135.942890163407));
#40202=CARTESIAN_POINT('Ctrl Pts',(28.9499455367427,8.39129047171135,135.916983334517));
#40203=CARTESIAN_POINT('',(-28.8338096210309,8.4,136.));
#40204=CARTESIAN_POINT('',(-38.,8.4,136.));
#40205=CARTESIAN_POINT('',(-28.9499455367427,8.39129047171135,135.916983334517));
#40206=CARTESIAN_POINT('Ctrl Pts',(-28.9499455367427,8.39129047171135,135.916983334517));
#40207=CARTESIAN_POINT('Ctrl Pts',(-28.9100201954571,8.39678689624297,135.942890163407));
#40208=CARTESIAN_POINT('Ctrl Pts',(-28.8713894972139,8.4,135.970783139968));
#40209=CARTESIAN_POINT('Ctrl Pts',(-28.833809621031,8.4,136.));
#40210=CARTESIAN_POINT('',(-29.3385749796646,8.29999999989175,135.735424868771));
#40211=CARTESIAN_POINT('Ctrl Pts',(-29.3381669864801,8.30010233118074,135.735322327554));
#40212=CARTESIAN_POINT('Ctrl Pts',(-29.2247952376504,8.33157740613302,135.770950841463));
#40213=CARTESIAN_POINT('Ctrl Pts',(-29.1155062056164,8.36211580901458,135.818341931665));
#40214=CARTESIAN_POINT('Ctrl Pts',(-29.0099454651912,8.3815739822389,135.880001956662));
#40215=CARTESIAN_POINT('Ctrl Pts',(-28.9983001592736,8.38372057934386,135.886804200101));
#40216=CARTESIAN_POINT('Ctrl Pts',(-28.9867478988158,8.3857073377265,135.893774692507));
#40217=CARTESIAN_POINT('Ctrl Pts',(-28.9752376631878,8.38753570208383,135.900923965067));
#40218=CARTESIAN_POINT('Ctrl Pts',(-28.9667729711371,8.38888029152071,135.906181580337));
#40219=CARTESIAN_POINT('Ctrl Pts',(-28.9583427274828,8.39013445090617,135.911534549944));
#40220=CARTESIAN_POINT('Ctrl Pts',(-28.9499455367427,8.39129047171136,135.916983334517));
#40221=CARTESIAN_POINT('',(-30.661425018322,8.29999999933447,135.735424868139));
#40222=CARTESIAN_POINT('Ctrl Pts',(-30.6614403324357,8.29990288566549,135.735450246584));
#40223=CARTESIAN_POINT('Ctrl Pts',(-30.5288224131844,8.26307573905403,135.693849975409));
#40224=CARTESIAN_POINT('Ctrl Pts',(-30.3889944469613,8.22475878909875,135.667443669542));
#40225=CARTESIAN_POINT('Ctrl Pts',(-30.2068474352435,8.19595429131145,135.651012005824));
#40226=CARTESIAN_POINT('Ctrl Pts',(-30.1685015966763,8.19115568892363,135.648342005986));
#40227=CARTESIAN_POINT('Ctrl Pts',(-30.0772899664358,8.18310206076612,135.644103777041));
#40228=CARTESIAN_POINT('Ctrl Pts',(-30.0241258793722,8.18117464424746,135.643151906577));
#40229=CARTESIAN_POINT('Ctrl Pts',(-29.9583002059055,8.18248038026162,135.643821210287));
#40230=CARTESIAN_POINT('Ctrl Pts',(-29.945607880728,8.18289720095053,135.6440346745));
#40231=CARTESIAN_POINT('Ctrl Pts',(-29.9066026001864,8.18468277370489,135.644958149235));
#40232=CARTESIAN_POINT('Ctrl Pts',(-29.8804218187696,8.1865934232616,135.645948287097));
#40233=CARTESIAN_POINT('Ctrl Pts',(-29.7775051143642,8.19662294325174,135.651344091606));
#40234=CARTESIAN_POINT('Ctrl Pts',(-29.6004619510134,8.2275301924826,135.668504490137));
#40235=CARTESIAN_POINT('Ctrl Pts',(-29.4324777206386,8.27391945427491,135.705706123537));
#40236=CARTESIAN_POINT('Ctrl Pts',(-29.3385146936142,8.30000579886974,135.735213097063));
#40237=CARTESIAN_POINT('',(-31.0500544632573,8.39129047171135,135.916983334517));
#40238=CARTESIAN_POINT('Ctrl Pts',(-31.0500544632574,8.39129047171136,135.916983334517));
#40239=CARTESIAN_POINT('Ctrl Pts',(-30.9908315655339,8.38313739956722,135.87855467171));
#40240=CARTESIAN_POINT('Ctrl Pts',(-30.8660346152952,8.35700091284835,135.809286827101));
#40241=CARTESIAN_POINT('Ctrl Pts',(-30.7318879198758,8.31946572940279,135.757548608235));
#40242=CARTESIAN_POINT('Ctrl Pts',(-30.6614403324357,8.29990288566549,135.735450246584));
#40243=CARTESIAN_POINT('',(-31.0754160204889,8.39448466110766,135.933804440098));
#40244=CARTESIAN_POINT('Ctrl Pts',(-31.0754096448176,8.39448483093512,135.933813086818));
#40245=CARTESIAN_POINT('Ctrl Pts',(-31.0670151585375,8.39352977637734,135.92811721501));
#40246=CARTESIAN_POINT('Ctrl Pts',(-31.0585642183151,8.39246198897211,135.922505160031));
#40247=CARTESIAN_POINT('Ctrl Pts',(-31.0500544632573,8.39129047171135,135.916983334517));
#40248=CARTESIAN_POINT('',(-31.1661903789691,8.4,136.));
#40249=CARTESIAN_POINT('Ctrl Pts',(-31.1661903789691,8.4,136.));
#40250=CARTESIAN_POINT('Ctrl Pts',(-31.1366203414292,8.3999999999997,135.97701047114));
#40251=CARTESIAN_POINT('Ctrl Pts',(-31.1063996916262,8.39801061970443,135.954840619422));
#40252=CARTESIAN_POINT('Ctrl Pts',(-31.0754096448176,8.39448483093512,135.933813086818));
#40253=CARTESIAN_POINT('',(-37.9,8.4,136.));
#40254=CARTESIAN_POINT('',(-38.,8.4,136.));
#40255=CARTESIAN_POINT('Origin',(-37.9,8.,136.));
#40256=CARTESIAN_POINT('Origin',(-38.,8.4,144.4));
#40257=CARTESIAN_POINT('',(31.1661903789691,8.4,144.));
#40258=CARTESIAN_POINT('',(-38.,8.4,144.));
#40259=CARTESIAN_POINT('',(28.8338096210309,8.4,144.));
#40260=CARTESIAN_POINT('Origin',(30.,8.4,142.5));
#40261=CARTESIAN_POINT('',(-28.8338096210309,8.4,144.));
#40262=CARTESIAN_POINT('',(-38.,8.4,144.));
#40263=CARTESIAN_POINT('',(-31.1661903789691,8.4,144.));
#40264=CARTESIAN_POINT('Origin',(-30.,8.4,142.5));
#40265=CARTESIAN_POINT('',(-37.9,8.4,144.));
#40266=CARTESIAN_POINT('',(-38.,8.4,144.));
#40267=CARTESIAN_POINT('',(-37.9,8.4,142.2));
#40268=CARTESIAN_POINT('Origin',(-30.,8.4,137.5));
#40269=CARTESIAN_POINT('Origin',(30.,8.4,137.5));
#40270=CARTESIAN_POINT('Origin',(-37.95,8.45,142.2));
#40271=CARTESIAN_POINT('',(-38.,8.5,136.));
#40272=CARTESIAN_POINT('',(-37.9,8.4,144.));
#40273=CARTESIAN_POINT('Origin',(-37.95,8.,136.));
#40274=CARTESIAN_POINT('',(-38.,8.,135.5));
#40275=CARTESIAN_POINT('Origin',(-37.95,7.45,135.55));
#40276=CARTESIAN_POINT('',(-38.,5.,135.5));
#40277=CARTESIAN_POINT('Origin',(-37.95,5.,136.));
#40278=CARTESIAN_POINT('',(-38.,4.50000000000002,136.));
#40279=CARTESIAN_POINT('Origin',(-37.95,4.55,137.8));
#40280=CARTESIAN_POINT('',(-38.,4.5,144.));
#40281=CARTESIAN_POINT('Origin',(-37.95,5.,144.));
#40282=CARTESIAN_POINT('',(-37.9,5.,144.4));
#40283=CARTESIAN_POINT('',(-38.,5.,144.5));
#40284=CARTESIAN_POINT('Origin',(-37.9,5.,144.));
#40285=CARTESIAN_POINT('Origin',(-37.95,5.55,144.45));
#40286=CARTESIAN_POINT('',(-37.9,8.,144.4));
#40287=CARTESIAN_POINT('',(-38.,8.,144.5));
#40288=CARTESIAN_POINT('',(-37.9,5.55,144.4));
#40289=CARTESIAN_POINT('Origin',(-37.95,8.,144.));
#40290=CARTESIAN_POINT('Origin',(-37.9,8.,144.));
#40291=CARTESIAN_POINT('Origin',(-38.,5.,144.));
#40292=CARTESIAN_POINT('',(-38.,5.,144.4));
#40293=CARTESIAN_POINT('Origin',(-38.,4.6,144.4));
#40294=CARTESIAN_POINT('',(-38.,8.,144.4));
#40295=CARTESIAN_POINT('Origin',(-38.,8.,144.));
#40296=CARTESIAN_POINT('',(-31.0500544632573,8.39129047171135,144.083016665483));
#40297=CARTESIAN_POINT('Ctrl Pts',(-31.0500544632573,8.39129047171135,144.083016665483));
#40298=CARTESIAN_POINT('Ctrl Pts',(-31.0899798045429,8.39678689624297,144.057109836593));
#40299=CARTESIAN_POINT('Ctrl Pts',(-31.1286105027861,8.4,144.029216860032));
#40300=CARTESIAN_POINT('Ctrl Pts',(-31.166190378969,8.4,144.));
#40301=CARTESIAN_POINT('',(-30.6614250203354,8.29999999989176,144.264575131229));
#40302=CARTESIAN_POINT('Ctrl Pts',(-30.6618396899871,8.29991781521182,144.264739808957));
#40303=CARTESIAN_POINT('Ctrl Pts',(-30.7751945183757,8.33150592132261,144.229066212155));
#40304=CARTESIAN_POINT('Ctrl Pts',(-30.8844650149679,8.36221060079717,144.181611705071));
#40305=CARTESIAN_POINT('Ctrl Pts',(-30.9900531081148,8.38157715543247,144.119996210819));
#40306=CARTESIAN_POINT('Ctrl Pts',(-31.0017014315445,8.38371364530919,144.113198879946));
#40307=CARTESIAN_POINT('Ctrl Pts',(-31.0132516281393,8.38570812580638,144.106224780502));
#40308=CARTESIAN_POINT('Ctrl Pts',(-31.0247621663533,8.38753570049785,144.099075932216));
#40309=CARTESIAN_POINT('Ctrl Pts',(-31.0332270809276,8.38887970921002,144.093818628959));
#40310=CARTESIAN_POINT('Ctrl Pts',(-31.0416572725171,8.39013445090614,144.088465450056));
#40311=CARTESIAN_POINT('Ctrl Pts',(-31.0500544632573,8.39129047171135,144.083016665483));
#40312=CARTESIAN_POINT('',(-29.338574981678,8.29999999933447,144.264575131861));
#40313=CARTESIAN_POINT('Ctrl Pts',(-29.338652459278,8.30015458067006,144.264432850785));
#40314=CARTESIAN_POINT('Ctrl Pts',(-29.471254955589,8.26335414343341,144.306032812001));
#40315=CARTESIAN_POINT('Ctrl Pts',(-29.6110602576202,8.22506281541357,144.332438307369));
#40316=CARTESIAN_POINT('Ctrl Pts',(-29.7931828978245,8.19627966997637,144.348871433016));
#40317=CARTESIAN_POINT('Ctrl Pts',(-29.8315050694548,8.19147962387844,144.351541055828));
#40318=CARTESIAN_POINT('Ctrl Pts',(-29.8980881273779,8.18561185509721,144.354637251728));
#40319=CARTESIAN_POINT('Ctrl Pts',(-29.9261331455688,8.18390663041651,144.355518923594));
#40320=CARTESIAN_POINT('Ctrl Pts',(-29.9791768427067,8.18222339100664,144.356378794531));
#40321=CARTESIAN_POINT('Ctrl Pts',(-30.0040925088588,8.18207177302637,144.356454836261));
#40322=CARTESIAN_POINT('Ctrl Pts',(-30.0416869686119,8.18281540243689,144.356073075862));
#40323=CARTESIAN_POINT('Ctrl Pts',(-30.0543793900807,8.18323091163571,144.355860174902));
#40324=CARTESIAN_POINT('Ctrl Pts',(-30.0933740369497,8.18502349243028,144.354933142189));
#40325=CARTESIAN_POINT('Ctrl Pts',(-30.1195554386871,8.18690252431569,144.353956583673));
#40326=CARTESIAN_POINT('Ctrl Pts',(-30.326804087216,8.2074032973194,144.342951164697));
#40327=CARTESIAN_POINT('Ctrl Pts',(-30.4983498772685,8.25464807568585,144.316029140081));
#40328=CARTESIAN_POINT('Ctrl Pts',(-30.661449901242,8.30007700746228,144.264722411094));
#40329=CARTESIAN_POINT('',(-28.9499455367427,8.39129047171135,144.083016665483));
#40330=CARTESIAN_POINT('Ctrl Pts',(-28.9499455367427,8.39129047171135,144.083016665483));
#40331=CARTESIAN_POINT('Ctrl Pts',(-29.009168434466,8.38313739956723,144.121445328289));
#40332=CARTESIAN_POINT('Ctrl Pts',(-29.1339710420765,8.35700176313992,144.190714621136));
#40333=CARTESIAN_POINT('Ctrl Pts',(-29.2681148397227,8.3194718198051,144.242448628163));
#40334=CARTESIAN_POINT('Ctrl Pts',(-29.3385631777598,8.29991175184865,144.264544801319));
#40335=CARTESIAN_POINT('Ctrl Pts',(-28.8338096210309,8.4,144.));
#40336=CARTESIAN_POINT('Ctrl Pts',(-28.8713894972124,8.39999999999963,144.029216860034));
#40337=CARTESIAN_POINT('Ctrl Pts',(-28.9100201954571,8.39678689624297,144.057109836593));
#40338=CARTESIAN_POINT('Ctrl Pts',(-28.9499455367427,8.39129047171135,144.083016665483));
#40339=CARTESIAN_POINT('',(28.9499455367427,8.39129047171135,144.083016665483));
#40340=CARTESIAN_POINT('Ctrl Pts',(28.9499455367427,8.39129047171135,144.083016665483));
#40341=CARTESIAN_POINT('Ctrl Pts',(28.9100201954571,8.39678689624297,144.057109836593));
#40342=CARTESIAN_POINT('Ctrl Pts',(28.8713894972139,8.4,144.029216860032));
#40343=CARTESIAN_POINT('Ctrl Pts',(28.833809621031,8.4,144.));
#40344=CARTESIAN_POINT('',(29.3385749796647,8.29999999989175,144.264575131229));
#40345=CARTESIAN_POINT('Ctrl Pts',(29.3382753761609,8.30022001211062,144.264570458976));
#40346=CARTESIAN_POINT('Ctrl Pts',(29.2248705789997,8.33165596203575,144.228985346631));
#40347=CARTESIAN_POINT('Ctrl Pts',(29.115491058347,8.36206433955672,144.181672395662));
#40348=CARTESIAN_POINT('Ctrl Pts',(29.0099464509446,8.38157135670728,144.119998131135));
#40349=CARTESIAN_POINT('Ctrl Pts',(28.9983029247983,8.38372334220249,144.113194316812));
#40350=CARTESIAN_POINT('Ctrl Pts',(28.9867485261411,8.38570645439427,144.106225228903));
#40351=CARTESIAN_POINT('Ctrl Pts',(28.9752382142316,8.38753536993229,144.099075890131));
#40352=CARTESIAN_POINT('Ctrl Pts',(28.9667734660829,8.38888036471055,144.093818226167));
#40353=CARTESIAN_POINT('Ctrl Pts',(28.9583427274828,8.39013445090616,144.088465450056));
#40354=CARTESIAN_POINT('Ctrl Pts',(28.9499455367427,8.39129047171136,144.083016665483));
#40355=CARTESIAN_POINT('',(30.661425018322,8.29999999933449,144.264575131861));
#40356=CARTESIAN_POINT('Ctrl Pts',(30.6614433761257,8.29987533145044,144.264537899321));
#40357=CARTESIAN_POINT('Ctrl Pts',(30.4943037331861,8.25333014297023,144.316908600203));
#40358=CARTESIAN_POINT('Ctrl Pts',(30.3162632139204,8.20435742950814,144.344707484172));
#40359=CARTESIAN_POINT('Ctrl Pts',(30.1021065839386,8.18529590996961,144.354567989873));
#40360=CARTESIAN_POINT('Ctrl Pts',(30.074028637424,8.18360776495036,144.355462743862));
#40361=CARTESIAN_POINT('Ctrl Pts',(30.0209792504149,8.18191724490555,144.356319890362));
#40362=CARTESIAN_POINT('Ctrl Pts',(29.9960550388621,8.18176901342238,144.356398301945));
#40363=CARTESIAN_POINT('Ctrl Pts',(29.9584499596871,8.18250975841238,144.356016804967));
#40364=CARTESIAN_POINT('Ctrl Pts',(29.9457591107073,8.18293041085672,144.355804314577));
#40365=CARTESIAN_POINT('Ctrl Pts',(29.8489171025918,8.18733644430337,144.353503744874));
#40366=CARTESIAN_POINT('Ctrl Pts',(29.6834564814262,8.20996035010193,144.34210623907));
#40367=CARTESIAN_POINT('Ctrl Pts',(29.4880447175627,8.25873483980795,144.307413737166));
#40368=CARTESIAN_POINT('Ctrl Pts',(29.3751540243146,8.28999725964461,144.276134934077));
#40369=CARTESIAN_POINT('Ctrl Pts',(29.3385834550246,8.30013461249329,144.264667098602));
#40370=CARTESIAN_POINT('',(31.0500544632573,8.39129047171135,144.083016665483));
#40371=CARTESIAN_POINT('Ctrl Pts',(31.0500544632573,8.39129047171135,144.083016665483));
#40372=CARTESIAN_POINT('Ctrl Pts',(31.0166500895791,8.38669177291414,144.104692156918));
#40373=CARTESIAN_POINT('Ctrl Pts',(30.9494752442691,8.37449659083024,144.144633707188));
#40374=CARTESIAN_POINT('Ctrl Pts',(30.8206483458436,8.34434509414795,144.208476224786));
#40375=CARTESIAN_POINT('Ctrl Pts',(30.7231761413096,8.31706672387149,144.245194863023));
#40376=CARTESIAN_POINT('Ctrl Pts',(30.6614433761257,8.29987533145044,144.264537899321));
#40377=CARTESIAN_POINT('',(31.0754160204992,8.39448466110884,144.066195559895));
#40378=CARTESIAN_POINT('Ctrl Pts',(31.0754096448279,8.3944848309363,144.066186913175));
#40379=CARTESIAN_POINT('Ctrl Pts',(31.0670151585444,8.39352977637821,144.071882784985));
#40380=CARTESIAN_POINT('Ctrl Pts',(31.0585642183186,8.39246198897259,144.077494839966));
#40381=CARTESIAN_POINT('Ctrl Pts',(31.0500544632573,8.39129047171135,144.083016665483));
#40382=CARTESIAN_POINT('Ctrl Pts',(31.1661903789691,8.4,144.));
#40383=CARTESIAN_POINT('Ctrl Pts',(31.1366203414324,8.39999999999971,144.022989528857));
#40384=CARTESIAN_POINT('Ctrl Pts',(31.1063996916329,8.39801061970488,144.045159380573));
#40385=CARTESIAN_POINT('Ctrl Pts',(31.0754096448279,8.3944848309363,144.066186913175));
#40386=CARTESIAN_POINT('Ctrl Pts',(28.9499455367427,8.39129047171135,144.083016665483));
#40387=CARTESIAN_POINT('Ctrl Pts',(28.9583427274828,8.39013445090615,144.088465450056));
#40388=CARTESIAN_POINT('Ctrl Pts',(28.9667734660829,8.38888036471054,144.093818226167));
#40389=CARTESIAN_POINT('Ctrl Pts',(28.9867485261411,8.38570645439426,144.106225228903));
#40390=CARTESIAN_POINT('Ctrl Pts',(28.9983029247983,8.38372334220247,144.113194316812));
#40391=CARTESIAN_POINT('Ctrl Pts',(29.1496202725203,8.35575649321004,144.201615566941));
#40392=CARTESIAN_POINT('Ctrl Pts',(29.3692050696252,8.28839704166518,144.286315495019));
#40393=CARTESIAN_POINT('Ctrl Pts',(29.6834564814262,8.20996035010193,144.34210623907));
#40394=CARTESIAN_POINT('Ctrl Pts',(29.8489171025918,8.18733644430337,144.353503744874));
#40395=CARTESIAN_POINT('Ctrl Pts',(29.9457591107073,8.18293041085672,144.355804314577));
#40396=CARTESIAN_POINT('Ctrl Pts',(29.9584499596871,8.18250975841238,144.356016804967));
#40397=CARTESIAN_POINT('Ctrl Pts',(29.9960550388621,8.18176901342238,144.356398301945));
#40398=CARTESIAN_POINT('Ctrl Pts',(30.0209792504149,8.18191724490555,144.356319890362));
#40399=CARTESIAN_POINT('Ctrl Pts',(30.074028637424,8.18360776495036,144.355462743862));
#40400=CARTESIAN_POINT('Ctrl Pts',(30.1021065839386,8.18529590996961,144.354567989873));
#40401=CARTESIAN_POINT('Ctrl Pts',(30.3850503615939,8.21047999297718,144.341540287986));
#40402=CARTESIAN_POINT('Ctrl Pts',(30.6646454100207,8.30783313849756,144.285786323045));
#40403=CARTESIAN_POINT('Ctrl Pts',(30.9494752442691,8.37449659083024,144.144633707188));
#40404=CARTESIAN_POINT('Ctrl Pts',(31.0166500895791,8.38669177291414,144.104692156918));
#40405=CARTESIAN_POINT('Ctrl Pts',(31.0500544632573,8.39129047171135,144.083016665483));
#40406=CARTESIAN_POINT('Ctrl Pts',(28.9683012121262,8.4275269811409,144.055344443655));
#40407=CARTESIAN_POINT('Ctrl Pts',(28.9767513031944,8.42675710035562,144.060870100283));
#40408=CARTESIAN_POINT('Ctrl Pts',(28.9852390011866,8.42588181711275,144.06630220525));
#40409=CARTESIAN_POINT('Ctrl Pts',(29.0053237629384,8.4235986014281,144.078903194632));
#40410=CARTESIAN_POINT('Ctrl Pts',(29.0169525178044,8.42211351066722,144.085988008261));
#40411=CARTESIAN_POINT('Ctrl Pts',(29.1689435287771,8.40060024527846,144.175976886636));
#40412=CARTESIAN_POINT('Ctrl Pts',(29.3886619077997,8.34023129010989,144.263730862112));
#40413=CARTESIAN_POINT('Ctrl Pts',(29.696681571984,8.2683613847734,144.32250041751));
#40414=CARTESIAN_POINT('Ctrl Pts',(29.8556533021349,8.24775166628686,144.334588797671));
#40415=CARTESIAN_POINT('Ctrl Pts',(29.9481782437644,8.24373599383981,144.337025491425));
#40416=CARTESIAN_POINT('Ctrl Pts',(29.96031140905,8.24335735060291,144.337249855718));
#40417=CARTESIAN_POINT('Ctrl Pts',(29.9962175677341,8.24267481277293,144.337656505504));
#40418=CARTESIAN_POINT('Ctrl Pts',(30.0200334024999,8.24282657196158,144.337568458374));
#40419=CARTESIAN_POINT('Ctrl Pts',(30.0706836000534,8.24433573825835,144.336668567379));
#40420=CARTESIAN_POINT('Ctrl Pts',(30.0975914106849,8.24592098169161,144.335706222849));
#40421=CARTESIAN_POINT('Ctrl Pts',(30.3682304958345,8.26852298441906,144.322002439928));
#40422=CARTESIAN_POINT('Ctrl Pts',(30.6450768082368,8.35906946466354,144.262471796798));
#40423=CARTESIAN_POINT('Ctrl Pts',(30.9305532331129,8.41520829163761,144.117944392387));
#40424=CARTESIAN_POINT('Ctrl Pts',(30.9980737545343,8.42441643284468,144.07732956379));
#40425=CARTESIAN_POINT('Ctrl Pts',(31.0316987878737,8.4275269811409,144.055344443655));
#40426=CARTESIAN_POINT('Ctrl Pts',(28.9866568875098,8.46376349057045,144.027672221828));
#40427=CARTESIAN_POINT('Ctrl Pts',(28.9951656176985,8.46337735055053,144.033274492976));
#40428=CARTESIAN_POINT('Ctrl Pts',(29.0036963658584,8.46288647378579,144.038786592855));
#40429=CARTESIAN_POINT('Ctrl Pts',(29.0239120783231,8.46148451114518,144.051580700947));
#40430=CARTESIAN_POINT('Ctrl Pts',(29.0355841910455,8.46051102292033,144.0587825374));
#40431=CARTESIAN_POINT('Ctrl Pts',(29.1883722702047,8.44537883300728,144.150336526785));
#40432=CARTESIAN_POINT('Ctrl Pts',(29.4080510514443,8.39198253043129,144.241165142077));
#40433=CARTESIAN_POINT('Ctrl Pts',(29.7098850519141,8.32670316605924,144.302908829508));
#40434=CARTESIAN_POINT('Ctrl Pts',(29.8622371244374,8.30806763961565,144.315696400422));
#40435=CARTESIAN_POINT('Ctrl Pts',(29.9505369330349,8.30446143099731,144.31827031418));
#40436=CARTESIAN_POINT('Ctrl Pts',(29.9620897184856,8.30411312061956,144.318508990909));
#40437=CARTESIAN_POINT('Ctrl Pts',(29.9963286954253,8.30351381528359,144.318933779595));
#40438=CARTESIAN_POINT('Ctrl Pts',(30.0189812519047,8.30362149184793,144.318850133658));
#40439=CARTESIAN_POINT('Ctrl Pts',(30.0673145445624,8.30502408395499,144.317885132574));
#40440=CARTESIAN_POINT('Ctrl Pts',(30.0929171127796,8.30638847697522,144.316890878399));
#40441=CARTESIAN_POINT('Ctrl Pts',(30.3521431978363,8.32703726600895,144.302319082293));
#40442=CARTESIAN_POINT('Ctrl Pts',(30.6253675036887,8.41040735865498,144.239151079469));
#40443=CARTESIAN_POINT('Ctrl Pts',(30.9116497481213,8.45585439427816,144.091276042087));
#40444=CARTESIAN_POINT('Ctrl Pts',(30.9795052502094,8.46227534006946,144.049954460767));
#40445=CARTESIAN_POINT('Ctrl Pts',(31.0133431124902,8.46376349057045,144.027672221828));
#40446=CARTESIAN_POINT('Ctrl Pts',(29.0050125628934,8.5,144.));
#40447=CARTESIAN_POINT('Ctrl Pts',(29.01357419341,8.5,144.005679143204));
#40448=CARTESIAN_POINT('Ctrl Pts',(29.0221619009622,8.49988792618801,144.011270571938));
#40449=CARTESIAN_POINT('Ctrl Pts',(29.0424873151203,8.49937665817902,144.024258666676));
#40450=CARTESIAN_POINT('Ctrl Pts',(29.0542337840516,8.49890119138508,144.031576228849));
#40451=CARTESIAN_POINT('Ctrl Pts',(29.2076955264615,8.4902225850757,144.12469784648));
#40452=CARTESIAN_POINT('Ctrl Pts',(29.4275078896188,8.44381677887601,144.218580509171));
#40453=CARTESIAN_POINT('Ctrl Pts',(29.7231101424719,8.38510420073072,144.283303007947));
#40454=CARTESIAN_POINT('Ctrl Pts',(29.8689733239806,8.36848286159914,144.296781453219));
#40455=CARTESIAN_POINT('Ctrl Pts',(29.9529560660921,8.36526701398041,144.299491491028));
#40456=CARTESIAN_POINT('Ctrl Pts',(29.9639511678485,8.36496071281008,144.29974204166));
#40457=CARTESIAN_POINT('Ctrl Pts',(29.9964912242973,8.36441961463413,144.300191983155));
#40458=CARTESIAN_POINT('Ctrl Pts',(30.0180354039898,8.36453081890395,144.30009870167));
#40459=CARTESIAN_POINT('Ctrl Pts',(30.0639695071918,8.36575205726298,144.299090956091));
#40460=CARTESIAN_POINT('Ctrl Pts',(30.0884019395258,8.36701354869723,144.298029111375));
#40461=CARTESIAN_POINT('Ctrl Pts',(30.3353233320769,8.38508025745083,144.282781234235));
#40462=CARTESIAN_POINT('Ctrl Pts',(30.6057989019047,8.46164368482096,144.215836553222));
#40463=CARTESIAN_POINT('Ctrl Pts',(30.892727736965,8.49656609508553,144.064586727286));
#40464=CARTESIAN_POINT('Ctrl Pts',(30.9609289151646,8.5,144.022591867639));
#40465=CARTESIAN_POINT('Ctrl Pts',(30.9949874371066,8.5,144.));
#40466=CARTESIAN_POINT('',(28.9499455367427,8.39129047171135,144.083016665483));
#40467=CARTESIAN_POINT('',(30.9949874371066,8.5,144.));
#40468=CARTESIAN_POINT('Origin',(30.,8.45,142.5));
#40469=CARTESIAN_POINT('',(31.1661903789691,8.4,144.));
#40470=CARTESIAN_POINT('',(28.8951880620293,8.5,143.921052631579));
#40471=CARTESIAN_POINT('Ctrl Pts',(31.0500544632573,8.39129047171135,144.083016665483));
#40472=CARTESIAN_POINT('Ctrl Pts',(31.0899798051577,8.39678689632762,144.057109836194));
#40473=CARTESIAN_POINT('Ctrl Pts',(31.1286105039774,8.40000000009859,144.029216859175));
#40474=CARTESIAN_POINT('Ctrl Pts',(31.1661903807052,8.4,143.99999999865));
#40475=CARTESIAN_POINT('Ctrl Pts',(31.0316987878737,8.4275269811409,144.055344443655));
#40476=CARTESIAN_POINT('Ctrl Pts',(31.0708423080612,8.43119126421841,144.029764000737));
#40477=CARTESIAN_POINT('Ctrl Pts',(31.1088103196971,8.43333333339906,144.002388493225));
#40478=CARTESIAN_POINT('Ctrl Pts',(31.145730900342,8.43333333333333,143.9736842092));
#40479=CARTESIAN_POINT('Ctrl Pts',(31.0133431124902,8.46376349057045,144.027672221828));
#40480=CARTESIAN_POINT('Ctrl Pts',(31.0517048109648,8.46559563210921,144.00241816528));
#40481=CARTESIAN_POINT('Ctrl Pts',(31.0890101354168,8.46666666669953,143.975560127274));
#40482=CARTESIAN_POINT('Ctrl Pts',(31.1252714199787,8.46666666666667,143.94736841975));
#40483=CARTESIAN_POINT('Ctrl Pts',(30.9949874371066,8.5,144.));
#40484=CARTESIAN_POINT('Ctrl Pts',(31.0325673138683,8.5,143.975072329823));
#40485=CARTESIAN_POINT('Ctrl Pts',(31.0692099511365,8.5,143.948731761324));
#40486=CARTESIAN_POINT('Ctrl Pts',(31.1048119396155,8.5,143.9210526303));
#40487=CARTESIAN_POINT('Ctrl Pts',(28.833809621031,8.4,144.));
#40488=CARTESIAN_POINT('Ctrl Pts',(28.8713894972139,8.4,144.029216860032));
#40489=CARTESIAN_POINT('Ctrl Pts',(28.9100201954571,8.39678689624297,144.057109836593));
#40490=CARTESIAN_POINT('Ctrl Pts',(28.9499455367427,8.39129047171135,144.083016665483));
#40491=CARTESIAN_POINT('Ctrl Pts',(28.8542691013637,8.43333333333333,143.973684210526));
#40492=CARTESIAN_POINT('Ctrl Pts',(28.8911896814733,8.43333333333333,144.002388494066));
#40493=CARTESIAN_POINT('Ctrl Pts',(28.9291576925416,8.43119126416198,144.029764001131));
#40494=CARTESIAN_POINT('Ctrl Pts',(28.9683012121263,8.4275269811409,144.055344443655));
#40495=CARTESIAN_POINT('Ctrl Pts',(28.8747285816965,8.46666666666667,143.947368421053));
#40496=CARTESIAN_POINT('Ctrl Pts',(28.9109898657327,8.46666666666667,143.975560128101));
#40497=CARTESIAN_POINT('Ctrl Pts',(28.948295189626,8.46559563208099,144.002418165669));
#40498=CARTESIAN_POINT('Ctrl Pts',(28.9866568875098,8.46376349057045,144.027672221828));
#40499=CARTESIAN_POINT('Ctrl Pts',(28.8951880620293,8.5,143.921052631579));
#40500=CARTESIAN_POINT('Ctrl Pts',(28.9307900499921,8.5,143.948731762135));
#40501=CARTESIAN_POINT('Ctrl Pts',(28.9674326867105,8.5,143.975072330207));
#40502=CARTESIAN_POINT('Ctrl Pts',(29.0050125628934,8.5,144.));
#40503=CARTESIAN_POINT('Origin',(-30.,8.95,137.5));
#40504=CARTESIAN_POINT('',(-29.19613123823,8.9,135.889473684211));
#40505=CARTESIAN_POINT('',(-29.1514718625761,9.,135.8));
#40506=CARTESIAN_POINT('',(-31.8,8.9,137.5));
#40507=CARTESIAN_POINT('Origin',(-30.,8.9,137.5));
#40508=CARTESIAN_POINT('',(-30.80386876177,8.9,135.889473684211));
#40509=CARTESIAN_POINT('Origin',(-30.,8.9,137.5));
#40510=CARTESIAN_POINT('',(-30.80386876177,8.9,135.889473684211));
#40511=CARTESIAN_POINT('Ctrl Pts',(-30.62442393624,8.99442305443429,135.70570254201));
#40512=CARTESIAN_POINT('Ctrl Pts',(-30.6031336007837,8.99354972599348,135.698345055793));
#40513=CARTESIAN_POINT('Ctrl Pts',(-30.5816752394099,8.99263100796461,135.691382689721));
#40514=CARTESIAN_POINT('Ctrl Pts',(-30.4123094665995,8.98495128128084,135.639444028187));
#40515=CARTESIAN_POINT('Ctrl Pts',(-30.1802232821902,8.97487183787893,135.600774173325));
#40516=CARTESIAN_POINT('Ctrl Pts',(-29.8198774693527,8.97481364719588,135.600649477793));
#40517=CARTESIAN_POINT('Ctrl Pts',(-29.5876626138109,8.9849459908676,135.639432675438));
#40518=CARTESIAN_POINT('Ctrl Pts',(-29.418327451187,8.9926309002887,135.691382459919));
#40519=CARTESIAN_POINT('Ctrl Pts',(-29.3968663992163,8.99354972599348,135.698345055793));
#40520=CARTESIAN_POINT('Ctrl Pts',(-29.37557606376,8.99442305443429,135.70570254201));
#40521=CARTESIAN_POINT('Ctrl Pts',(-30.6134852835967,8.96294870295619,135.737135028007));
#40522=CARTESIAN_POINT('Ctrl Pts',(-30.5926585146851,8.96237089086999,135.729918298573));
#40523=CARTESIAN_POINT('Ctrl Pts',(-30.5716540370928,8.96172231480688,135.723090172466));
#40524=CARTESIAN_POINT('Ctrl Pts',(-30.4057627068958,8.95618694003155,135.671989821309));
#40525=CARTESIAN_POINT('Ctrl Pts',(-30.1774809150283,8.94781763959255,135.633524301555));
#40526=CARTESIAN_POINT('Ctrl Pts',(-29.8226191720034,8.94775803303614,135.63340083736));
#40527=CARTESIAN_POINT('Ctrl Pts',(-29.5942099936947,8.9561825817824,135.671977657888));
#40528=CARTESIAN_POINT('Ctrl Pts',(-29.4283485325563,8.96172203669287,135.723090090889));
#40529=CARTESIAN_POINT('Ctrl Pts',(-29.4073415857357,8.96237102991341,135.729918177652));
#40530=CARTESIAN_POINT('Ctrl Pts',(-29.3865147164033,8.96294870295619,135.737135028007));
#40531=CARTESIAN_POINT('Ctrl Pts',(-30.6025466309533,8.9314743514781,135.768567514003));
#40532=CARTESIAN_POINT('Ctrl Pts',(-30.582184785483,8.93117883512348,135.761502062769));
#40533=CARTESIAN_POINT('Ctrl Pts',(-30.5616314866267,8.93082738428349,135.754786613406));
#40534=CARTESIAN_POINT('Ctrl Pts',(-30.3992200288979,8.92734716856885,135.704598391766));
#40535=CARTESIAN_POINT('Ctrl Pts',(-30.1747360509692,8.92072266060556,135.666303758425));
#40536=CARTESIAN_POINT('Ctrl Pts',(-29.8253607851682,8.92068624425422,135.666171804744));
#40537=CARTESIAN_POINT('Ctrl Pts',(-29.6007527034052,8.92734279840361,135.704587303278));
#40538=CARTESIAN_POINT('Ctrl Pts',(-29.4383712024403,8.93082748462832,135.75478622414));
#40539=CARTESIAN_POINT('Ctrl Pts',(-29.4178151140962,8.93117869608006,135.761502183691));
#40540=CARTESIAN_POINT('Ctrl Pts',(-29.3974533690467,8.9314743514781,135.768567514003));
#40541=CARTESIAN_POINT('Ctrl Pts',(-30.59160797831,8.9,135.8));
#40542=CARTESIAN_POINT('Ctrl Pts',(-30.5717096993844,8.9,135.793075305549));
#40543=CARTESIAN_POINT('Ctrl Pts',(-30.5516102843096,8.89991869112576,135.786494096152));
#40544=CARTESIAN_POINT('Ctrl Pts',(-30.3926732691942,8.89858282731956,135.737144184887));
#40545=CARTESIAN_POINT('Ctrl Pts',(-30.1719936838072,8.89366846231917,135.699053886655));
#40546=CARTESIAN_POINT('Ctrl Pts',(-29.8281024878188,8.89363063009448,135.698923164311));
#40547=CARTESIAN_POINT('Ctrl Pts',(-29.607300083289,8.89857938931841,135.737132285728));
#40548=CARTESIAN_POINT('Ctrl Pts',(-29.4483922838095,8.89991862103249,135.78649385511));
#40549=CARTESIAN_POINT('Ctrl Pts',(-29.4282903006156,8.9,135.793075305549));
#40550=CARTESIAN_POINT('Ctrl Pts',(-29.40839202169,8.9,135.8));
#40551=CARTESIAN_POINT('',(-29.40839202169,8.9,135.8));
#40552=CARTESIAN_POINT('',(-29.40839202169,8.9,135.8));
#40553=CARTESIAN_POINT('',(-30.59160797831,8.9,135.8));
#40554=CARTESIAN_POINT('',(-30.62442393624,8.99442305443429,135.70570254201));
#40555=CARTESIAN_POINT('Ctrl Pts',(-30.59160797831,8.9,135.8));
#40556=CARTESIAN_POINT('Ctrl Pts',(-30.5717096993844,8.9,135.793075305549));
#40557=CARTESIAN_POINT('Ctrl Pts',(-30.5516102843096,8.89991869112576,135.786494096152));
#40558=CARTESIAN_POINT('Ctrl Pts',(-30.3926732691942,8.89858282731956,135.737144184887));
#40559=CARTESIAN_POINT('Ctrl Pts',(-30.1719936838072,8.89366846231917,135.699053886655));
#40560=CARTESIAN_POINT('Ctrl Pts',(-29.8281024878188,8.89363063009448,135.698923164311));
#40561=CARTESIAN_POINT('Ctrl Pts',(-29.607300083289,8.89857938931841,135.737132285728));
#40562=CARTESIAN_POINT('Ctrl Pts',(-29.4483922838095,8.89991862103249,135.78649385511));
#40563=CARTESIAN_POINT('Ctrl Pts',(-29.4282903006156,8.9,135.793075305549));
#40564=CARTESIAN_POINT('Ctrl Pts',(-29.40839202169,8.9,135.8));
#40565=CARTESIAN_POINT('Ctrl Pts',(-30.8485281374239,9.,135.8));
#40566=CARTESIAN_POINT('Ctrl Pts',(-30.7759616147067,9.,135.763779566847));
#40567=CARTESIAN_POINT('Ctrl Pts',(-30.7010733797628,8.99756721057679,135.732190956222));
#40568=CARTESIAN_POINT('Ctrl Pts',(-30.62442393624,8.99442305443429,135.70570254201));
#40569=CARTESIAN_POINT('Ctrl Pts',(-30.8336416788726,8.96666666666667,135.829824561404));
#40570=CARTESIAN_POINT('Ctrl Pts',(-30.7623482530451,8.96666666666667,135.794239574446));
#40571=CARTESIAN_POINT('Ctrl Pts',(-30.6887737535176,8.96504480705119,135.763211800971));
#40572=CARTESIAN_POINT('Ctrl Pts',(-30.6134852835966,8.96294870295619,135.737135028007));
#40573=CARTESIAN_POINT('Ctrl Pts',(-30.8187552203213,8.93333333333333,135.859649122807));
#40574=CARTESIAN_POINT('Ctrl Pts',(-30.7487348913836,8.93333333333333,135.824699582045));
#40575=CARTESIAN_POINT('Ctrl Pts',(-30.6764741272724,8.9325224035256,135.79423264572));
#40576=CARTESIAN_POINT('Ctrl Pts',(-30.6025466309533,8.9314743514781,135.768567514003));
#40577=CARTESIAN_POINT('Ctrl Pts',(-30.80386876177,8.9,135.889473684211));
#40578=CARTESIAN_POINT('Ctrl Pts',(-30.7351215297221,8.9,135.855159589644));
#40579=CARTESIAN_POINT('Ctrl Pts',(-30.6641745010272,8.9,135.825253490469));
#40580=CARTESIAN_POINT('Ctrl Pts',(-30.59160797831,8.9,135.8));
#40581=CARTESIAN_POINT('Ctrl Pts',(-30.80386876177,8.9,135.889473684211));
#40582=CARTESIAN_POINT('Ctrl Pts',(-30.7351215297221,8.9,135.855159589644));
#40583=CARTESIAN_POINT('Ctrl Pts',(-30.6641745010272,8.9,135.825253490469));
#40584=CARTESIAN_POINT('Ctrl Pts',(-30.59160797831,8.9,135.8));
#40585=CARTESIAN_POINT('Ctrl Pts',(-29.37557606376,8.99442305443429,135.70570254201));
#40586=CARTESIAN_POINT('Ctrl Pts',(-29.2989266202368,8.99756721057681,135.732190956222));
#40587=CARTESIAN_POINT('Ctrl Pts',(-29.2240383852925,9.00000000000003,135.763779566847));
#40588=CARTESIAN_POINT('Ctrl Pts',(-29.1514718625749,9.,135.800000000001));
#40589=CARTESIAN_POINT('Ctrl Pts',(-29.3865147164033,8.96294870295619,135.737135028007));
#40590=CARTESIAN_POINT('Ctrl Pts',(-29.311226246482,8.96504480705121,135.763211800971));
#40591=CARTESIAN_POINT('Ctrl Pts',(-29.237651746954,8.96666666666669,135.794239574446));
#40592=CARTESIAN_POINT('Ctrl Pts',(-29.1663583211262,8.96666666666667,135.829824561404));
#40593=CARTESIAN_POINT('Ctrl Pts',(-29.3974533690467,8.9314743514781,135.768567514003));
#40594=CARTESIAN_POINT('Ctrl Pts',(-29.3235258727272,8.9325224035256,135.79423264572));
#40595=CARTESIAN_POINT('Ctrl Pts',(-29.2512651086155,8.93333333333334,135.824699582045));
#40596=CARTESIAN_POINT('Ctrl Pts',(-29.1812447796775,8.93333333333333,135.859649122808));
#40597=CARTESIAN_POINT('Ctrl Pts',(-29.40839202169,8.9,135.8));
#40598=CARTESIAN_POINT('Ctrl Pts',(-29.3358254989724,8.9,135.825253490469));
#40599=CARTESIAN_POINT('Ctrl Pts',(-29.2648784702771,8.9,135.855159589645));
#40600=CARTESIAN_POINT('Ctrl Pts',(-29.1961312382288,8.9,135.889473684211));
#40601=CARTESIAN_POINT('Ctrl Pts',(-29.40839202169,8.9,135.8));
#40602=CARTESIAN_POINT('Ctrl Pts',(-29.3358254989724,8.9,135.825253490469));
#40603=CARTESIAN_POINT('Ctrl Pts',(-29.2648784702771,8.9,135.855159589645));
#40604=CARTESIAN_POINT('Ctrl Pts',(-29.1961312382288,8.9,135.889473684211));
#40605=CARTESIAN_POINT('Origin',(-30.,9.1,137.5));
#40606=CARTESIAN_POINT('',(-31.8,8.5,137.5));
#40607=CARTESIAN_POINT('',(-31.8,9.1,137.5));
#40608=CARTESIAN_POINT('',(-31.1048119379707,8.5,136.078947368421));
#40609=CARTESIAN_POINT('Origin',(-30.,8.5,137.5));
#40610=CARTESIAN_POINT('',(-30.9949874371066,8.5,136.));
#40611=CARTESIAN_POINT('Ctrl Pts',(-30.9949874371066,8.5,136.));
#40612=CARTESIAN_POINT('Ctrl Pts',(-31.0325673132895,8.5,136.024927669793));
#40613=CARTESIAN_POINT('Ctrl Pts',(-31.0692099500079,8.5,136.051268237865));
#40614=CARTESIAN_POINT('Ctrl Pts',(-31.1048119379707,8.5,136.078947368421));
#40615=CARTESIAN_POINT('',(-29.0050125628934,8.5,136.));
#40616=CARTESIAN_POINT('Ctrl Pts',(-29.0050125628934,8.5,136.));
#40617=CARTESIAN_POINT('Ctrl Pts',(-29.0135741934101,8.5,135.994320856796));
#40618=CARTESIAN_POINT('Ctrl Pts',(-29.0221618769299,8.4998881340947,135.988729270797));
#40619=CARTESIAN_POINT('Ctrl Pts',(-29.0307744240967,8.49967145659893,135.98322540583));
#40620=CARTESIAN_POINT('Ctrl Pts',(-29.0424857121922,8.49937681988721,135.975741284465));
#40621=CARTESIAN_POINT('Ctrl Pts',(-29.0542374418331,8.49890259856716,135.968422529549));
#40622=CARTESIAN_POINT('Ctrl Pts',(-29.0660378041393,8.49823351737356,135.961258388211));
#40623=CARTESIAN_POINT('Ctrl Pts',(-29.2617610405741,8.48713599907278,135.842432466379));
#40624=CARTESIAN_POINT('Ctrl Pts',(-29.4674506362191,8.43232113429692,135.768015720858));
#40625=CARTESIAN_POINT('Ctrl Pts',(-29.6708139777886,8.3968702701052,135.730147139424));
#40626=CARTESIAN_POINT('Ctrl Pts',(-29.7386017583118,8.38505331537463,135.717524278947));
#40627=CARTESIAN_POINT('Ctrl Pts',(-29.8061310661599,8.37538791626452,135.70896232559));
#40628=CARTESIAN_POINT('Ctrl Pts',(-29.8734626000106,8.36988598131075,135.704221903287));
#40629=CARTESIAN_POINT('Ctrl Pts',(-29.8963182945236,8.36801834905373,135.702612766559));
#40630=CARTESIAN_POINT('Ctrl Pts',(-29.9191264886051,8.36662503132851,135.701446014514));
#40631=CARTESIAN_POINT('Ctrl Pts',(-29.9419585439552,8.36574539366428,135.70071174992));
#40632=CARTESIAN_POINT('Ctrl Pts',(-29.9529619128661,8.36532147310264,135.70035788847));
#40633=CARTESIAN_POINT('Ctrl Pts',(-29.963955947468,8.365017872708,135.700106267193));
#40634=CARTESIAN_POINT('Ctrl Pts',(-29.9749570822295,8.36483405979636,135.699953932128));
#40635=CARTESIAN_POINT('Ctrl Pts',(-30.0209171987356,8.36406613330358,135.699317512567));
#40636=CARTESIAN_POINT('Ctrl Pts',(-30.0667990439102,8.36546505443102,135.700441545656));
#40637=CARTESIAN_POINT('Ctrl Pts',(-30.1127851886818,8.36886140284237,135.703319027213));
#40638=CARTESIAN_POINT('Ctrl Pts',(-30.1465700186564,8.37135661208814,135.705433038415));
#40639=CARTESIAN_POINT('Ctrl Pts',(-30.180449969916,8.37490071039504,135.70857305589));
#40640=CARTESIAN_POINT('Ctrl Pts',(-30.2142551605804,8.37930108895793,135.712568730666));
#40641=CARTESIAN_POINT('Ctrl Pts',(-30.4121935701959,8.40506647934105,135.735964472415));
#40642=CARTESIAN_POINT('Ctrl Pts',(-30.618223774017,8.46017177748985,135.795991006846));
#40643=CARTESIAN_POINT('Ctrl Pts',(-30.8090649857056,8.48601923378611,135.891967734795));
#40644=CARTESIAN_POINT('Ctrl Pts',(-30.8726787229352,8.49463505255153,135.923959977444));
#40645=CARTESIAN_POINT('Ctrl Pts',(-30.9346047943722,8.5,135.95994668604));
#40646=CARTESIAN_POINT('Ctrl Pts',(-30.9949874371066,8.5,136.));
#40647=CARTESIAN_POINT('',(-28.8951880620293,8.5,136.078947368421));
#40648=CARTESIAN_POINT('Ctrl Pts',(-28.8951880620293,8.5,136.078947368421));
#40649=CARTESIAN_POINT('Ctrl Pts',(-28.9307900499921,8.5,136.051268237865));
#40650=CARTESIAN_POINT('Ctrl Pts',(-28.9674326867105,8.5,136.024927669793));
#40651=CARTESIAN_POINT('Ctrl Pts',(-29.0050125628934,8.5,136.));
#40652=CARTESIAN_POINT('Origin',(-30.,8.5,137.5));
#40653=CARTESIAN_POINT('Ctrl Pts',(-28.9499455367427,8.39129047171135,135.916983334517));
#40654=CARTESIAN_POINT('Ctrl Pts',(-28.9583427274828,8.39013445090615,135.911534549944));
#40655=CARTESIAN_POINT('Ctrl Pts',(-28.966772971137,8.38888029152069,135.906181580337));
#40656=CARTESIAN_POINT('Ctrl Pts',(-28.9867478988158,8.38570733772648,135.893774692507));
#40657=CARTESIAN_POINT('Ctrl Pts',(-28.9983001592736,8.38372057934384,135.886804200101));
#40658=CARTESIAN_POINT('Ctrl Pts',(-29.2030969044704,8.34597008112109,135.767178547826));
#40659=CARTESIAN_POINT('Ctrl Pts',(-29.4772754648992,8.24903543084451,135.680444681192));
#40660=CARTESIAN_POINT('Ctrl Pts',(-29.7775051143642,8.19662294325174,135.651344091606));
#40661=CARTESIAN_POINT('Ctrl Pts',(-29.8804218187696,8.1865934232616,135.645948287097));
#40662=CARTESIAN_POINT('Ctrl Pts',(-29.9066026001864,8.18468277370489,135.644958149235));
#40663=CARTESIAN_POINT('Ctrl Pts',(-29.945607880728,8.18289720095053,135.6440346745));
#40664=CARTESIAN_POINT('Ctrl Pts',(-29.9583002059055,8.18248038026162,135.643821210287));
#40665=CARTESIAN_POINT('Ctrl Pts',(-30.0241258793722,8.18117464424746,135.643151906577));
#40666=CARTESIAN_POINT('Ctrl Pts',(-30.0772899664358,8.18310206076612,135.644103777041));
#40667=CARTESIAN_POINT('Ctrl Pts',(-30.1685015966763,8.19115568892363,135.648342005986));
#40668=CARTESIAN_POINT('Ctrl Pts',(-30.2068474352435,8.19595429131145,135.651012005824));
#40669=CARTESIAN_POINT('Ctrl Pts',(-30.465694468065,8.23688803331381,135.674362854996));
#40670=CARTESIAN_POINT('Ctrl Pts',(-30.7462229722334,8.33190850945499,135.742786049171));
#40671=CARTESIAN_POINT('Ctrl Pts',(-30.9908315655339,8.38313739956722,135.87855467171));
#40672=CARTESIAN_POINT('Ctrl Pts',(-31.0500544632574,8.39129047171136,135.916983334517));
#40673=CARTESIAN_POINT('Ctrl Pts',(-28.9683012121262,8.4275269811409,135.944655556345));
#40674=CARTESIAN_POINT('Ctrl Pts',(-28.9767482458833,8.42675447068797,135.939129772415));
#40675=CARTESIAN_POINT('Ctrl Pts',(-28.9852428165901,8.4258854532691,135.933697780808));
#40676=CARTESIAN_POINT('Ctrl Pts',(-29.0053155369763,8.42359293603061,135.921096409854));
#40677=CARTESIAN_POINT('Ctrl Pts',(-29.0169595159405,8.42211931541817,135.914010922128));
#40678=CARTESIAN_POINT('Ctrl Pts',(-29.2225856050001,8.39302212150272,135.792260131076));
#40679=CARTESIAN_POINT('Ctrl Pts',(-29.4968121969792,8.30401382953196,135.701370817213));
#40680=CARTESIAN_POINT('Ctrl Pts',(-29.7870605852856,8.25623003142132,135.670553593888));
#40681=CARTESIAN_POINT('Ctrl Pts',(-29.88567998585,8.24706050714524,135.664841173047));
#40682=CARTESIAN_POINT('Ctrl Pts',(-29.9107585634698,8.24533390764406,135.663791948766));
#40683=CARTESIAN_POINT('Ctrl Pts',(-29.9480281814684,8.24370245708609,135.662813622199));
#40684=CARTESIAN_POINT('Ctrl Pts',(-29.9601594059379,8.24332623806954,135.662587713756));
#40685=CARTESIAN_POINT('Ctrl Pts',(-30.0230260928526,8.242135170428,135.661877452567));
#40686=CARTESIAN_POINT('Ctrl Pts',(-30.0737662618809,8.243894603273,135.662889336933));
#40687=CARTESIAN_POINT('Ctrl Pts',(-30.1611638741047,8.25121736432493,135.66737577025));
#40688=CARTESIAN_POINT('Ctrl Pts',(-30.1980240267559,8.25561494071651,135.670207472671));
#40689=CARTESIAN_POINT('Ctrl Pts',(-30.4478023473742,8.29287747645514,135.694882333825));
#40690=CARTESIAN_POINT('Ctrl Pts',(-30.7264868782781,8.38080329713428,135.767194847034));
#40691=CARTESIAN_POINT('Ctrl Pts',(-30.9720741462826,8.42207265865225,135.90569558041));
#40692=CARTESIAN_POINT('Ctrl Pts',(-31.0316987878738,8.4275269811409,135.944655556345));
#40693=CARTESIAN_POINT('Ctrl Pts',(-28.9866568875098,8.46376349057045,135.972327778172));
#40694=CARTESIAN_POINT('Ctrl Pts',(-28.9951686750096,8.46337998021818,135.966725634326));
#40695=CARTESIAN_POINT('Ctrl Pts',(-29.0036920314769,8.46288297234629,135.961213070326));
#40696=CARTESIAN_POINT('Ctrl Pts',(-29.0239180740316,8.46149122158308,135.948419567118));
#40697=CARTESIAN_POINT('Ctrl Pts',(-29.0355780851662,8.46050386249283,135.941215807522));
#40698=CARTESIAN_POINT('Ctrl Pts',(-29.2422723400444,8.44008395869115,135.817350883128));
#40699=CARTESIAN_POINT('Ctrl Pts',(-29.5164771026875,8.35907111401752,135.722284002996));
#40700=CARTESIAN_POINT('Ctrl Pts',(-29.7965755952385,8.31578082809494,135.689752823308));
#40701=CARTESIAN_POINT('Ctrl Pts',(-29.8910601274432,8.3075512651701,135.683719880609));
#40702=CARTESIAN_POINT('Ctrl Pts',(-29.9149705253217,8.30597389738934,135.682612214983));
#40703=CARTESIAN_POINT('Ctrl Pts',(-29.9505416121257,8.30451621696708,135.681578940771));
#40704=CARTESIAN_POINT('Ctrl Pts',(-29.9620967474356,8.30417201490008,135.681339763724));
#40705=CARTESIAN_POINT('Ctrl Pts',(-30.0220169852552,8.30310560712303,135.680591966577));
#40706=CARTESIAN_POINT('Ctrl Pts',(-30.0703227484652,8.30467251192415,135.681655985765));
#40707=CARTESIAN_POINT('Ctrl Pts',(-30.153907741228,8.31129493668684,135.686399274151));
#40708=CARTESIAN_POINT('Ctrl Pts',(-30.1892733784037,8.31524006098998,135.689377589043));
#40709=CARTESIAN_POINT('Ctrl Pts',(-30.4300856908867,8.34907703619973,135.715444993586));
#40710=CARTESIAN_POINT('Ctrl Pts',(-30.7066366025794,8.42964542252683,135.791591053794));
#40711=CARTESIAN_POINT('Ctrl Pts',(-30.9533622136235,8.46106474091497,135.93280577734));
#40712=CARTESIAN_POINT('Ctrl Pts',(-31.0133431124902,8.46376349057045,135.972327778172));
#40713=CARTESIAN_POINT('Ctrl Pts',(-29.0050125628934,8.5,136.));
#40714=CARTESIAN_POINT('Ctrl Pts',(-29.01357419341,8.5,135.994320856796));
#40715=CARTESIAN_POINT('Ctrl Pts',(-29.0221618769299,8.4998881340947,135.988729270797));
#40716=CARTESIAN_POINT('Ctrl Pts',(-29.0424857121922,8.49937681988721,135.975741284465));
#40717=CARTESIAN_POINT('Ctrl Pts',(-29.0542374418331,8.49890259856716,135.968422529549));
#40718=CARTESIAN_POINT('Ctrl Pts',(-29.2617610405741,8.48713599907278,135.842432466379));
#40719=CARTESIAN_POINT('Ctrl Pts',(-29.5360138347675,8.41404951270497,135.743210139017));
#40720=CARTESIAN_POINT('Ctrl Pts',(-29.8061310661599,8.37538791626452,135.70896232559));
#40721=CARTESIAN_POINT('Ctrl Pts',(-29.8963182945236,8.36801834905373,135.702612766559));
#40722=CARTESIAN_POINT('Ctrl Pts',(-29.9191264886051,8.36662503132851,135.701446014514));
#40723=CARTESIAN_POINT('Ctrl Pts',(-29.9529619128661,8.36532147310264,135.70035788847));
#40724=CARTESIAN_POINT('Ctrl Pts',(-29.963955947468,8.365017872708,135.700106267193));
#40725=CARTESIAN_POINT('Ctrl Pts',(-30.0209171987356,8.36406613330358,135.699317512567));
#40726=CARTESIAN_POINT('Ctrl Pts',(-30.0667990439102,8.36546505443102,135.700441545656));
#40727=CARTESIAN_POINT('Ctrl Pts',(-30.1465700186564,8.37135661208814,135.705433038415));
#40728=CARTESIAN_POINT('Ctrl Pts',(-30.180449969916,8.37490071039504,135.70857305589));
#40729=CARTESIAN_POINT('Ctrl Pts',(-30.4121935701959,8.40506647934105,135.735964472415));
#40730=CARTESIAN_POINT('Ctrl Pts',(-30.6869005086241,8.47854021020612,135.815999851657));
#40731=CARTESIAN_POINT('Ctrl Pts',(-30.9346047943722,8.5,135.95994668604));
#40732=CARTESIAN_POINT('Ctrl Pts',(-30.9949874371067,8.5,136.));
#40733=CARTESIAN_POINT('',(-28.9499455367427,8.39129047171135,135.916983334517));
#40734=CARTESIAN_POINT('',(-30.9949874371066,8.5,136.));
#40735=CARTESIAN_POINT('Origin',(-30.,8.45,137.5));
#40736=CARTESIAN_POINT('',(-31.1661903789691,8.4,136.));
#40737=CARTESIAN_POINT('',(-28.8951880620293,8.5,136.078947368421));
#40738=CARTESIAN_POINT('Ctrl Pts',(-31.0500544632573,8.39129047171135,135.916983334517));
#40739=CARTESIAN_POINT('Ctrl Pts',(-31.0899798051577,8.39678689632762,135.942890163806));
#40740=CARTESIAN_POINT('Ctrl Pts',(-31.1286105039774,8.40000000009859,135.970783140825));
#40741=CARTESIAN_POINT('Ctrl Pts',(-31.1661903807052,8.4,136.00000000135));
#40742=CARTESIAN_POINT('Ctrl Pts',(-31.0316987878738,8.4275269811409,135.944655556345));
#40743=CARTESIAN_POINT('Ctrl Pts',(-31.0708423080613,8.43119126421841,135.970235999263));
#40744=CARTESIAN_POINT('Ctrl Pts',(-31.1088103196971,8.43333333339906,135.997611506775));
#40745=CARTESIAN_POINT('Ctrl Pts',(-31.145730900342,8.43333333333333,136.0263157908));
#40746=CARTESIAN_POINT('Ctrl Pts',(-31.0133431124902,8.46376349057045,135.972327778172));
#40747=CARTESIAN_POINT('Ctrl Pts',(-31.0517048109648,8.46559563210921,135.99758183472));
#40748=CARTESIAN_POINT('Ctrl Pts',(-31.0890101354168,8.46666666669953,136.024439872726));
#40749=CARTESIAN_POINT('Ctrl Pts',(-31.1252714199787,8.46666666666667,136.05263158025));
#40750=CARTESIAN_POINT('Ctrl Pts',(-30.9949874371066,8.5,136.));
#40751=CARTESIAN_POINT('Ctrl Pts',(-31.0325673138683,8.5,136.024927670177));
#40752=CARTESIAN_POINT('Ctrl Pts',(-31.0692099511365,8.5,136.051268238676));
#40753=CARTESIAN_POINT('Ctrl Pts',(-31.1048119396155,8.5,136.0789473697));
#40754=CARTESIAN_POINT('Ctrl Pts',(-28.833809621031,8.4,136.));
#40755=CARTESIAN_POINT('Ctrl Pts',(-28.8713894972139,8.4,135.970783139968));
#40756=CARTESIAN_POINT('Ctrl Pts',(-28.9100201954571,8.39678689624297,135.942890163407));
#40757=CARTESIAN_POINT('Ctrl Pts',(-28.9499455367427,8.39129047171135,135.916983334517));
#40758=CARTESIAN_POINT('Ctrl Pts',(-28.8542691013637,8.43333333333333,136.026315789474));
#40759=CARTESIAN_POINT('Ctrl Pts',(-28.8911896814733,8.43333333333333,135.997611505934));
#40760=CARTESIAN_POINT('Ctrl Pts',(-28.9291576925416,8.43119126416198,135.970235998869));
#40761=CARTESIAN_POINT('Ctrl Pts',(-28.9683012121263,8.4275269811409,135.944655556345));
#40762=CARTESIAN_POINT('Ctrl Pts',(-28.8747285816965,8.46666666666667,136.052631578947));
#40763=CARTESIAN_POINT('Ctrl Pts',(-28.9109898657327,8.46666666666667,136.024439871899));
#40764=CARTESIAN_POINT('Ctrl Pts',(-28.948295189626,8.46559563208099,135.997581834331));
#40765=CARTESIAN_POINT('Ctrl Pts',(-28.9866568875098,8.46376349057045,135.972327778172));
#40766=CARTESIAN_POINT('Ctrl Pts',(-28.8951880620293,8.5,136.078947368421));
#40767=CARTESIAN_POINT('Ctrl Pts',(-28.9307900499921,8.5,136.051268237865));
#40768=CARTESIAN_POINT('Ctrl Pts',(-28.9674326867105,8.5,136.024927669793));
#40769=CARTESIAN_POINT('Ctrl Pts',(-29.0050125628934,8.5,136.));
#40770=CARTESIAN_POINT('Ctrl Pts',(-29.37557606376,8.99442305443429,144.29429745799));
#40771=CARTESIAN_POINT('Ctrl Pts',(-29.3968663992163,8.99354972599348,144.301654944207));
#40772=CARTESIAN_POINT('Ctrl Pts',(-29.4183017778428,8.99262938553082,144.308615224025));
#40773=CARTESIAN_POINT('Ctrl Pts',(-29.5879618888624,8.98495073555583,144.36060019061));
#40774=CARTESIAN_POINT('Ctrl Pts',(-29.8570704543082,8.97294630891696,144.405692333025));
#40775=CARTESIAN_POINT('Ctrl Pts',(-30.1448589551985,8.97549033242365,144.39734513884));
#40776=CARTESIAN_POINT('Ctrl Pts',(-30.3737546351539,8.98306099714656,144.364880756376));
#40777=CARTESIAN_POINT('Ctrl Pts',(-30.4860772057434,8.98837707594693,144.337802199667));
#40778=CARTESIAN_POINT('Ctrl Pts',(-30.5816983343123,8.99261835182926,144.308632644433));
#40779=CARTESIAN_POINT('Ctrl Pts',(-30.6031336007837,8.99354972599348,144.301654944207));
#40780=CARTESIAN_POINT('Ctrl Pts',(-30.62442393624,8.99442305443429,144.29429745799));
#40781=CARTESIAN_POINT('Ctrl Pts',(-29.3865147164033,8.96294870295619,144.262864971993));
#40782=CARTESIAN_POINT('Ctrl Pts',(-29.4073401763186,8.96237080371183,144.270080554424));
#40783=CARTESIAN_POINT('Ctrl Pts',(-29.4283245709687,8.96172080327479,144.276909137492));
#40784=CARTESIAN_POINT('Ctrl Pts',(-29.594500212573,8.95618570956421,144.328046949343));
#40785=CARTESIAN_POINT('Ctrl Pts',(-29.8591950711281,8.94617889889013,144.372922700884));
#40786=CARTESIAN_POINT('Ctrl Pts',(-30.1426748215025,8.9483374189058,144.364588161718));
#40787=CARTESIAN_POINT('Ctrl Pts',(-30.3677623300152,8.95450008198494,144.332371964081));
#40788=CARTESIAN_POINT('Ctrl Pts',(-30.4780285068212,8.95865448574558,144.305612529178));
#40789=CARTESIAN_POINT('Ctrl Pts',(-30.5716737135296,8.96171637278058,144.276928607877));
#40790=CARTESIAN_POINT('Ctrl Pts',(-30.5926609072949,8.96236576597913,144.270078935029));
#40791=CARTESIAN_POINT('Ctrl Pts',(-30.6134852835967,8.96294870295619,144.262864971993));
#40792=CARTESIAN_POINT('Ctrl Pts',(-29.3974533690467,8.9314743514781,144.231432485996));
#40793=CARTESIAN_POINT('Ctrl Pts',(-29.4178165235133,8.93117892228165,144.238499084234));
#40794=CARTESIAN_POINT('Ctrl Pts',(-29.4383449914353,8.93082558456286,144.245210604997));
#40795=CARTESIAN_POINT('Ctrl Pts',(-29.6010478149954,8.92735264779638,144.295449195762));
#40796=CARTESIAN_POINT('Ctrl Pts',(-29.861341108549,8.91940129063077,144.340159362869));
#40797=CARTESIAN_POINT('Ctrl Pts',(-30.1404741111915,8.92117778746871,144.331810860123));
#40798=CARTESIAN_POINT('Ctrl Pts',(-30.3617899054628,8.9259156506157,144.299860032397));
#40799=CARTESIAN_POINT('Ctrl Pts',(-30.4699427746209,8.92894383621034,144.273406936258));
#40800=CARTESIAN_POINT('Ctrl Pts',(-30.5616573345954,8.93081126954196,144.245227705831));
#40801=CARTESIAN_POINT('Ctrl Pts',(-30.5821823928732,8.93118396001435,144.238500703629));
#40802=CARTESIAN_POINT('Ctrl Pts',(-30.6025466309533,8.9314743514781,144.231432485997));
#40803=CARTESIAN_POINT('Ctrl Pts',(-29.40839202169,8.9,144.2));
#40804=CARTESIAN_POINT('Ctrl Pts',(-29.4282903006156,8.9,144.206924694451));
#40805=CARTESIAN_POINT('Ctrl Pts',(-29.4483677845611,8.89991700230683,144.213504518463));
#40806=CARTESIAN_POINT('Ctrl Pts',(-29.607586138706,8.89858762180476,144.262895954495));
#40807=CARTESIAN_POINT('Ctrl Pts',(-29.8634657253689,8.89263388060395,144.307389730728));
#40808=CARTESIAN_POINT('Ctrl Pts',(-30.1382899774955,8.89402487395086,144.299053883001));
#40809=CARTESIAN_POINT('Ctrl Pts',(-30.3557976003241,8.89735473545407,144.267351240102));
#40810=CARTESIAN_POINT('Ctrl Pts',(-30.4618940756987,8.899221246009,144.241217265769));
#40811=CARTESIAN_POINT('Ctrl Pts',(-30.5516327138128,8.89990929049328,144.213523669276));
#40812=CARTESIAN_POINT('Ctrl Pts',(-30.5717096993844,8.9,144.206924694451));
#40813=CARTESIAN_POINT('Ctrl Pts',(-30.59160797831,8.9,144.2));
#40814=CARTESIAN_POINT('',(-30.59160797831,8.9,144.2));
#40815=CARTESIAN_POINT('',(-30.59160797831,8.9,144.2));
#40816=CARTESIAN_POINT('',(-29.40839202169,8.9,144.2));
#40817=CARTESIAN_POINT('',(-29.37557606376,8.99442305443429,144.29429745799));
#40818=CARTESIAN_POINT('Ctrl Pts',(-29.40839202169,8.9,144.2));
#40819=CARTESIAN_POINT('Ctrl Pts',(-29.4282903006156,8.9,144.206924694451));
#40820=CARTESIAN_POINT('Ctrl Pts',(-29.4483677845611,8.89991700230683,144.213504518463));
#40821=CARTESIAN_POINT('Ctrl Pts',(-29.607586138706,8.89858762180476,144.262895954495));
#40822=CARTESIAN_POINT('Ctrl Pts',(-29.8634657253689,8.89263388060395,144.307389730728));
#40823=CARTESIAN_POINT('Ctrl Pts',(-30.1382899774955,8.89402487395086,144.299053883001));
#40824=CARTESIAN_POINT('Ctrl Pts',(-30.3557976003241,8.89735473545407,144.267351240102));
#40825=CARTESIAN_POINT('Ctrl Pts',(-30.4618940756987,8.899221246009,144.241217265769));
#40826=CARTESIAN_POINT('Ctrl Pts',(-30.5516327138128,8.89990929049328,144.213523669276));
#40827=CARTESIAN_POINT('Ctrl Pts',(-30.5717096993844,8.9,144.206924694451));
#40828=CARTESIAN_POINT('Ctrl Pts',(-30.59160797831,8.9,144.2));
#40829=CARTESIAN_POINT('Origin',(-30.,8.95,142.5));
#40830=CARTESIAN_POINT('',(-30.80386876177,8.9,144.110526315789));
#40831=CARTESIAN_POINT('',(-30.8485281374239,9.,144.2));
#40832=CARTESIAN_POINT('',(-31.8,8.9,142.5));
#40833=CARTESIAN_POINT('Origin',(-30.,8.9,142.5));
#40834=CARTESIAN_POINT('',(-29.19613123823,8.9,144.110526315789));
#40835=CARTESIAN_POINT('Origin',(-30.,8.9,142.5));
#40836=CARTESIAN_POINT('',(-29.19613123823,8.9,144.110526315789));
#40837=CARTESIAN_POINT('Ctrl Pts',(-30.62442393624,8.99442305443429,144.29429745799));
#40838=CARTESIAN_POINT('Ctrl Pts',(-30.7010733797632,8.99756721057681,144.267809043778));
#40839=CARTESIAN_POINT('Ctrl Pts',(-30.7759616147075,9.00000000000003,144.236220433153));
#40840=CARTESIAN_POINT('Ctrl Pts',(-30.8485281374251,9.,144.199999999999));
#40841=CARTESIAN_POINT('Ctrl Pts',(-30.6134852835967,8.96294870295619,144.262864971993));
#40842=CARTESIAN_POINT('Ctrl Pts',(-30.688773753518,8.96504480705121,144.236788199029));
#40843=CARTESIAN_POINT('Ctrl Pts',(-30.762348253046,8.96666666666669,144.205760425554));
#40844=CARTESIAN_POINT('Ctrl Pts',(-30.8336416788738,8.96666666666667,144.170175438596));
#40845=CARTESIAN_POINT('Ctrl Pts',(-30.6025466309533,8.9314743514781,144.231432485997));
#40846=CARTESIAN_POINT('Ctrl Pts',(-30.6764741272728,8.9325224035256,144.20576735428));
#40847=CARTESIAN_POINT('Ctrl Pts',(-30.7487348913845,8.93333333333334,144.175300417955));
#40848=CARTESIAN_POINT('Ctrl Pts',(-30.8187552203225,8.93333333333333,144.140350877192));
#40849=CARTESIAN_POINT('Ctrl Pts',(-30.59160797831,8.9,144.2));
#40850=CARTESIAN_POINT('Ctrl Pts',(-30.6641745010276,8.9,144.174746509531));
#40851=CARTESIAN_POINT('Ctrl Pts',(-30.7351215297229,8.9,144.144840410355));
#40852=CARTESIAN_POINT('Ctrl Pts',(-30.8038687617712,8.9,144.110526315789));
#40853=CARTESIAN_POINT('Ctrl Pts',(-30.59160797831,8.9,144.2));
#40854=CARTESIAN_POINT('Ctrl Pts',(-30.6641745010276,8.9,144.174746509531));
#40855=CARTESIAN_POINT('Ctrl Pts',(-30.7351215297229,8.9,144.144840410355));
#40856=CARTESIAN_POINT('Ctrl Pts',(-30.8038687617712,8.9,144.110526315789));
#40857=CARTESIAN_POINT('Ctrl Pts',(-29.1514718625761,9.,144.2));
#40858=CARTESIAN_POINT('Ctrl Pts',(-29.2240383852933,9.,144.236220433153));
#40859=CARTESIAN_POINT('Ctrl Pts',(-29.2989266202372,8.99756721057679,144.267809043778));
#40860=CARTESIAN_POINT('Ctrl Pts',(-29.37557606376,8.99442305443429,144.29429745799));
#40861=CARTESIAN_POINT('Ctrl Pts',(-29.1663583211274,8.96666666666667,144.170175438596));
#40862=CARTESIAN_POINT('Ctrl Pts',(-29.2376517469549,8.96666666666667,144.205760425554));
#40863=CARTESIAN_POINT('Ctrl Pts',(-29.3112262464824,8.96504480705119,144.236788199029));
#40864=CARTESIAN_POINT('Ctrl Pts',(-29.3865147164034,8.96294870295619,144.262864971993));
#40865=CARTESIAN_POINT('Ctrl Pts',(-29.1812447796787,8.93333333333333,144.140350877193));
#40866=CARTESIAN_POINT('Ctrl Pts',(-29.2512651086164,8.93333333333333,144.175300417955));
#40867=CARTESIAN_POINT('Ctrl Pts',(-29.3235258727276,8.9325224035256,144.20576735428));
#40868=CARTESIAN_POINT('Ctrl Pts',(-29.3974533690467,8.9314743514781,144.231432485997));
#40869=CARTESIAN_POINT('Ctrl Pts',(-29.19613123823,8.9,144.110526315789));
#40870=CARTESIAN_POINT('Ctrl Pts',(-29.2648784702779,8.9,144.144840410356));
#40871=CARTESIAN_POINT('Ctrl Pts',(-29.3358254989728,8.9,144.174746509531));
#40872=CARTESIAN_POINT('Ctrl Pts',(-29.40839202169,8.9,144.2));
#40873=CARTESIAN_POINT('Ctrl Pts',(-29.19613123823,8.9,144.110526315789));
#40874=CARTESIAN_POINT('Ctrl Pts',(-29.2648784702779,8.9,144.144840410356));
#40875=CARTESIAN_POINT('Ctrl Pts',(-29.3358254989728,8.9,144.174746509531));
#40876=CARTESIAN_POINT('Ctrl Pts',(-29.40839202169,8.9,144.2));
#40877=CARTESIAN_POINT('Origin',(-30.,9.1,142.5));
#40878=CARTESIAN_POINT('',(-31.8,8.5,142.5));
#40879=CARTESIAN_POINT('',(-31.8,9.1,142.5));
#40880=CARTESIAN_POINT('',(-28.8951880620293,8.5,143.921052631579));
#40881=CARTESIAN_POINT('Origin',(-30.,8.5,142.5));
#40882=CARTESIAN_POINT('',(-29.0050125628934,8.5,144.));
#40883=CARTESIAN_POINT('Ctrl Pts',(-29.0050125628934,8.5,144.));
#40884=CARTESIAN_POINT('Ctrl Pts',(-28.9674326867105,8.5,143.975072330207));
#40885=CARTESIAN_POINT('Ctrl Pts',(-28.9307900499921,8.5,143.948731762135));
#40886=CARTESIAN_POINT('Ctrl Pts',(-28.8951880620293,8.5,143.921052631579));
#40887=CARTESIAN_POINT('',(-30.9949874371066,8.5,144.));
#40888=CARTESIAN_POINT('Ctrl Pts',(-30.9949874371066,8.49999999999999,144.));
#40889=CARTESIAN_POINT('Ctrl Pts',(-30.9864258065899,8.49999999999999,144.005679143204));
#40890=CARTESIAN_POINT('Ctrl Pts',(-30.9778386719318,8.49988852054169,144.011270754062));
#40891=CARTESIAN_POINT('Ctrl Pts',(-30.9692250597263,8.49967146108473,144.016774507783));
#40892=CARTESIAN_POINT('Ctrl Pts',(-30.9575123233977,8.49937630498455,144.024258477877));
#40893=CARTESIAN_POINT('Ctrl Pts',(-30.9457720398319,8.49890718075588,144.031578258464));
#40894=CARTESIAN_POINT('Ctrl Pts',(-30.9339557366539,8.49823143451159,144.038740897101));
#40895=CARTESIAN_POINT('Ctrl Pts',(-30.6726388899699,8.48328734624167,144.197142227399));
#40896=CARTESIAN_POINT('Ctrl Pts',(-30.3955689407068,8.39161125939828,144.276735792559));
#40897=CARTESIAN_POINT('Ctrl Pts',(-30.1265319331592,8.36984745763126,144.295772364356));
#40898=CARTESIAN_POINT('Ctrl Pts',(-30.1037007747645,8.36800052657168,144.297387855808));
#40899=CARTESIAN_POINT('Ctrl Pts',(-30.0808712194313,8.36659012091945,144.298549094101));
#40900=CARTESIAN_POINT('Ctrl Pts',(-30.0580431077713,8.36571381605628,144.299284047477));
#40901=CARTESIAN_POINT('Ctrl Pts',(-30.0470416394284,8.36529150165926,144.299638240868));
#40902=CARTESIAN_POINT('Ctrl Pts',(-30.036044636314,8.36498601410341,144.299889873607));
#40903=CARTESIAN_POINT('Ctrl Pts',(-30.0250454942028,8.36480330495199,144.300041744189));
#40904=CARTESIAN_POINT('Ctrl Pts',(-30.0035042967233,8.36444547941686,144.300339174131));
#40905=CARTESIAN_POINT('Ctrl Pts',(-29.9819683006895,8.36455538212952,144.30024955842));
#40906=CARTESIAN_POINT('Ctrl Pts',(-29.9604261249166,8.36513079602048,144.299774357394));
#40907=CARTESIAN_POINT('Ctrl Pts',(-29.9360144221004,8.36578285795937,144.299235857181));
#40908=CARTESIAN_POINT('Ctrl Pts',(-29.9116476872554,8.36702849219147,144.298196931516));
#40909=CARTESIAN_POINT('Ctrl Pts',(-29.8872073846878,8.36883152973277,144.29666716382));
#40910=CARTESIAN_POINT('Ctrl Pts',(-29.8534067066909,8.37132511143786,144.294551511398));
#40911=CARTESIAN_POINT('Ctrl Pts',(-29.8195400563255,8.37487055555119,144.291412849903));
#40912=CARTESIAN_POINT('Ctrl Pts',(-29.7857330314176,8.3792716381878,144.287417383752));
#40913=CARTESIAN_POINT('Ctrl Pts',(-29.5877838818172,8.40504115111046,144.264022863562));
#40914=CARTESIAN_POINT('Ctrl Pts',(-29.3817727081634,8.46016437071621,144.204005312567));
#40915=CARTESIAN_POINT('Ctrl Pts',(-29.1909346646337,8.48601711341369,144.108031216413));
#40916=CARTESIAN_POINT('Ctrl Pts',(-29.1273219834571,8.49463469431285,144.076039851029));
#40917=CARTESIAN_POINT('Ctrl Pts',(-29.0653952056277,8.49999999999999,144.04005331396));
#40918=CARTESIAN_POINT('Ctrl Pts',(-29.0050125628934,8.49999999999999,144.));
#40919=CARTESIAN_POINT('',(-31.1048119379707,8.5,143.921052631579));
#40920=CARTESIAN_POINT('Ctrl Pts',(-31.1048119379707,8.5,143.921052631579));
#40921=CARTESIAN_POINT('Ctrl Pts',(-31.0692099500079,8.5,143.948731762135));
#40922=CARTESIAN_POINT('Ctrl Pts',(-31.0325673132895,8.5,143.975072330207));
#40923=CARTESIAN_POINT('Ctrl Pts',(-30.9949874371066,8.5,144.));
#40924=CARTESIAN_POINT('Origin',(-30.,8.5,142.5));
#40925=CARTESIAN_POINT('Ctrl Pts',(-31.0500544632573,8.39129047171135,144.083016665483));
#40926=CARTESIAN_POINT('Ctrl Pts',(-31.0416572725172,8.39013445090615,144.088465450056));
#40927=CARTESIAN_POINT('Ctrl Pts',(-31.0332270809276,8.38887970921002,144.093818628959));
#40928=CARTESIAN_POINT('Ctrl Pts',(-31.0132516281393,8.38570812580638,144.106224780502));
#40929=CARTESIAN_POINT('Ctrl Pts',(-31.0017014315445,8.38371364530919,144.113198879946));
#40930=CARTESIAN_POINT('Ctrl Pts',(-30.7324511236407,8.33432880803088,144.270318781487));
#40931=CARTESIAN_POINT('Ctrl Pts',(-30.4529311916243,8.21959507258029,144.336354071163));
#40932=CARTESIAN_POINT('Ctrl Pts',(-30.1195807496158,8.18661062269483,144.354047747419));
#40933=CARTESIAN_POINT('Ctrl Pts',(-30.0933941115233,8.18473112770877,144.355023956059));
#40934=CARTESIAN_POINT('Ctrl Pts',(-30.0543910542229,8.18293757017519,144.355950759946));
#40935=CARTESIAN_POINT('Ctrl Pts',(-30.0416959390612,8.18252195324135,144.35616358648));
#40936=CARTESIAN_POINT('Ctrl Pts',(-30.0040933217041,8.18177796546578,144.356545242999));
#40937=CARTESIAN_POINT('Ctrl Pts',(-29.9791722273264,8.18192966483189,144.356469222117));
#40938=CARTESIAN_POINT('Ctrl Pts',(-29.9261171052882,8.18361364393076,144.355609595774));
#40939=CARTESIAN_POINT('Ctrl Pts',(-29.8980661716417,8.18531958471388,144.354728185553));
#40940=CARTESIAN_POINT('Ctrl Pts',(-29.8314696713767,8.19118993782772,144.351632857542));
#40941=CARTESIAN_POINT('Ctrl Pts',(-29.7931403426605,8.19599191204271,144.348964017633));
#40942=CARTESIAN_POINT('Ctrl Pts',(-29.5342776523695,8.23691405320499,144.32561688535));
#40943=CARTESIAN_POINT('Ctrl Pts',(-29.2537806211792,8.33191174571249,144.257212629307));
#40944=CARTESIAN_POINT('Ctrl Pts',(-29.009168434466,8.38313739956723,144.121445328289));
#40945=CARTESIAN_POINT('Ctrl Pts',(-28.9499455367427,8.39129047171135,144.083016665483));
#40946=CARTESIAN_POINT('Ctrl Pts',(-31.0316987878738,8.4275269811409,144.055344443655));
#40947=CARTESIAN_POINT('Ctrl Pts',(-31.0232494782234,8.42674758136909,144.060871364535));
#40948=CARTESIAN_POINT('Ctrl Pts',(-31.0147604421638,8.4258945773603,144.066300826652));
#40949=CARTESIAN_POINT('Ctrl Pts',(-30.9946783468982,8.42357664552238,144.078905881521));
#40950=CARTESIAN_POINT('Ctrl Pts',(-30.9830491673224,8.42213380515014,144.085988624004));
#40951=CARTESIAN_POINT('Ctrl Pts',(-30.7126406025825,8.38391948813827,144.245935181324));
#40952=CARTESIAN_POINT('Ctrl Pts',(-30.4335871468451,8.27667769995428,144.316530411117));
#40953=CARTESIAN_POINT('Ctrl Pts',(-30.1143332642689,8.24713075999365,144.335146729607));
#40954=CARTESIAN_POINT('Ctrl Pts',(-30.0892321163076,8.24534698733409,144.336195530571));
#40955=CARTESIAN_POINT('Ctrl Pts',(-30.0519728840255,8.24375611845358,144.337169744628));
#40956=CARTESIAN_POINT('Ctrl Pts',(-30.03983621471,8.24336276859699,144.337398013963));
#40957=CARTESIAN_POINT('Ctrl Pts',(-30.0039249294193,8.24269311190836,144.337801203055));
#40958=CARTESIAN_POINT('Ctrl Pts',(-29.9801292530066,8.24282792333394,144.33772086074));
#40959=CARTESIAN_POINT('Ctrl Pts',(-29.9294428595935,8.24435853719646,144.33681052603));
#40960=CARTESIAN_POINT('Ctrl Pts',(-29.902618367519,8.24591603275185,144.335874860442));
#40961=CARTESIAN_POINT('Ctrl Pts',(-29.8388088722218,8.25125052269469,144.332599609949));
#40962=CARTESIAN_POINT('Ctrl Pts',(-29.8019634018542,8.25565283346855,144.329768423253));
#40963=CARTESIAN_POINT('Ctrl Pts',(-29.5521701639099,8.29290319017188,144.305097549906));
#40964=CARTESIAN_POINT('Ctrl Pts',(-29.2735164712547,8.3808067246845,144.232803741881));
#40965=CARTESIAN_POINT('Ctrl Pts',(-29.0279259249285,8.42207260275014,144.094304445759));
#40966=CARTESIAN_POINT('Ctrl Pts',(-28.9683012121263,8.4275269811409,144.055344443655));
#40967=CARTESIAN_POINT('Ctrl Pts',(-31.0133431124902,8.46376349057045,144.027672221828));
#40968=CARTESIAN_POINT('Ctrl Pts',(-31.0048336008837,8.46338686953705,144.033273228725));
#40969=CARTESIAN_POINT('Ctrl Pts',(-30.9963053106956,8.46287365239142,144.038788556369));
#40970=CARTESIAN_POINT('Ctrl Pts',(-30.9760856046388,8.46150778526856,144.051577376858));
#40971=CARTESIAN_POINT('Ctrl Pts',(-30.964424304054,8.46048702091494,144.058788514405));
#40972=CARTESIAN_POINT('Ctrl Pts',(-30.6924494110281,8.43369666613429,144.221525827561));
#40973=CARTESIAN_POINT('Ctrl Pts',(-30.4149129854861,8.33452863202431,144.296559452605));
#40974=CARTESIAN_POINT('Ctrl Pts',(-30.1089482601113,8.30748038927288,144.316288873621));
#40975=CARTESIAN_POINT('Ctrl Pts',(-30.085033214647,8.30597426129415,144.317377519589));
#40976=CARTESIAN_POINT('Ctrl Pts',(-30.0494598096259,8.30447295338088,144.318419256187));
#40977=CARTESIAN_POINT('Ctrl Pts',(-30.0379043606653,8.30414519874779,144.318655446124));
#40978=CARTESIAN_POINT('Ctrl Pts',(-30.0036726890082,8.3035303329743,144.319083214075));
#40979=CARTESIAN_POINT('Ctrl Pts',(-29.9810112750093,8.3036571236275,144.318997919797));
#40980=CARTESIAN_POINT('Ctrl Pts',(-29.9326886677951,8.30503796469369,144.318034926925));
#40981=CARTESIAN_POINT('Ctrl Pts',(-29.9070954913782,8.30643204415352,144.317050256628));
#40982=CARTESIAN_POINT('Ctrl Pts',(-29.8460675058458,8.31126452657091,144.31358475899));
#40983=CARTESIAN_POINT('Ctrl Pts',(-29.8107169971318,8.31520963412536,144.310608444283));
#40984=CARTESIAN_POINT('Ctrl Pts',(-29.5698913702768,8.34905201414359,144.284542199006));
#40985=CARTESIAN_POINT('Ctrl Pts',(-29.29336646687,8.42964379827947,144.208408349661));
#40986=CARTESIAN_POINT('Ctrl Pts',(-29.0466377151652,8.46106479681709,144.067194196491));
#40987=CARTESIAN_POINT('Ctrl Pts',(-28.9866568875098,8.46376349057045,144.027672221828));
#40988=CARTESIAN_POINT('Ctrl Pts',(-30.9949874371066,8.5,144.));
#40989=CARTESIAN_POINT('Ctrl Pts',(-30.9864258065899,8.5,144.005679143204));
#40990=CARTESIAN_POINT('Ctrl Pts',(-30.9778386719318,8.49988852054171,144.011270754062));
#40991=CARTESIAN_POINT('Ctrl Pts',(-30.9575123233977,8.49937630498457,144.024258477877));
#40992=CARTESIAN_POINT('Ctrl Pts',(-30.9457720398319,8.49890718075589,144.031578258464));
#40993=CARTESIAN_POINT('Ctrl Pts',(-30.6726388899699,8.48328734624168,144.197142227399));
#40994=CARTESIAN_POINT('Ctrl Pts',(-30.3955689407068,8.3916112593983,144.276735792559));
#40995=CARTESIAN_POINT('Ctrl Pts',(-30.1037007747645,8.3680005265717,144.297387855808));
#40996=CARTESIAN_POINT('Ctrl Pts',(-30.0808712194313,8.36659012091947,144.298549094101));
#40997=CARTESIAN_POINT('Ctrl Pts',(-30.0470416394284,8.36529150165928,144.299638240868));
#40998=CARTESIAN_POINT('Ctrl Pts',(-30.036044636314,8.36498601410343,144.299889873607));
#40999=CARTESIAN_POINT('Ctrl Pts',(-30.0035042967233,8.36444547941688,144.300339174131));
#41000=CARTESIAN_POINT('Ctrl Pts',(-29.9819683006895,8.36455538212954,144.30024955842));
#41001=CARTESIAN_POINT('Ctrl Pts',(-29.9360144221004,8.36578285795938,144.299235857181));
#41002=CARTESIAN_POINT('Ctrl Pts',(-29.9116476872554,8.36702849219149,144.298196931516));
#41003=CARTESIAN_POINT('Ctrl Pts',(-29.8534067066909,8.37132511143788,144.294551511398));
#41004=CARTESIAN_POINT('Ctrl Pts',(-29.8195400563255,8.3748705555512,144.291412849903));
#41005=CARTESIAN_POINT('Ctrl Pts',(-29.5877838818172,8.40504115111048,144.264022863562));
#41006=CARTESIAN_POINT('Ctrl Pts',(-29.3131023169455,8.47853877725148,144.183999462235));
#41007=CARTESIAN_POINT('Ctrl Pts',(-29.0653952056277,8.5,144.04005331396));
#41008=CARTESIAN_POINT('Ctrl Pts',(-29.0050125628934,8.5,144.));
#41009=CARTESIAN_POINT('',(-31.0500544632573,8.39129047171135,144.083016665483));
#41010=CARTESIAN_POINT('',(-29.0050125628934,8.5,144.));
#41011=CARTESIAN_POINT('Origin',(-30.,8.45,142.5));
#41012=CARTESIAN_POINT('',(-28.8338096210309,8.4,144.));
#41013=CARTESIAN_POINT('',(-31.1048119379707,8.5,143.921052631579));
#41014=CARTESIAN_POINT('Ctrl Pts',(-28.9499455367427,8.39129047171135,144.083016665483));
#41015=CARTESIAN_POINT('Ctrl Pts',(-28.9100201948423,8.39678689632762,144.057109836194));
#41016=CARTESIAN_POINT('Ctrl Pts',(-28.8713894960226,8.40000000009859,144.029216859175));
#41017=CARTESIAN_POINT('Ctrl Pts',(-28.8338096192947,8.4,143.99999999865));
#41018=CARTESIAN_POINT('Ctrl Pts',(-28.9683012121262,8.4275269811409,144.055344443655));
#41019=CARTESIAN_POINT('Ctrl Pts',(-28.9291576919387,8.43119126421841,144.029764000737));
#41020=CARTESIAN_POINT('Ctrl Pts',(-28.8911896803029,8.43333333339906,144.002388493225));
#41021=CARTESIAN_POINT('Ctrl Pts',(-28.854269099658,8.43333333333333,143.9736842092));
#41022=CARTESIAN_POINT('Ctrl Pts',(-28.9866568875098,8.46376349057045,144.027672221828));
#41023=CARTESIAN_POINT('Ctrl Pts',(-28.9482951890352,8.46559563210921,144.00241816528));
#41024=CARTESIAN_POINT('Ctrl Pts',(-28.9109898645832,8.46666666669953,143.975560127274));
#41025=CARTESIAN_POINT('Ctrl Pts',(-28.8747285800212,8.46666666666667,143.94736841975));
#41026=CARTESIAN_POINT('Ctrl Pts',(-29.0050125628934,8.5,144.));
#41027=CARTESIAN_POINT('Ctrl Pts',(-28.9674326861317,8.5,143.975072329823));
#41028=CARTESIAN_POINT('Ctrl Pts',(-28.9307900488635,8.5,143.948731761324));
#41029=CARTESIAN_POINT('Ctrl Pts',(-28.8951880603845,8.5,143.9210526303));
#41030=CARTESIAN_POINT('Ctrl Pts',(-31.166190378969,8.4,144.));
#41031=CARTESIAN_POINT('Ctrl Pts',(-31.1286105027861,8.4,144.029216860032));
#41032=CARTESIAN_POINT('Ctrl Pts',(-31.0899798045429,8.39678689624297,144.057109836593));
#41033=CARTESIAN_POINT('Ctrl Pts',(-31.0500544632573,8.39129047171135,144.083016665483));
#41034=CARTESIAN_POINT('Ctrl Pts',(-31.1457308986363,8.43333333333333,143.973684210526));
#41035=CARTESIAN_POINT('Ctrl Pts',(-31.1088103185267,8.43333333333333,144.002388494066));
#41036=CARTESIAN_POINT('Ctrl Pts',(-31.0708423074584,8.43119126416198,144.029764001131));
#41037=CARTESIAN_POINT('Ctrl Pts',(-31.0316987878737,8.4275269811409,144.055344443655));
#41038=CARTESIAN_POINT('Ctrl Pts',(-31.1252714183035,8.46666666666667,143.947368421053));
#41039=CARTESIAN_POINT('Ctrl Pts',(-31.0890101342673,8.46666666666667,143.975560128101));
#41040=CARTESIAN_POINT('Ctrl Pts',(-31.051704810374,8.46559563208099,144.002418165669));
#41041=CARTESIAN_POINT('Ctrl Pts',(-31.0133431124902,8.46376349057045,144.027672221828));
#41042=CARTESIAN_POINT('Ctrl Pts',(-31.1048119379707,8.5,143.921052631579));
#41043=CARTESIAN_POINT('Ctrl Pts',(-31.0692099500079,8.5,143.948731762135));
#41044=CARTESIAN_POINT('Ctrl Pts',(-31.0325673132895,8.5,143.975072330207));
#41045=CARTESIAN_POINT('Ctrl Pts',(-30.9949874371066,8.5,144.));
#41046=CARTESIAN_POINT('Origin',(30.,8.95,137.5));
#41047=CARTESIAN_POINT('',(30.80386876177,8.9,135.889473684211));
#41048=CARTESIAN_POINT('',(30.8485281374239,9.,135.8));
#41049=CARTESIAN_POINT('',(28.2,8.9,137.5));
#41050=CARTESIAN_POINT('Origin',(30.,8.9,137.5));
#41051=CARTESIAN_POINT('',(29.19613123823,8.9,135.889473684211));
#41052=CARTESIAN_POINT('Origin',(30.,8.9,137.5));
#41053=CARTESIAN_POINT('',(29.19613123823,8.9,135.889473684211));
#41054=CARTESIAN_POINT('Ctrl Pts',(29.37557606376,8.99442305443429,135.70570254201));
#41055=CARTESIAN_POINT('Ctrl Pts',(29.3968663992163,8.99354972599348,135.698345055793));
#41056=CARTESIAN_POINT('Ctrl Pts',(29.4183247605901,8.99263100796461,135.691382689721));
#41057=CARTESIAN_POINT('Ctrl Pts',(29.5876905334005,8.98495128128084,135.639444028187));
#41058=CARTESIAN_POINT('Ctrl Pts',(29.8197767178098,8.97487183787893,135.600774173325));
#41059=CARTESIAN_POINT('Ctrl Pts',(30.1801225306472,8.97481364719588,135.600649477793));
#41060=CARTESIAN_POINT('Ctrl Pts',(30.4123373861891,8.9849459908676,135.639432675438));
#41061=CARTESIAN_POINT('Ctrl Pts',(30.581672548813,8.99263090028869,135.69138245992));
#41062=CARTESIAN_POINT('Ctrl Pts',(30.6031336007837,8.99354972599348,135.698345055793));
#41063=CARTESIAN_POINT('Ctrl Pts',(30.62442393624,8.99442305443429,135.70570254201));
#41064=CARTESIAN_POINT('Ctrl Pts',(29.3865147164033,8.96294870295619,135.737135028007));
#41065=CARTESIAN_POINT('Ctrl Pts',(29.4073414853149,8.96237089086999,135.729918298573));
#41066=CARTESIAN_POINT('Ctrl Pts',(29.4283459629072,8.96172231480688,135.723090172466));
#41067=CARTESIAN_POINT('Ctrl Pts',(29.5942372931042,8.95618694003155,135.671989821309));
#41068=CARTESIAN_POINT('Ctrl Pts',(29.8225190849717,8.94781763959254,135.633524301555));
#41069=CARTESIAN_POINT('Ctrl Pts',(30.1773808279966,8.94775803303614,135.63340083736));
#41070=CARTESIAN_POINT('Ctrl Pts',(30.4057900063053,8.9561825817824,135.671977657887));
#41071=CARTESIAN_POINT('Ctrl Pts',(30.5716514674437,8.96172203669286,135.723090090889));
#41072=CARTESIAN_POINT('Ctrl Pts',(30.5926584142642,8.96237102991341,135.729918177652));
#41073=CARTESIAN_POINT('Ctrl Pts',(30.6134852835967,8.96294870295619,135.737135028007));
#41074=CARTESIAN_POINT('Ctrl Pts',(29.3974533690467,8.9314743514781,135.768567514004));
#41075=CARTESIAN_POINT('Ctrl Pts',(29.417815214517,8.93117883512348,135.761502062769));
#41076=CARTESIAN_POINT('Ctrl Pts',(29.4383685133733,8.93082738428349,135.754786613407));
#41077=CARTESIAN_POINT('Ctrl Pts',(29.6007799711022,8.92734716856884,135.704598391766));
#41078=CARTESIAN_POINT('Ctrl Pts',(29.8252639490309,8.92072266060556,135.666303758425));
#41079=CARTESIAN_POINT('Ctrl Pts',(30.1746392148318,8.92068624425422,135.666171804744));
#41080=CARTESIAN_POINT('Ctrl Pts',(30.3992472965949,8.9273427984036,135.704587303278));
#41081=CARTESIAN_POINT('Ctrl Pts',(30.5616287975597,8.93082748462833,135.75478622414));
#41082=CARTESIAN_POINT('Ctrl Pts',(30.5821848859038,8.93117869608006,135.761502183691));
#41083=CARTESIAN_POINT('Ctrl Pts',(30.6025466309533,8.9314743514781,135.768567514004));
#41084=CARTESIAN_POINT('Ctrl Pts',(29.40839202169,8.9,135.8));
#41085=CARTESIAN_POINT('Ctrl Pts',(29.4282903006156,8.9,135.793075305549));
#41086=CARTESIAN_POINT('Ctrl Pts',(29.4483897156904,8.89991869112576,135.786494096152));
#41087=CARTESIAN_POINT('Ctrl Pts',(29.6073267308058,8.89858282731955,135.737144184887));
#41088=CARTESIAN_POINT('Ctrl Pts',(29.8280063161928,8.89366846231917,135.699053886655));
#41089=CARTESIAN_POINT('Ctrl Pts',(30.1718975121812,8.89363063009448,135.698923164311));
#41090=CARTESIAN_POINT('Ctrl Pts',(30.3926999167111,8.8985793893184,135.737132285728));
#41091=CARTESIAN_POINT('Ctrl Pts',(30.5516077161905,8.8999186210325,135.78649385511));
#41092=CARTESIAN_POINT('Ctrl Pts',(30.5717096993844,8.9,135.793075305549));
#41093=CARTESIAN_POINT('Ctrl Pts',(30.59160797831,8.9,135.8));
#41094=CARTESIAN_POINT('',(30.59160797831,8.9,135.8));
#41095=CARTESIAN_POINT('',(30.59160797831,8.9,135.8));
#41096=CARTESIAN_POINT('',(29.40839202169,8.9,135.8));
#41097=CARTESIAN_POINT('',(29.37557606376,8.99442305443429,135.70570254201));
#41098=CARTESIAN_POINT('Ctrl Pts',(29.40839202169,8.9,135.8));
#41099=CARTESIAN_POINT('Ctrl Pts',(29.4282903006156,8.9,135.793075305549));
#41100=CARTESIAN_POINT('Ctrl Pts',(29.4483897156904,8.89991869112576,135.786494096152));
#41101=CARTESIAN_POINT('Ctrl Pts',(29.6073267308058,8.89858282731955,135.737144184887));
#41102=CARTESIAN_POINT('Ctrl Pts',(29.8280063161928,8.89366846231917,135.699053886655));
#41103=CARTESIAN_POINT('Ctrl Pts',(30.1718975121812,8.89363063009448,135.698923164311));
#41104=CARTESIAN_POINT('Ctrl Pts',(30.3926999167111,8.8985793893184,135.737132285728));
#41105=CARTESIAN_POINT('Ctrl Pts',(30.5516077161905,8.8999186210325,135.78649385511));
#41106=CARTESIAN_POINT('Ctrl Pts',(30.5717096993844,8.9,135.793075305549));
#41107=CARTESIAN_POINT('Ctrl Pts',(30.59160797831,8.9,135.8));
#41108=CARTESIAN_POINT('Ctrl Pts',(29.1514718625761,9.,135.8));
#41109=CARTESIAN_POINT('Ctrl Pts',(29.2240383852933,9.,135.763779566847));
#41110=CARTESIAN_POINT('Ctrl Pts',(29.2989266202372,8.99756721057679,135.732190956222));
#41111=CARTESIAN_POINT('Ctrl Pts',(29.37557606376,8.99442305443429,135.70570254201));
#41112=CARTESIAN_POINT('Ctrl Pts',(29.1663583211274,8.96666666666667,135.829824561404));
#41113=CARTESIAN_POINT('Ctrl Pts',(29.2376517469549,8.96666666666667,135.794239574446));
#41114=CARTESIAN_POINT('Ctrl Pts',(29.3112262464824,8.96504480705119,135.763211800971));
#41115=CARTESIAN_POINT('Ctrl Pts',(29.3865147164034,8.96294870295619,135.737135028007));
#41116=CARTESIAN_POINT('Ctrl Pts',(29.1812447796787,8.93333333333333,135.859649122807));
#41117=CARTESIAN_POINT('Ctrl Pts',(29.2512651086164,8.93333333333333,135.824699582045));
#41118=CARTESIAN_POINT('Ctrl Pts',(29.3235258727276,8.9325224035256,135.79423264572));
#41119=CARTESIAN_POINT('Ctrl Pts',(29.3974533690467,8.9314743514781,135.768567514003));
#41120=CARTESIAN_POINT('Ctrl Pts',(29.19613123823,8.9,135.889473684211));
#41121=CARTESIAN_POINT('Ctrl Pts',(29.2648784702779,8.9,135.855159589644));
#41122=CARTESIAN_POINT('Ctrl Pts',(29.3358254989728,8.9,135.825253490469));
#41123=CARTESIAN_POINT('Ctrl Pts',(29.40839202169,8.9,135.8));
#41124=CARTESIAN_POINT('Ctrl Pts',(29.19613123823,8.9,135.889473684211));
#41125=CARTESIAN_POINT('Ctrl Pts',(29.2648784702779,8.9,135.855159589644));
#41126=CARTESIAN_POINT('Ctrl Pts',(29.3358254989728,8.9,135.825253490469));
#41127=CARTESIAN_POINT('Ctrl Pts',(29.40839202169,8.9,135.8));
#41128=CARTESIAN_POINT('Ctrl Pts',(30.62442393624,8.99442305443429,135.70570254201));
#41129=CARTESIAN_POINT('Ctrl Pts',(30.7010733797633,8.99756721057681,135.732190956222));
#41130=CARTESIAN_POINT('Ctrl Pts',(30.7759616147075,9.00000000000003,135.763779566847));
#41131=CARTESIAN_POINT('Ctrl Pts',(30.8485281374252,9.,135.800000000001));
#41132=CARTESIAN_POINT('Ctrl Pts',(30.6134852835967,8.96294870295619,135.737135028007));
#41133=CARTESIAN_POINT('Ctrl Pts',(30.6887737535181,8.96504480705121,135.763211800971));
#41134=CARTESIAN_POINT('Ctrl Pts',(30.762348253046,8.96666666666669,135.794239574446));
#41135=CARTESIAN_POINT('Ctrl Pts',(30.8336416788738,8.96666666666667,135.829824561404));
#41136=CARTESIAN_POINT('Ctrl Pts',(30.6025466309533,8.9314743514781,135.768567514003));
#41137=CARTESIAN_POINT('Ctrl Pts',(30.6764741272728,8.9325224035256,135.79423264572));
#41138=CARTESIAN_POINT('Ctrl Pts',(30.7487348913845,8.93333333333334,135.824699582045));
#41139=CARTESIAN_POINT('Ctrl Pts',(30.8187552203225,8.93333333333333,135.859649122808));
#41140=CARTESIAN_POINT('Ctrl Pts',(30.59160797831,8.9,135.8));
#41141=CARTESIAN_POINT('Ctrl Pts',(30.6641745010276,8.9,135.825253490469));
#41142=CARTESIAN_POINT('Ctrl Pts',(30.7351215297229,8.9,135.855159589645));
#41143=CARTESIAN_POINT('Ctrl Pts',(30.8038687617712,8.9,135.889473684211));
#41144=CARTESIAN_POINT('Ctrl Pts',(30.59160797831,8.9,135.8));
#41145=CARTESIAN_POINT('Ctrl Pts',(30.6641745010276,8.9,135.825253490469));
#41146=CARTESIAN_POINT('Ctrl Pts',(30.7351215297229,8.9,135.855159589645));
#41147=CARTESIAN_POINT('Ctrl Pts',(30.8038687617712,8.9,135.889473684211));
#41148=CARTESIAN_POINT('Origin',(30.,9.1,137.5));
#41149=CARTESIAN_POINT('',(28.2,8.5,137.5));
#41150=CARTESIAN_POINT('',(28.2,9.1,137.5));
#41151=CARTESIAN_POINT('',(28.8951880620293,8.5,136.078947368421));
#41152=CARTESIAN_POINT('Origin',(30.,8.5,137.5));
#41153=CARTESIAN_POINT('',(29.0050125628934,8.5,136.));
#41154=CARTESIAN_POINT('Ctrl Pts',(29.0050125628934,8.5,136.));
#41155=CARTESIAN_POINT('Ctrl Pts',(28.9674326867105,8.5,136.024927669793));
#41156=CARTESIAN_POINT('Ctrl Pts',(28.9307900499921,8.5,136.051268237865));
#41157=CARTESIAN_POINT('Ctrl Pts',(28.8951880620293,8.5,136.078947368421));
#41158=CARTESIAN_POINT('',(30.9949874371066,8.5,136.));
#41159=CARTESIAN_POINT('Ctrl Pts',(30.9949874371066,8.5,136.));
#41160=CARTESIAN_POINT('Ctrl Pts',(30.9864258065899,8.5,135.994320856796));
#41161=CARTESIAN_POINT('Ctrl Pts',(30.9778385803597,8.49988842326335,135.98872938726));
#41162=CARTESIAN_POINT('Ctrl Pts',(30.969224994042,8.49967132634843,135.983225754498));
#41163=CARTESIAN_POINT('Ctrl Pts',(30.9575122929155,8.49937611931315,135.975741948882));
#41164=CARTESIAN_POINT('Ctrl Pts',(30.9457713217168,8.49890678768928,135.968421934072));
#41165=CARTESIAN_POINT('Ctrl Pts',(30.9339557970041,8.49823106356219,135.961260087485));
#41166=CARTESIAN_POINT('Ctrl Pts',(30.672656166037,8.48328746441287,135.802876273328));
#41167=CARTESIAN_POINT('Ctrl Pts',(30.3954457405881,8.39151314723882,135.72337153152));
#41168=CARTESIAN_POINT('Ctrl Pts',(30.12651806476,8.36979419621021,135.704342425858));
#41169=CARTESIAN_POINT('Ctrl Pts',(30.1036961845309,8.36795107129735,135.702727568001));
#41170=CARTESIAN_POINT('Ctrl Pts',(30.0808655520404,8.36653921144899,135.701565046591));
#41171=CARTESIAN_POINT('Ctrl Pts',(30.0580358116452,8.3656616809124,135.700830713729));
#41172=CARTESIAN_POINT('Ctrl Pts',(30.047033558372,8.36523877583107,135.700476819378));
#41173=CARTESIAN_POINT('Ctrl Pts',(30.0360377469811,8.36493371946735,135.700224932826));
#41174=CARTESIAN_POINT('Ctrl Pts',(30.0250383816017,8.36475069000845,135.70007315735));
#41175=CARTESIAN_POINT('Ctrl Pts',(30.0034967468638,8.36439223716922,135.699775913669));
#41176=CARTESIAN_POINT('Ctrl Pts',(29.9819578260176,8.36450298023026,135.69986705092));
#41177=CARTESIAN_POINT('Ctrl Pts',(29.9604219380954,8.36507608574144,135.700340519536));
#41178=CARTESIAN_POINT('Ctrl Pts',(29.9360173607035,8.36572553181268,135.700877056574));
#41179=CARTESIAN_POINT('Ctrl Pts',(29.911581134165,8.36698783297317,135.701939651609));
#41180=CARTESIAN_POINT('Ctrl Pts',(29.8872393421969,8.36876645171126,135.703437238886));
#41181=CARTESIAN_POINT('Ctrl Pts',(29.6648767426176,8.38501415799279,135.717117718958));
#41182=CARTESIAN_POINT('Ctrl Pts',(29.4328429101899,8.45069979287912,135.774591014166));
#41183=CARTESIAN_POINT('Ctrl Pts',(29.2152684605821,8.48252846513542,135.880025058399));
#41184=CARTESIAN_POINT('Ctrl Pts',(29.1790060523141,8.48783324384481,135.897597399105));
#41185=CARTESIAN_POINT('Ctrl Pts',(29.1431452935689,8.49219755137002,135.916501982839));
#41186=CARTESIAN_POINT('Ctrl Pts',(29.1081615516992,8.49523924040882,135.936454666153));
#41187=CARTESIAN_POINT('Ctrl Pts',(29.0731778098294,8.49828092944762,135.956407349467));
#41188=CARTESIAN_POINT('Ctrl Pts',(29.0390710848352,8.5,135.977408132361));
#41189=CARTESIAN_POINT('Ctrl Pts',(29.0050125628934,8.5,136.));
#41190=CARTESIAN_POINT('',(31.1048119379707,8.5,136.078947368421));
#41191=CARTESIAN_POINT('Ctrl Pts',(31.1048119379707,8.5,136.078947368421));
#41192=CARTESIAN_POINT('Ctrl Pts',(31.0692099500079,8.5,136.051268237865));
#41193=CARTESIAN_POINT('Ctrl Pts',(31.0325673132895,8.5,136.024927669793));
#41194=CARTESIAN_POINT('Ctrl Pts',(30.9949874371066,8.5,136.));
#41195=CARTESIAN_POINT('Origin',(30.,8.5,137.5));
#41196=CARTESIAN_POINT('Ctrl Pts',(31.0500544632573,8.39129047171135,135.916983334517));
#41197=CARTESIAN_POINT('Ctrl Pts',(31.0416572725171,8.39013445090614,135.911534549944));
#41198=CARTESIAN_POINT('Ctrl Pts',(31.0332269292893,8.38887979850224,135.906181548932));
#41199=CARTESIAN_POINT('Ctrl Pts',(31.0132512017485,8.38570823783423,135.893775706518));
#41200=CARTESIAN_POINT('Ctrl Pts',(31.0017011490689,8.38371414702549,135.886801483368));
#41201=CARTESIAN_POINT('Ctrl Pts',(30.73243501588,8.33432174868635,135.729698539418));
#41202=CARTESIAN_POINT('Ctrl Pts',(30.4528075616641,8.21969538053694,135.663791800073));
#41203=CARTESIAN_POINT('Ctrl Pts',(30.1194544951314,8.18662675501976,135.646080977264));
#41204=CARTESIAN_POINT('Ctrl Pts',(30.0932684231087,8.18474888991971,135.645104148142));
#41205=CARTESIAN_POINT('Ctrl Pts',(30.0542637892422,8.18295722410468,135.644178995873));
#41206=CARTESIAN_POINT('Ctrl Pts',(30.0415691426709,8.18254082843928,135.643965691679));
#41207=CARTESIAN_POINT('Ctrl Pts',(30.0039648708177,8.18179778951162,135.64358472223));
#41208=CARTESIAN_POINT('Ctrl Pts',(29.9790422078338,8.18194773384953,135.643661590033));
#41209=CARTESIAN_POINT('Ctrl Pts',(29.9259892365849,8.18363575834559,135.644519987645));
#41210=CARTESIAN_POINT('Ctrl Pts',(29.8979097346567,8.18532290965731,135.645414992116));
#41211=CARTESIAN_POINT('Ctrl Pts',(29.6150612328207,8.21055133692172,135.658397917784));
#41212=CARTESIAN_POINT('Ctrl Pts',(29.3353440644627,8.30782885450725,135.714217769816));
#41213=CARTESIAN_POINT('Ctrl Pts',(29.0505321085055,8.3745011316311,135.855362112556));
#41214=CARTESIAN_POINT('Ctrl Pts',(28.9833499104208,8.38669177291416,135.895307843082));
#41215=CARTESIAN_POINT('Ctrl Pts',(28.9499455367427,8.39129047171135,135.916983334517));
#41216=CARTESIAN_POINT('Ctrl Pts',(31.0316987878737,8.4275269811409,135.944655556345));
#41217=CARTESIAN_POINT('Ctrl Pts',(31.0232496115585,8.42674793297165,135.939128693744));
#41218=CARTESIAN_POINT('Ctrl Pts',(31.0147601027094,8.42589417137142,135.933699269146));
#41219=CARTESIAN_POINT('Ctrl Pts',(30.9946782507695,8.42357762853484,135.921094749865));
#41220=CARTESIAN_POINT('Ctrl Pts',(30.9830484738135,8.42213322181795,135.914011559485));
#41221=CARTESIAN_POINT('Ctrl Pts',(30.7126277643191,8.3839211305528,135.754083580217));
#41222=CARTESIAN_POINT('Ctrl Pts',(30.4334575445295,8.27676192071996,135.683612800791));
#41223=CARTESIAN_POINT('Ctrl Pts',(30.11421209809,8.24716089858398,135.664984304196));
#41224=CARTESIAN_POINT('Ctrl Pts',(30.0891005771669,8.24535197239345,135.663930548954));
#41225=CARTESIAN_POINT('Ctrl Pts',(30.0518486109606,8.24377963463304,135.662960509384));
#41226=CARTESIAN_POINT('Ctrl Pts',(30.0397052276191,8.2433830423102,135.66273192281));
#41227=CARTESIAN_POINT('Ctrl Pts',(30.0038065076672,8.24270601822244,135.662326479773));
#41228=CARTESIAN_POINT('Ctrl Pts',(29.9799830207133,8.24285973044089,135.662414140564));
#41229=CARTESIAN_POINT('Ctrl Pts',(29.9293414259812,8.24435747176978,135.66331209502));
#41230=CARTESIAN_POINT('Ctrl Pts',(29.9024170132781,8.24595661414936,135.664279393149));
#41231=CARTESIAN_POINT('Ctrl Pts',(29.6318884637786,8.26858643327872,135.677933353777));
#41232=CARTESIAN_POINT('Ctrl Pts',(29.3549087480204,8.35906934575154,135.737533569262));
#41233=CARTESIAN_POINT('Ctrl Pts',(29.0694554505283,8.41521142211316,135.882050996154));
#41234=CARTESIAN_POINT('Ctrl Pts',(29.0019254602039,8.42441726441167,135.922670690471));
#41235=CARTESIAN_POINT('Ctrl Pts',(28.9683012121262,8.4275269811409,135.944655556345));
#41236=CARTESIAN_POINT('Ctrl Pts',(31.0133431124902,8.46376349057045,135.972327778172));
#41237=CARTESIAN_POINT('Ctrl Pts',(31.0048334675486,8.46338651793449,135.966726712996));
#41238=CARTESIAN_POINT('Ctrl Pts',(30.9963054069395,8.46287405039417,135.961211667046));
#41239=CARTESIAN_POINT('Ctrl Pts',(30.9760852438945,8.46150672861254,135.948422905536));
#41240=CARTESIAN_POINT('Ctrl Pts',(30.9644239969721,8.46048771289681,135.941211857955));
#41241=CARTESIAN_POINT('Ctrl Pts',(30.6924634175979,8.43368808254642,135.778491232529));
#41242=CARTESIAN_POINT('Ctrl Pts',(30.4147957577227,8.3344466070558,135.703550530802));
#41243=CARTESIAN_POINT('Ctrl Pts',(30.1089385815722,8.30741692773313,135.683824241069));
#41244=CARTESIAN_POINT('Ctrl Pts',(30.0850333979822,8.30593612897524,135.68273864578));
#41245=CARTESIAN_POINT('Ctrl Pts',(30.0494487366536,8.30441636530272,135.681695305867));
#41246=CARTESIAN_POINT('Ctrl Pts',(30.0379016620329,8.30409150559643,135.681458701694));
#41247=CARTESIAN_POINT('Ctrl Pts',(30.0036551100143,8.3034840084584,135.681034156126));
#41248=CARTESIAN_POINT('Ctrl Pts',(29.981017013138,8.3035909836389,135.681114500388));
#41249=CARTESIAN_POINT('Ctrl Pts',(29.9326651713072,8.30500381838849,135.682084949199));
#41250=CARTESIAN_POINT('Ctrl Pts',(29.9070738555437,8.30635412848112,135.683075250576));
#41251=CARTESIAN_POINT('Ctrl Pts',(29.6480495116597,8.32697906163579,135.697582282965));
#41252=CARTESIAN_POINT('Ctrl Pts',(29.3746059212276,8.41040690744922,135.760854097255));
#41253=CARTESIAN_POINT('Ctrl Pts',(29.0883611928009,8.45585156841319,135.908717682976));
#41254=CARTESIAN_POINT('Ctrl Pts',(29.020495535052,8.46227450850248,135.950045284972));
#41255=CARTESIAN_POINT('Ctrl Pts',(28.9866568875098,8.46376349057045,135.972327778172));
#41256=CARTESIAN_POINT('Ctrl Pts',(30.9949874371066,8.5,136.));
#41257=CARTESIAN_POINT('Ctrl Pts',(30.9864258065899,8.5,135.994320856796));
#41258=CARTESIAN_POINT('Ctrl Pts',(30.9778385803597,8.49988842326335,135.98872938726));
#41259=CARTESIAN_POINT('Ctrl Pts',(30.9575122929155,8.49937611931315,135.975741948882));
#41260=CARTESIAN_POINT('Ctrl Pts',(30.9457713217168,8.49890678768928,135.968421934072));
#41261=CARTESIAN_POINT('Ctrl Pts',(30.672656166037,8.48328746441287,135.802876273328));
#41262=CARTESIAN_POINT('Ctrl Pts',(30.3954457405881,8.39151314723882,135.72337153152));
#41263=CARTESIAN_POINT('Ctrl Pts',(30.1036961845309,8.36795107129735,135.702727568001));
#41264=CARTESIAN_POINT('Ctrl Pts',(30.0808655520404,8.36653921144899,135.701565046591));
#41265=CARTESIAN_POINT('Ctrl Pts',(30.047033558372,8.36523877583107,135.700476819378));
#41266=CARTESIAN_POINT('Ctrl Pts',(30.0360377469811,8.36493371946735,135.700224932826));
#41267=CARTESIAN_POINT('Ctrl Pts',(30.0034967468638,8.36439223716922,135.699775913669));
#41268=CARTESIAN_POINT('Ctrl Pts',(29.9819578260176,8.36450298023026,135.69986705092));
#41269=CARTESIAN_POINT('Ctrl Pts',(29.9360173607035,8.36572553181268,135.700877056574));
#41270=CARTESIAN_POINT('Ctrl Pts',(29.911581134165,8.36698783297317,135.701939651609));
#41271=CARTESIAN_POINT('Ctrl Pts',(29.6648767426176,8.38501415799279,135.717117718958));
#41272=CARTESIAN_POINT('Ctrl Pts',(29.3941706047853,8.46164739869351,135.784169896701));
#41273=CARTESIAN_POINT('Ctrl Pts',(29.1072845348237,8.49656185889524,135.935406566573));
#41274=CARTESIAN_POINT('Ctrl Pts',(29.0390710848352,8.5,135.977408132361));
#41275=CARTESIAN_POINT('Ctrl Pts',(29.0050125628934,8.5,136.));
#41276=CARTESIAN_POINT('',(31.0500544632573,8.39129047171135,135.916983334517));
#41277=CARTESIAN_POINT('',(29.0050125628934,8.5,136.));
#41278=CARTESIAN_POINT('Origin',(30.,8.45,137.5));
#41279=CARTESIAN_POINT('',(28.8338096210309,8.4,136.));
#41280=CARTESIAN_POINT('',(31.1048119379707,8.5,136.078947368421));
#41281=CARTESIAN_POINT('Ctrl Pts',(28.9499455367427,8.39129047171135,135.916983334517));
#41282=CARTESIAN_POINT('Ctrl Pts',(28.9100201948422,8.39678689632762,135.942890163806));
#41283=CARTESIAN_POINT('Ctrl Pts',(28.8713894960226,8.40000000009859,135.970783140825));
#41284=CARTESIAN_POINT('Ctrl Pts',(28.8338096192947,8.4,136.00000000135));
#41285=CARTESIAN_POINT('Ctrl Pts',(28.9683012121262,8.4275269811409,135.944655556345));
#41286=CARTESIAN_POINT('Ctrl Pts',(28.9291576919387,8.43119126421841,135.970235999263));
#41287=CARTESIAN_POINT('Ctrl Pts',(28.8911896803029,8.43333333339906,135.997611506775));
#41288=CARTESIAN_POINT('Ctrl Pts',(28.854269099658,8.43333333333333,136.0263157908));
#41289=CARTESIAN_POINT('Ctrl Pts',(28.9866568875098,8.46376349057045,135.972327778172));
#41290=CARTESIAN_POINT('Ctrl Pts',(28.9482951890352,8.46559563210921,135.99758183472));
#41291=CARTESIAN_POINT('Ctrl Pts',(28.9109898645832,8.46666666669953,136.024439872726));
#41292=CARTESIAN_POINT('Ctrl Pts',(28.8747285800212,8.46666666666667,136.05263158025));
#41293=CARTESIAN_POINT('Ctrl Pts',(29.0050125628934,8.5,136.));
#41294=CARTESIAN_POINT('Ctrl Pts',(28.9674326861317,8.5,136.024927670177));
#41295=CARTESIAN_POINT('Ctrl Pts',(28.9307900488635,8.5,136.051268238676));
#41296=CARTESIAN_POINT('Ctrl Pts',(28.8951880603845,8.5,136.0789473697));
#41297=CARTESIAN_POINT('Ctrl Pts',(31.166190378969,8.4,136.));
#41298=CARTESIAN_POINT('Ctrl Pts',(31.1286105027861,8.4,135.970783139968));
#41299=CARTESIAN_POINT('Ctrl Pts',(31.0899798045429,8.39678689624297,135.942890163407));
#41300=CARTESIAN_POINT('Ctrl Pts',(31.0500544632573,8.39129047171135,135.916983334517));
#41301=CARTESIAN_POINT('Ctrl Pts',(31.1457308986363,8.43333333333333,136.026315789474));
#41302=CARTESIAN_POINT('Ctrl Pts',(31.1088103185267,8.43333333333333,135.997611505934));
#41303=CARTESIAN_POINT('Ctrl Pts',(31.0708423074584,8.43119126416198,135.970235998869));
#41304=CARTESIAN_POINT('Ctrl Pts',(31.0316987878737,8.4275269811409,135.944655556345));
#41305=CARTESIAN_POINT('Ctrl Pts',(31.1252714183035,8.46666666666667,136.052631578947));
#41306=CARTESIAN_POINT('Ctrl Pts',(31.0890101342673,8.46666666666667,136.024439871899));
#41307=CARTESIAN_POINT('Ctrl Pts',(31.051704810374,8.46559563208099,135.997581834331));
#41308=CARTESIAN_POINT('Ctrl Pts',(31.0133431124902,8.46376349057045,135.972327778172));
#41309=CARTESIAN_POINT('Ctrl Pts',(31.1048119379707,8.5,136.078947368421));
#41310=CARTESIAN_POINT('Ctrl Pts',(31.0692099500079,8.5,136.051268237865));
#41311=CARTESIAN_POINT('Ctrl Pts',(31.0325673132895,8.5,136.024927669793));
#41312=CARTESIAN_POINT('Ctrl Pts',(30.9949874371066,8.5,136.));
#41313=CARTESIAN_POINT('Origin',(18.5,0.,134.05));
#41314=CARTESIAN_POINT('',(17.895,7.40911313484149E-17,134.));
#41315=CARTESIAN_POINT('Origin',(18.5,0.,134.));
#41316=CARTESIAN_POINT('',(17.995,-6.18446633569412E-17,134.1));
#41317=CARTESIAN_POINT('',(17.945,6.79678973526781E-17,134.05));
#41318=CARTESIAN_POINT('Origin',(18.5,0.,134.1));
#41319=CARTESIAN_POINT('Origin',(18.5,0.,134.));
#41320=CARTESIAN_POINT('',(17.995,6.18446633569412E-17,134.9));
#41321=CARTESIAN_POINT('',(17.995,-6.18446633569412E-17,134.));
#41322=CARTESIAN_POINT('Origin',(18.5,0.,134.9));
#41323=CARTESIAN_POINT('Origin',(0.,0.,134.));
#41324=CARTESIAN_POINT('',(-19.105,7.40911313484149E-17,134.));
#41325=CARTESIAN_POINT('Origin',(-18.5,0.,134.));
#41326=CARTESIAN_POINT('Origin',(18.5,0.,134.95));
#41327=CARTESIAN_POINT('',(17.895,-7.40911313484149E-17,135.));
#41328=CARTESIAN_POINT('Origin',(18.5,0.,135.));
#41329=CARTESIAN_POINT('',(17.945,-6.79678973526781E-17,134.95));
#41330=CARTESIAN_POINT('Origin',(0.,0.,135.));
#41331=CARTESIAN_POINT('',(-25.8,9.,135.));
#41332=CARTESIAN_POINT('',(-19.105,-7.40911313484149E-17,135.));
#41333=CARTESIAN_POINT('Origin',(-18.5,0.,135.));
#41334=CARTESIAN_POINT('Origin',(-18.5,0.,134.05));
#41335=CARTESIAN_POINT('',(-19.005,-6.18446633569412E-17,134.1));
#41336=CARTESIAN_POINT('',(-19.055,6.79678973526781E-17,134.05));
#41337=CARTESIAN_POINT('Origin',(-18.5,0.,134.1));
#41338=CARTESIAN_POINT('Origin',(-18.5,0.,134.));
#41339=CARTESIAN_POINT('',(-19.005,6.18446633569412E-17,134.9));
#41340=CARTESIAN_POINT('',(-19.005,-6.18446633569412E-17,134.));
#41341=CARTESIAN_POINT('Origin',(-18.5,0.,134.9));
#41342=CARTESIAN_POINT('Origin',(-18.5,0.,134.95));
#41343=CARTESIAN_POINT('',(-19.055,-6.79678973526781E-17,134.95));
#41344=CARTESIAN_POINT('Ctrl Pts',(5.24283818900585,-9.,140.915348529816));
#41345=CARTESIAN_POINT('Ctrl Pts',(5.24283818900585,-8.9,140.915348529816));
#41346=CARTESIAN_POINT('Ctrl Pts',(5.00361661612988,-9.,141.188950061798));
#41347=CARTESIAN_POINT('Ctrl Pts',(5.00361661612988,-8.9,141.188950061798));
#41348=CARTESIAN_POINT('Ctrl Pts',(4.59392957389355,-9.,141.188950061798));
#41349=CARTESIAN_POINT('Ctrl Pts',(4.59392957389355,-8.9,141.188950061798));
#41350=CARTESIAN_POINT('',(5.24283818900585,-9.,140.915348529816));
#41351=CARTESIAN_POINT('',(4.59392957389355,-9.,141.188950061798));
#41352=CARTESIAN_POINT('Ctrl Pts',(5.24283818900585,-9.,140.915348529816));
#41353=CARTESIAN_POINT('Ctrl Pts',(5.00361661612988,-9.,141.188950061798));
#41354=CARTESIAN_POINT('Ctrl Pts',(4.59392957389355,-9.,141.188950061798));
#41355=CARTESIAN_POINT('',(5.24283818900585,-8.9,140.915348529816));
#41356=CARTESIAN_POINT('',(5.24283818900585,-9.,140.915348529816));
#41357=CARTESIAN_POINT('',(4.59392957389355,-8.9,141.188950061798));
#41358=CARTESIAN_POINT('Ctrl Pts',(5.24283818900585,-8.9,140.915348529816));
#41359=CARTESIAN_POINT('Ctrl Pts',(5.00361661612988,-8.9,141.188950061798));
#41360=CARTESIAN_POINT('Ctrl Pts',(4.59392957389355,-8.9,141.188950061798));
#41361=CARTESIAN_POINT('',(4.59392957389355,-9.,141.188950061798));
#41362=CARTESIAN_POINT('Ctrl Pts',(5.48205976188183,-9.,140.048704624176));
#41363=CARTESIAN_POINT('Ctrl Pts',(5.48205976188183,-8.9,140.048704624176));
#41364=CARTESIAN_POINT('Ctrl Pts',(5.48205976188183,-9.,140.641746997833));
#41365=CARTESIAN_POINT('Ctrl Pts',(5.48205976188183,-8.9,140.641746997833));
#41366=CARTESIAN_POINT('Ctrl Pts',(5.24283818900585,-9.,140.915348529816));
#41367=CARTESIAN_POINT('Ctrl Pts',(5.24283818900585,-8.9,140.915348529816));
#41368=CARTESIAN_POINT('',(5.48205976188183,-9.,140.048704624176));
#41369=CARTESIAN_POINT('Ctrl Pts',(5.48205976188183,-9.,140.048704624176));
#41370=CARTESIAN_POINT('Ctrl Pts',(5.48205976188183,-9.,140.641746997833));
#41371=CARTESIAN_POINT('Ctrl Pts',(5.24283818900585,-9.,140.915348529816));
#41372=CARTESIAN_POINT('',(5.48205976188183,-8.9,140.048704624176));
#41373=CARTESIAN_POINT('',(5.48205976188183,-9.,140.048704624176));
#41374=CARTESIAN_POINT('Ctrl Pts',(5.48205976188183,-8.9,140.048704624176));
#41375=CARTESIAN_POINT('Ctrl Pts',(5.48205976188183,-8.9,140.641746997833));
#41376=CARTESIAN_POINT('Ctrl Pts',(5.24283818900585,-8.9,140.915348529816));
#41377=CARTESIAN_POINT('Ctrl Pts',(5.25286512076855,-9.,139.071760654449));
#41378=CARTESIAN_POINT('Ctrl Pts',(5.25286512076855,-8.9,139.071760654449));
#41379=CARTESIAN_POINT('Ctrl Pts',(5.48205976188183,-9.,139.343929767609));
#41380=CARTESIAN_POINT('Ctrl Pts',(5.48205976188183,-8.9,139.343929767609));
#41381=CARTESIAN_POINT('Ctrl Pts',(5.48205976188183,-9.,140.048704624176));
#41382=CARTESIAN_POINT('Ctrl Pts',(5.48205976188183,-8.9,140.048704624176));
#41383=CARTESIAN_POINT('',(5.25286512076855,-9.,139.071760654449));
#41384=CARTESIAN_POINT('Ctrl Pts',(5.25286512076855,-9.,139.071760654449));
#41385=CARTESIAN_POINT('Ctrl Pts',(5.48205976188183,-9.,139.343929767609));
#41386=CARTESIAN_POINT('Ctrl Pts',(5.48205976188183,-9.,140.048704624176));
#41387=CARTESIAN_POINT('',(5.25286512076855,-8.9,139.071760654449));
#41388=CARTESIAN_POINT('',(5.25286512076855,-9.,139.071760654449));
#41389=CARTESIAN_POINT('Ctrl Pts',(5.25286512076855,-8.9,139.071760654449));
#41390=CARTESIAN_POINT('Ctrl Pts',(5.48205976188183,-8.9,139.343929767609));
#41391=CARTESIAN_POINT('Ctrl Pts',(5.48205976188183,-8.9,140.048704624176));
#41392=CARTESIAN_POINT('Ctrl Pts',(4.60538892447948,-9.,138.79959154129));
#41393=CARTESIAN_POINT('Ctrl Pts',(4.60538892447948,-8.9,138.79959154129));
#41394=CARTESIAN_POINT('Ctrl Pts',(5.02367047965527,-9.,138.79959154129));
#41395=CARTESIAN_POINT('Ctrl Pts',(5.02367047965527,-8.9,138.79959154129));
#41396=CARTESIAN_POINT('Ctrl Pts',(5.25286512076855,-9.,139.071760654449));
#41397=CARTESIAN_POINT('Ctrl Pts',(5.25286512076855,-8.9,139.071760654449));
#41398=CARTESIAN_POINT('',(4.60538892447948,-9.,138.79959154129));
#41399=CARTESIAN_POINT('Ctrl Pts',(4.60538892447948,-9.,138.79959154129));
#41400=CARTESIAN_POINT('Ctrl Pts',(5.02367047965527,-9.,138.79959154129));
#41401=CARTESIAN_POINT('Ctrl Pts',(5.25286512076855,-9.,139.071760654449));
#41402=CARTESIAN_POINT('',(4.60538892447948,-8.9,138.79959154129));
#41403=CARTESIAN_POINT('',(4.60538892447948,-9.,138.79959154129));
#41404=CARTESIAN_POINT('Ctrl Pts',(4.60538892447948,-8.9,138.79959154129));
#41405=CARTESIAN_POINT('Ctrl Pts',(5.02367047965527,-8.9,138.79959154129));
#41406=CARTESIAN_POINT('Ctrl Pts',(5.25286512076855,-8.9,139.071760654449));
#41407=CARTESIAN_POINT('Ctrl Pts',(3.96220998466015,-9.,139.077490329742));
#41408=CARTESIAN_POINT('Ctrl Pts',(3.96220998466015,-8.9,139.077490329742));
#41409=CARTESIAN_POINT('Ctrl Pts',(4.19856862723827,-9.,138.79959154129));
#41410=CARTESIAN_POINT('Ctrl Pts',(4.19856862723827,-8.9,138.79959154129));
#41411=CARTESIAN_POINT('Ctrl Pts',(4.60538892447948,-9.,138.79959154129));
#41412=CARTESIAN_POINT('Ctrl Pts',(4.60538892447948,-8.9,138.79959154129));
#41413=CARTESIAN_POINT('',(3.96220998466015,-9.,139.077490329742));
#41414=CARTESIAN_POINT('Ctrl Pts',(3.96220998466015,-9.,139.077490329742));
#41415=CARTESIAN_POINT('Ctrl Pts',(4.19856862723827,-9.,138.79959154129));
#41416=CARTESIAN_POINT('Ctrl Pts',(4.60538892447948,-9.,138.79959154129));
#41417=CARTESIAN_POINT('',(3.96220998466015,-8.9,139.077490329742));
#41418=CARTESIAN_POINT('',(3.96220998466015,-9.,139.077490329742));
#41419=CARTESIAN_POINT('Ctrl Pts',(3.96220998466015,-8.9,139.077490329742));
#41420=CARTESIAN_POINT('Ctrl Pts',(4.19856862723827,-8.9,138.79959154129));
#41421=CARTESIAN_POINT('Ctrl Pts',(4.60538892447948,-8.9,138.79959154129));
#41422=CARTESIAN_POINT('Ctrl Pts',(3.72585324943066,-9.,139.991405963898));
#41423=CARTESIAN_POINT('Ctrl Pts',(3.72585324943066,-8.9,139.991405963898));
#41424=CARTESIAN_POINT('Ctrl Pts',(3.72585324943066,-9.,139.355389595032));
#41425=CARTESIAN_POINT('Ctrl Pts',(3.72585324943066,-8.9,139.355389595032));
#41426=CARTESIAN_POINT('Ctrl Pts',(3.96220998466015,-9.,139.077490329742));
#41427=CARTESIAN_POINT('Ctrl Pts',(3.96220998466015,-8.9,139.077490329742));
#41428=CARTESIAN_POINT('',(3.72585324943066,-9.,139.991405963898));
#41429=CARTESIAN_POINT('Ctrl Pts',(3.72585324943066,-9.,139.991405963898));
#41430=CARTESIAN_POINT('Ctrl Pts',(3.72585324943066,-9.,139.355389595032));
#41431=CARTESIAN_POINT('Ctrl Pts',(3.96220998466015,-9.,139.077490329742));
#41432=CARTESIAN_POINT('',(3.72585324943066,-8.9,139.991405963898));
#41433=CARTESIAN_POINT('',(3.72585324943066,-9.,139.991405963898));
#41434=CARTESIAN_POINT('Ctrl Pts',(3.72585324943066,-8.9,139.991405963898));
#41435=CARTESIAN_POINT('Ctrl Pts',(3.72585324943066,-8.9,139.355389595032));
#41436=CARTESIAN_POINT('Ctrl Pts',(3.96220998466015,-8.9,139.077490329742));
#41437=CARTESIAN_POINT('Ctrl Pts',(3.96364431083202,-9.,140.911051273346));
#41438=CARTESIAN_POINT('Ctrl Pts',(3.96364431083202,-8.9,140.911051273346));
#41439=CARTESIAN_POINT('Ctrl Pts',(3.72585324943066,-9.,140.633152008057));
#41440=CARTESIAN_POINT('Ctrl Pts',(3.72585324943066,-8.9,140.633152008057));
#41441=CARTESIAN_POINT('Ctrl Pts',(3.72585324943066,-9.,139.991405963898));
#41442=CARTESIAN_POINT('Ctrl Pts',(3.72585324943066,-8.9,139.991405963898));
#41443=CARTESIAN_POINT('',(3.96364431083202,-9.,140.911051273346));
#41444=CARTESIAN_POINT('Ctrl Pts',(3.96364431083202,-9.,140.911051273346));
#41445=CARTESIAN_POINT('Ctrl Pts',(3.72585324943066,-9.,140.633152008057));
#41446=CARTESIAN_POINT('Ctrl Pts',(3.72585324943066,-9.,139.991405963898));
#41447=CARTESIAN_POINT('',(3.96364431083202,-8.9,140.911051273346));
#41448=CARTESIAN_POINT('',(3.96364431083202,-9.,140.911051273346));
#41449=CARTESIAN_POINT('Ctrl Pts',(3.96364431083202,-8.9,140.911051273346));
#41450=CARTESIAN_POINT('Ctrl Pts',(3.72585324943066,-8.9,140.633152008057));
#41451=CARTESIAN_POINT('Ctrl Pts',(3.72585324943066,-8.9,139.991405963898));
#41452=CARTESIAN_POINT('Ctrl Pts',(4.59392957389355,-9.,141.188950061798));
#41453=CARTESIAN_POINT('Ctrl Pts',(4.59392957389355,-8.9,141.188950061798));
#41454=CARTESIAN_POINT('Ctrl Pts',(4.20143346488476,-9.,141.188950061798));
#41455=CARTESIAN_POINT('Ctrl Pts',(4.20143346488476,-8.9,141.188950061798));
#41456=CARTESIAN_POINT('Ctrl Pts',(3.96364431083202,-9.,140.911051273346));
#41457=CARTESIAN_POINT('Ctrl Pts',(3.96364431083202,-8.9,140.911051273346));
#41458=CARTESIAN_POINT('Ctrl Pts',(4.59392957389355,-9.,141.188950061798));
#41459=CARTESIAN_POINT('Ctrl Pts',(4.20143346488476,-9.,141.188950061798));
#41460=CARTESIAN_POINT('Ctrl Pts',(3.96364431083202,-9.,140.911051273346));
#41461=CARTESIAN_POINT('Ctrl Pts',(4.59392957389355,-8.9,141.188950061798));
#41462=CARTESIAN_POINT('Ctrl Pts',(4.20143346488476,-8.9,141.188950061798));
#41463=CARTESIAN_POINT('Ctrl Pts',(3.96364431083202,-8.9,140.911051273346));
#41464=CARTESIAN_POINT('Ctrl Pts',(3.47230558097363,-9.,138.054707050323));
#41465=CARTESIAN_POINT('Ctrl Pts',(3.47230558097363,-8.9,138.054707050323));
#41466=CARTESIAN_POINT('Ctrl Pts',(3.00675420463085,-9.,138.281037330627));
#41467=CARTESIAN_POINT('Ctrl Pts',(3.00675420463085,-8.9,138.281037330627));
#41468=CARTESIAN_POINT('Ctrl Pts',(2.71739415824413,-9.,138.770942211151));
#41469=CARTESIAN_POINT('Ctrl Pts',(2.71739415824413,-8.9,138.770942211151));
#41470=CARTESIAN_POINT('',(3.47230558097363,-8.9,138.054707050323));
#41471=CARTESIAN_POINT('',(3.47230558097363,-9.,138.054707050323));
#41472=CARTESIAN_POINT('',(2.71739415824413,-8.9,138.770942211151));
#41473=CARTESIAN_POINT('Ctrl Pts',(3.47230558097363,-8.9,138.054707050323));
#41474=CARTESIAN_POINT('Ctrl Pts',(3.00675420463085,-8.9,138.281037330627));
#41475=CARTESIAN_POINT('Ctrl Pts',(2.71739415824413,-8.9,138.770942211151));
#41476=CARTESIAN_POINT('',(2.71739415824413,-9.,138.770942211151));
#41477=CARTESIAN_POINT('Ctrl Pts',(4.64836339652538,-9.,137.828377246857));
#41478=CARTESIAN_POINT('Ctrl Pts',(4.64836339652538,-8.9,137.828377246857));
#41479=CARTESIAN_POINT('Ctrl Pts',(3.93785886466503,-9.,137.828377246857));
#41480=CARTESIAN_POINT('Ctrl Pts',(3.93785886466503,-8.9,137.828377246857));
#41481=CARTESIAN_POINT('Ctrl Pts',(3.47230558097363,-9.,138.054707050323));
#41482=CARTESIAN_POINT('Ctrl Pts',(3.47230558097363,-8.9,138.054707050323));
#41483=CARTESIAN_POINT('',(4.64836339652538,-8.9,137.828377246857));
#41484=CARTESIAN_POINT('',(4.64836339652538,-9.,137.828377246857));
#41485=CARTESIAN_POINT('Ctrl Pts',(4.64836339652538,-8.9,137.828377246857));
#41486=CARTESIAN_POINT('Ctrl Pts',(3.93785886466503,-8.9,137.828377246857));
#41487=CARTESIAN_POINT('Ctrl Pts',(3.47230558097363,-8.9,138.054707050323));
#41488=CARTESIAN_POINT('Ctrl Pts',(5.81582669913769,-9.,138.090518951416));
#41489=CARTESIAN_POINT('Ctrl Pts',(5.81582669913769,-8.9,138.090518951416));
#41490=CARTESIAN_POINT('Ctrl Pts',(5.3474085777998,-9.,137.828377246857));
#41491=CARTESIAN_POINT('Ctrl Pts',(5.3474085777998,-8.9,137.828377246857));
#41492=CARTESIAN_POINT('Ctrl Pts',(4.64836339652538,-9.,137.828377246857));
#41493=CARTESIAN_POINT('Ctrl Pts',(4.64836339652538,-8.9,137.828377246857));
#41494=CARTESIAN_POINT('',(5.81582669913769,-8.9,138.090518951416));
#41495=CARTESIAN_POINT('',(5.81582669913769,-9.,138.090518951416));
#41496=CARTESIAN_POINT('Ctrl Pts',(5.81582669913769,-8.9,138.090518951416));
#41497=CARTESIAN_POINT('Ctrl Pts',(5.3474085777998,-8.9,137.828377246857));
#41498=CARTESIAN_POINT('Ctrl Pts',(4.64836339652538,-8.9,137.828377246857));
#41499=CARTESIAN_POINT('Ctrl Pts',(6.53206090629101,-9.,138.823943138123));
#41500=CARTESIAN_POINT('Ctrl Pts',(6.53206090629101,-8.9,138.823943138123));
#41501=CARTESIAN_POINT('Ctrl Pts',(6.28424291312695,-9.,138.352660655975));
#41502=CARTESIAN_POINT('Ctrl Pts',(6.28424291312695,-8.9,138.352660655975));
#41503=CARTESIAN_POINT('Ctrl Pts',(5.81582669913769,-9.,138.090518951416));
#41504=CARTESIAN_POINT('Ctrl Pts',(5.81582669913769,-8.9,138.090518951416));
#41505=CARTESIAN_POINT('',(6.53206090629101,-8.9,138.823943138123));
#41506=CARTESIAN_POINT('',(6.53206090629101,-9.,138.823943138123));
#41507=CARTESIAN_POINT('Ctrl Pts',(6.53206090629101,-8.9,138.823943138123));
#41508=CARTESIAN_POINT('Ctrl Pts',(6.28424291312695,-8.9,138.352660655975));
#41509=CARTESIAN_POINT('Ctrl Pts',(5.81582669913769,-8.9,138.090518951416));
#41510=CARTESIAN_POINT('Ctrl Pts',(6.77987699210644,-9.,140.031514644623));
#41511=CARTESIAN_POINT('Ctrl Pts',(6.77987699210644,-8.9,140.031514644623));
#41512=CARTESIAN_POINT('Ctrl Pts',(6.77987699210644,-9.,139.29522562027));
#41513=CARTESIAN_POINT('Ctrl Pts',(6.77987699210644,-8.9,139.29522562027));
#41514=CARTESIAN_POINT('Ctrl Pts',(6.53206090629101,-9.,138.823943138123));
#41515=CARTESIAN_POINT('Ctrl Pts',(6.53206090629101,-8.9,138.823943138123));
#41516=CARTESIAN_POINT('',(6.77987699210644,-8.9,140.031514644623));
#41517=CARTESIAN_POINT('',(6.77987699210644,-9.,140.031514644623));
#41518=CARTESIAN_POINT('Ctrl Pts',(6.77987699210644,-8.9,140.031514644623));
#41519=CARTESIAN_POINT('Ctrl Pts',(6.77987699210644,-8.9,139.29522562027));
#41520=CARTESIAN_POINT('Ctrl Pts',(6.53206090629101,-8.9,138.823943138123));
#41521=CARTESIAN_POINT('Ctrl Pts',(6.2126200646162,-9.,141.60866355896));
#41522=CARTESIAN_POINT('Ctrl Pts',(6.2126200646162,-8.9,141.60866355896));
#41523=CARTESIAN_POINT('Ctrl Pts',(6.77987699210644,-9.,141.045703411102));
#41524=CARTESIAN_POINT('Ctrl Pts',(6.77987699210644,-8.9,141.045703411102));
#41525=CARTESIAN_POINT('Ctrl Pts',(6.77987699210644,-9.,140.031514644623));
#41526=CARTESIAN_POINT('Ctrl Pts',(6.77987699210644,-8.9,140.031514644623));
#41527=CARTESIAN_POINT('',(6.2126200646162,-8.9,141.60866355896));
#41528=CARTESIAN_POINT('',(6.2126200646162,-9.,141.60866355896));
#41529=CARTESIAN_POINT('Ctrl Pts',(6.2126200646162,-8.9,141.60866355896));
#41530=CARTESIAN_POINT('Ctrl Pts',(6.77987699210644,-8.9,141.045703411102));
#41531=CARTESIAN_POINT('Ctrl Pts',(6.77987699210644,-8.9,140.031514644623));
#41532=CARTESIAN_POINT('Ctrl Pts',(4.59679441154003,-9.,142.171624183655));
#41533=CARTESIAN_POINT('Ctrl Pts',(4.59679441154003,-8.9,142.171624183655));
#41534=CARTESIAN_POINT('Ctrl Pts',(5.64536122977734,-9.,142.171624183655));
#41535=CARTESIAN_POINT('Ctrl Pts',(5.64536122977734,-8.9,142.171624183655));
#41536=CARTESIAN_POINT('Ctrl Pts',(6.2126200646162,-9.,141.60866355896));
#41537=CARTESIAN_POINT('Ctrl Pts',(6.2126200646162,-8.9,141.60866355896));
#41538=CARTESIAN_POINT('',(4.59679441154003,-8.9,142.171624183655));
#41539=CARTESIAN_POINT('',(4.59679441154003,-9.,142.171624183655));
#41540=CARTESIAN_POINT('Ctrl Pts',(4.59679441154003,-8.9,142.171624183655));
#41541=CARTESIAN_POINT('Ctrl Pts',(5.64536122977734,-8.9,142.171624183655));
#41542=CARTESIAN_POINT('Ctrl Pts',(6.2126200646162,-8.9,141.60866355896));
#41543=CARTESIAN_POINT('Ctrl Pts',(3.00102452933788,-9.,141.598636388779));
#41544=CARTESIAN_POINT('Ctrl Pts',(3.00102452933788,-8.9,141.598636388779));
#41545=CARTESIAN_POINT('Ctrl Pts',(3.57401113212109,-9.,142.171624183655));
#41546=CARTESIAN_POINT('Ctrl Pts',(3.57401113212109,-8.9,142.171624183655));
#41547=CARTESIAN_POINT('Ctrl Pts',(4.59679441154003,-9.,142.171624183655));
#41548=CARTESIAN_POINT('Ctrl Pts',(4.59679441154003,-8.9,142.171624183655));
#41549=CARTESIAN_POINT('',(3.00102452933788,-8.9,141.598636388779));
#41550=CARTESIAN_POINT('',(3.00102452933788,-9.,141.598636388779));
#41551=CARTESIAN_POINT('Ctrl Pts',(3.00102452933788,-8.9,141.598636388779));
#41552=CARTESIAN_POINT('Ctrl Pts',(3.57401113212109,-8.9,142.171624183655));
#41553=CARTESIAN_POINT('Ctrl Pts',(4.59679441154003,-8.9,142.171624183655));
#41554=CARTESIAN_POINT('Ctrl Pts',(2.42803601920605,-9.,139.997135639191));
#41555=CARTESIAN_POINT('Ctrl Pts',(2.42803601920605,-8.9,139.997135639191));
#41556=CARTESIAN_POINT('Ctrl Pts',(2.42803601920605,-9.,141.025648593903));
#41557=CARTESIAN_POINT('Ctrl Pts',(2.42803601920605,-8.9,141.025648593903));
#41558=CARTESIAN_POINT('Ctrl Pts',(3.00102452933788,-9.,141.598636388779));
#41559=CARTESIAN_POINT('Ctrl Pts',(3.00102452933788,-8.9,141.598636388779));
#41560=CARTESIAN_POINT('',(2.42803601920605,-8.9,139.997135639191));
#41561=CARTESIAN_POINT('',(2.42803601920605,-9.,139.997135639191));
#41562=CARTESIAN_POINT('Ctrl Pts',(2.42803601920605,-8.9,139.997135639191));
#41563=CARTESIAN_POINT('Ctrl Pts',(2.42803601920605,-8.9,141.025648593903));
#41564=CARTESIAN_POINT('Ctrl Pts',(3.00102452933788,-8.9,141.598636388779));
#41565=CARTESIAN_POINT('Ctrl Pts',(2.71739415824413,-9.,138.770942211151));
#41566=CARTESIAN_POINT('Ctrl Pts',(2.71739415824413,-8.9,138.770942211151));
#41567=CARTESIAN_POINT('Ctrl Pts',(2.42803601920605,-9.,139.260846614838));
#41568=CARTESIAN_POINT('Ctrl Pts',(2.42803601920605,-8.9,139.260846614838));
#41569=CARTESIAN_POINT('Ctrl Pts',(2.42803601920605,-9.,139.997135639191));
#41570=CARTESIAN_POINT('Ctrl Pts',(2.42803601920605,-8.9,139.997135639191));
#41571=CARTESIAN_POINT('Ctrl Pts',(2.71739415824413,-8.9,138.770942211151));
#41572=CARTESIAN_POINT('Ctrl Pts',(2.42803601920605,-8.9,139.260846614838));
#41573=CARTESIAN_POINT('Ctrl Pts',(2.42803601920605,-8.9,139.997135639191));
#41574=CARTESIAN_POINT('Origin',(4.60395650565624,-8.9,140.000000715256));
#41575=CARTESIAN_POINT('Origin',(-0.41684789955616,-9.,141.062892436981));
#41576=CARTESIAN_POINT('',(-0.41684789955616,-8.9,141.062892436981));
#41577=CARTESIAN_POINT('',(-0.41684789955616,-9.,141.062892436981));
#41578=CARTESIAN_POINT('',(-1.74044962227345,-8.9,141.062892436981));
#41579=CARTESIAN_POINT('',(-0.41684789955616,-8.9,141.062892436981));
#41580=CARTESIAN_POINT('',(-1.74044962227345,-9.,141.062892436981));
#41581=CARTESIAN_POINT('Origin',(-0.41684789955616,-9.,137.900000572205));
#41582=CARTESIAN_POINT('',(-0.41684789955616,-8.9,137.900000572205));
#41583=CARTESIAN_POINT('',(-0.41684789955616,-9.,137.900000572205));
#41584=CARTESIAN_POINT('',(-0.41684789955616,-8.9,137.900000572205));
#41585=CARTESIAN_POINT('Origin',(0.880968376994133,-9.,137.900000572205));
#41586=CARTESIAN_POINT('',(0.880968376994133,-8.9,137.900000572205));
#41587=CARTESIAN_POINT('',(0.880968376994133,-9.,137.900000572205));
#41588=CARTESIAN_POINT('',(0.880968376994133,-8.9,137.900000572205));
#41589=CARTESIAN_POINT('Origin',(0.880968376994133,-9.,141.062892436981));
#41590=CARTESIAN_POINT('',(0.880968376994133,-8.9,141.062892436981));
#41591=CARTESIAN_POINT('',(0.880968376994133,-9.,141.062892436981));
#41592=CARTESIAN_POINT('',(0.880968376994133,-8.9,141.062892436981));
#41593=CARTESIAN_POINT('Origin',(2.20457105338573,-9.,141.062892436981));
#41594=CARTESIAN_POINT('',(2.20457105338573,-8.9,141.062892436981));
#41595=CARTESIAN_POINT('',(2.20457105338573,-9.,141.062892436981));
#41596=CARTESIAN_POINT('',(2.20457105338573,-8.9,141.062892436981));
#41597=CARTESIAN_POINT('Origin',(2.20457105338573,-9.,142.10000038147));
#41598=CARTESIAN_POINT('',(2.20457105338573,-8.9,142.10000038147));
#41599=CARTESIAN_POINT('',(2.20457105338573,-9.,142.10000038147));
#41600=CARTESIAN_POINT('',(2.20457105338573,-8.9,142.10000038147));
#41601=CARTESIAN_POINT('Origin',(-1.74044962227345,-9.,142.10000038147));
#41602=CARTESIAN_POINT('',(-1.74044962227345,-8.9,142.10000038147));
#41603=CARTESIAN_POINT('',(-1.74044962227345,-9.,142.10000038147));
#41604=CARTESIAN_POINT('',(-1.74044962227345,-8.9,142.10000038147));
#41605=CARTESIAN_POINT('Origin',(-1.74044962227345,-9.,141.062892436981));
#41606=CARTESIAN_POINT('',(-1.74044962227345,-8.9,141.062892436981));
#41607=CARTESIAN_POINT('Origin',(0.232060715556145,-8.9,140.000000476837));
#41608=CARTESIAN_POINT('Ctrl Pts',(-5.37462396919727,-9.,141.10729932785));
#41609=CARTESIAN_POINT('Ctrl Pts',(-5.37462396919727,-8.9,141.10729932785));
#41610=CARTESIAN_POINT('Ctrl Pts',(-5.51643820106983,-9.,141.395225763321));
#41611=CARTESIAN_POINT('Ctrl Pts',(-5.51643820106983,-8.9,141.395225763321));
#41612=CARTESIAN_POINT('Ctrl Pts',(-5.80006761848927,-9.,141.395225763321));
#41613=CARTESIAN_POINT('Ctrl Pts',(-5.80006761848927,-8.9,141.395225763321));
#41614=CARTESIAN_POINT('',(-5.37462396919727,-9.,141.10729932785));
#41615=CARTESIAN_POINT('',(-5.80006761848927,-9.,141.395225763321));
#41616=CARTESIAN_POINT('Ctrl Pts',(-5.37462396919727,-9.,141.10729932785));
#41617=CARTESIAN_POINT('Ctrl Pts',(-5.51643820106983,-9.,141.395225763321));
#41618=CARTESIAN_POINT('Ctrl Pts',(-5.80006761848927,-9.,141.395225763321));
#41619=CARTESIAN_POINT('',(-5.37462396919727,-8.9,141.10729932785));
#41620=CARTESIAN_POINT('',(-5.37462396919727,-9.,141.10729932785));
#41621=CARTESIAN_POINT('',(-5.80006761848927,-8.9,141.395225763321));
#41622=CARTESIAN_POINT('Ctrl Pts',(-5.37462396919727,-8.9,141.10729932785));
#41623=CARTESIAN_POINT('Ctrl Pts',(-5.51643820106983,-8.9,141.395225763321));
#41624=CARTESIAN_POINT('Ctrl Pts',(-5.80006761848927,-8.9,141.395225763321));
#41625=CARTESIAN_POINT('',(-5.80006761848927,-9.,141.395225763321));
#41626=CARTESIAN_POINT('Ctrl Pts',(-5.23280973732471,-9.,139.982810974121));
#41627=CARTESIAN_POINT('Ctrl Pts',(-5.23280973732471,-8.9,139.982810974121));
#41628=CARTESIAN_POINT('Ctrl Pts',(-5.23280973732471,-9.,140.819372653961));
#41629=CARTESIAN_POINT('Ctrl Pts',(-5.23280973732471,-8.9,140.819372653961));
#41630=CARTESIAN_POINT('Ctrl Pts',(-5.37462396919727,-9.,141.10729932785));
#41631=CARTESIAN_POINT('Ctrl Pts',(-5.37462396919727,-8.9,141.10729932785));
#41632=CARTESIAN_POINT('',(-5.23280973732471,-9.,139.982810974121));
#41633=CARTESIAN_POINT('Ctrl Pts',(-5.23280973732471,-9.,139.982810974121));
#41634=CARTESIAN_POINT('Ctrl Pts',(-5.23280973732471,-9.,140.819372653961));
#41635=CARTESIAN_POINT('Ctrl Pts',(-5.37462396919727,-9.,141.10729932785));
#41636=CARTESIAN_POINT('',(-5.23280973732471,-8.9,139.982810974121));
#41637=CARTESIAN_POINT('',(-5.23280973732471,-9.,139.982810974121));
#41638=CARTESIAN_POINT('Ctrl Pts',(-5.23280973732471,-8.9,139.982810974121));
#41639=CARTESIAN_POINT('Ctrl Pts',(-5.23280973732471,-8.9,140.819372653961));
#41640=CARTESIAN_POINT('Ctrl Pts',(-5.37462396919727,-8.9,141.10729932785));
#41641=CARTESIAN_POINT('Ctrl Pts',(-5.29440565407276,-9.,139.143383979797));
#41642=CARTESIAN_POINT('Ctrl Pts',(-5.29440565407276,-8.9,139.143383979797));
#41643=CARTESIAN_POINT('Ctrl Pts',(-5.23280973732471,-9.,139.41268825531));
#41644=CARTESIAN_POINT('Ctrl Pts',(-5.23280973732471,-8.9,139.41268825531));
#41645=CARTESIAN_POINT('Ctrl Pts',(-5.23280973732471,-9.,139.982810974121));
#41646=CARTESIAN_POINT('Ctrl Pts',(-5.23280973732471,-8.9,139.982810974121));
#41647=CARTESIAN_POINT('',(-5.29440565407276,-9.,139.143383979797));
#41648=CARTESIAN_POINT('Ctrl Pts',(-5.29440565407276,-9.,139.143383979797));
#41649=CARTESIAN_POINT('Ctrl Pts',(-5.23280973732471,-9.,139.41268825531));
#41650=CARTESIAN_POINT('Ctrl Pts',(-5.23280973732471,-9.,139.982810974121));
#41651=CARTESIAN_POINT('',(-5.29440565407276,-8.9,139.143383979797));
#41652=CARTESIAN_POINT('',(-5.29440565407276,-9.,139.143383979797));
#41653=CARTESIAN_POINT('Ctrl Pts',(-5.29440565407276,-8.9,139.143383979797));
#41654=CARTESIAN_POINT('Ctrl Pts',(-5.23280973732471,-8.9,139.41268825531));
#41655=CARTESIAN_POINT('Ctrl Pts',(-5.23280973732471,-8.9,139.982810974121));
#41656=CARTESIAN_POINT('Ctrl Pts',(-5.48635645210743,-9.,138.749454975128));
#41657=CARTESIAN_POINT('Ctrl Pts',(-5.48635645210743,-8.9,138.749454975128));
#41658=CARTESIAN_POINT('Ctrl Pts',(-5.35600157082081,-9.,138.874079704285));
#41659=CARTESIAN_POINT('Ctrl Pts',(-5.35600157082081,-8.9,138.874079704285));
#41660=CARTESIAN_POINT('Ctrl Pts',(-5.29440565407276,-9.,139.143383979797));
#41661=CARTESIAN_POINT('Ctrl Pts',(-5.29440565407276,-8.9,139.143383979797));
#41662=CARTESIAN_POINT('',(-5.48635645210743,-9.,138.749454975128));
#41663=CARTESIAN_POINT('Ctrl Pts',(-5.48635645210743,-9.,138.749454975128));
#41664=CARTESIAN_POINT('Ctrl Pts',(-5.35600157082081,-9.,138.874079704285));
#41665=CARTESIAN_POINT('Ctrl Pts',(-5.29440565407276,-9.,139.143383979797));
#41666=CARTESIAN_POINT('',(-5.48635645210743,-8.9,138.749454975128));
#41667=CARTESIAN_POINT('',(-5.48635645210743,-9.,138.749454975128));
#41668=CARTESIAN_POINT('Ctrl Pts',(-5.48635645210743,-8.9,138.749454975128));
#41669=CARTESIAN_POINT('Ctrl Pts',(-5.35600157082081,-8.9,138.874079704285));
#41670=CARTESIAN_POINT('Ctrl Pts',(-5.29440565407276,-8.9,139.143383979797));
#41671=CARTESIAN_POINT('Ctrl Pts',(-5.7943379431963,-9.,138.624830245972));
#41672=CARTESIAN_POINT('Ctrl Pts',(-5.7943379431963,-8.9,138.624830245972));
#41673=CARTESIAN_POINT('Ctrl Pts',(-5.61671133339405,-9.,138.624830245972));
#41674=CARTESIAN_POINT('Ctrl Pts',(-5.61671133339405,-8.9,138.624830245972));
#41675=CARTESIAN_POINT('Ctrl Pts',(-5.48635645210743,-9.,138.749454975128));
#41676=CARTESIAN_POINT('Ctrl Pts',(-5.48635645210743,-8.9,138.749454975128));
#41677=CARTESIAN_POINT('',(-5.7943379431963,-9.,138.624830245972));
#41678=CARTESIAN_POINT('Ctrl Pts',(-5.7943379431963,-9.,138.624830245972));
#41679=CARTESIAN_POINT('Ctrl Pts',(-5.61671133339405,-9.,138.624830245972));
#41680=CARTESIAN_POINT('Ctrl Pts',(-5.48635645210743,-9.,138.749454975128));
#41681=CARTESIAN_POINT('',(-5.7943379431963,-8.9,138.624830245972));
#41682=CARTESIAN_POINT('',(-5.7943379431963,-9.,138.624830245972));
#41683=CARTESIAN_POINT('Ctrl Pts',(-5.7943379431963,-8.9,138.624830245972));
#41684=CARTESIAN_POINT('Ctrl Pts',(-5.61671133339405,-8.9,138.624830245972));
#41685=CARTESIAN_POINT('Ctrl Pts',(-5.48635645210743,-8.9,138.749454975128));
#41686=CARTESIAN_POINT('Ctrl Pts',(-6.20545549690723,-9.,138.918486118317));
#41687=CARTESIAN_POINT('Ctrl Pts',(-6.20545549690723,-8.9,138.918486118317));
#41688=CARTESIAN_POINT('Ctrl Pts',(-6.06364221870899,-9.,138.624830245972));
#41689=CARTESIAN_POINT('Ctrl Pts',(-6.06364221870899,-8.9,138.624830245972));
#41690=CARTESIAN_POINT('Ctrl Pts',(-5.7943379431963,-9.,138.624830245972));
#41691=CARTESIAN_POINT('Ctrl Pts',(-5.7943379431963,-8.9,138.624830245972));
#41692=CARTESIAN_POINT('',(-6.20545549690723,-9.,138.918486118317));
#41693=CARTESIAN_POINT('Ctrl Pts',(-6.20545549690723,-9.,138.918486118317));
#41694=CARTESIAN_POINT('Ctrl Pts',(-6.06364221870899,-9.,138.624830245972));
#41695=CARTESIAN_POINT('Ctrl Pts',(-5.7943379431963,-9.,138.624830245972));
#41696=CARTESIAN_POINT('',(-6.20545549690723,-8.9,138.918486118317));
#41697=CARTESIAN_POINT('',(-6.20545549690723,-9.,138.918486118317));
#41698=CARTESIAN_POINT('Ctrl Pts',(-6.20545549690723,-8.9,138.918486118317));
#41699=CARTESIAN_POINT('Ctrl Pts',(-6.06364221870899,-8.9,138.624830245972));
#41700=CARTESIAN_POINT('Ctrl Pts',(-5.7943379431963,-8.9,138.624830245972));
#41701=CARTESIAN_POINT('Ctrl Pts',(-6.34727068245411,-9.,140.014325141907));
#41702=CARTESIAN_POINT('Ctrl Pts',(-6.34727068245411,-8.9,140.014325141907));
#41703=CARTESIAN_POINT('Ctrl Pts',(-6.34727068245411,-9.,139.212142467499));
#41704=CARTESIAN_POINT('Ctrl Pts',(-6.34727068245411,-8.9,139.212142467499));
#41705=CARTESIAN_POINT('Ctrl Pts',(-6.20545549690723,-9.,138.918486118317));
#41706=CARTESIAN_POINT('Ctrl Pts',(-6.20545549690723,-8.9,138.918486118317));
#41707=CARTESIAN_POINT('',(-6.34727068245411,-9.,140.014325141907));
#41708=CARTESIAN_POINT('Ctrl Pts',(-6.34727068245411,-9.,140.014325141907));
#41709=CARTESIAN_POINT('Ctrl Pts',(-6.34727068245411,-9.,139.212142467499));
#41710=CARTESIAN_POINT('Ctrl Pts',(-6.20545549690723,-9.,138.918486118317));
#41711=CARTESIAN_POINT('',(-6.34727068245411,-8.9,140.014325141907));
#41712=CARTESIAN_POINT('',(-6.34727068245411,-9.,140.014325141907));
#41713=CARTESIAN_POINT('Ctrl Pts',(-6.34727068245411,-8.9,140.014325141907));
#41714=CARTESIAN_POINT('Ctrl Pts',(-6.34727068245411,-8.9,139.212142467499));
#41715=CARTESIAN_POINT('Ctrl Pts',(-6.20545549690723,-8.9,138.918486118317));
#41716=CARTESIAN_POINT('Ctrl Pts',(-6.21834821999073,-9.,141.101569652557));
#41717=CARTESIAN_POINT('Ctrl Pts',(-6.21834821999073,-8.9,141.101569652557));
#41718=CARTESIAN_POINT('Ctrl Pts',(-6.34727068245411,-9.,140.807913303375));
#41719=CARTESIAN_POINT('Ctrl Pts',(-6.34727068245411,-8.9,140.807913303375));
#41720=CARTESIAN_POINT('Ctrl Pts',(-6.34727068245411,-9.,140.014325141907));
#41721=CARTESIAN_POINT('Ctrl Pts',(-6.34727068245411,-8.9,140.014325141907));
#41722=CARTESIAN_POINT('',(-6.21834821999073,-9.,141.101569652557));
#41723=CARTESIAN_POINT('Ctrl Pts',(-6.21834821999073,-9.,141.101569652557));
#41724=CARTESIAN_POINT('Ctrl Pts',(-6.34727068245411,-9.,140.807913303375));
#41725=CARTESIAN_POINT('Ctrl Pts',(-6.34727068245411,-9.,140.014325141907));
#41726=CARTESIAN_POINT('',(-6.21834821999073,-8.9,141.101569652557));
#41727=CARTESIAN_POINT('',(-6.21834821999073,-9.,141.101569652557));
#41728=CARTESIAN_POINT('Ctrl Pts',(-6.21834821999073,-8.9,141.101569652557));
#41729=CARTESIAN_POINT('Ctrl Pts',(-6.34727068245411,-8.9,140.807913303375));
#41730=CARTESIAN_POINT('Ctrl Pts',(-6.34727068245411,-8.9,140.014325141907));
#41731=CARTESIAN_POINT('Ctrl Pts',(-5.80006761848927,-9.,141.395225763321));
#41732=CARTESIAN_POINT('Ctrl Pts',(-5.80006761848927,-8.9,141.395225763321));
#41733=CARTESIAN_POINT('Ctrl Pts',(-6.08942575752735,-9.,141.395225763321));
#41734=CARTESIAN_POINT('Ctrl Pts',(-6.08942575752735,-8.9,141.395225763321));
#41735=CARTESIAN_POINT('Ctrl Pts',(-6.21834821999073,-9.,141.101569652557));
#41736=CARTESIAN_POINT('Ctrl Pts',(-6.21834821999073,-8.9,141.101569652557));
#41737=CARTESIAN_POINT('Ctrl Pts',(-5.80006761848927,-9.,141.395225763321));
#41738=CARTESIAN_POINT('Ctrl Pts',(-6.08942575752735,-9.,141.395225763321));
#41739=CARTESIAN_POINT('Ctrl Pts',(-6.21834821999073,-9.,141.101569652557));
#41740=CARTESIAN_POINT('Ctrl Pts',(-5.80006761848927,-8.9,141.395225763321));
#41741=CARTESIAN_POINT('Ctrl Pts',(-6.08942575752735,-8.9,141.395225763321));
#41742=CARTESIAN_POINT('Ctrl Pts',(-6.21834821999073,-8.9,141.101569652557));
#41743=CARTESIAN_POINT('Ctrl Pts',(-7.1838323622942,-9.,138.493042945862));
#41744=CARTESIAN_POINT('Ctrl Pts',(-7.1838323622942,-8.9,138.493042945862));
#41745=CARTESIAN_POINT('Ctrl Pts',(-7.33567447960377,-9.,138.725102901459));
#41746=CARTESIAN_POINT('Ctrl Pts',(-7.33567447960377,-8.9,138.725102901459));
#41747=CARTESIAN_POINT('Ctrl Pts',(-7.42019005119801,-9.,139.127626895905));
#41748=CARTESIAN_POINT('Ctrl Pts',(-7.42019005119801,-8.9,139.127626895905));
#41749=CARTESIAN_POINT('',(-7.1838323622942,-8.9,138.493042945862));
#41750=CARTESIAN_POINT('',(-7.1838323622942,-9.,138.493042945862));
#41751=CARTESIAN_POINT('',(-7.42019005119801,-8.9,139.127626895905));
#41752=CARTESIAN_POINT('Ctrl Pts',(-7.1838323622942,-8.9,138.493042945862));
#41753=CARTESIAN_POINT('Ctrl Pts',(-7.33567447960377,-8.9,138.725102901459));
#41754=CARTESIAN_POINT('Ctrl Pts',(-7.42019005119801,-8.9,139.127626895905));
#41755=CARTESIAN_POINT('',(-7.42019005119801,-9.,139.127626895905));
#41756=CARTESIAN_POINT('Ctrl Pts',(-6.64808912575245,-9.,137.997408390045));
#41757=CARTESIAN_POINT('Ctrl Pts',(-6.64808912575245,-8.9,137.997408390045));
#41758=CARTESIAN_POINT('Ctrl Pts',(-6.97469206154346,-9.,138.166440010071));
#41759=CARTESIAN_POINT('Ctrl Pts',(-6.97469206154346,-8.9,138.166440010071));
#41760=CARTESIAN_POINT('Ctrl Pts',(-7.1838323622942,-9.,138.493042945862));
#41761=CARTESIAN_POINT('Ctrl Pts',(-7.1838323622942,-8.9,138.493042945862));
#41762=CARTESIAN_POINT('',(-6.64808912575245,-8.9,137.997408390045));
#41763=CARTESIAN_POINT('',(-6.64808912575245,-9.,137.997408390045));
#41764=CARTESIAN_POINT('Ctrl Pts',(-6.64808912575245,-8.9,137.997408390045));
#41765=CARTESIAN_POINT('Ctrl Pts',(-6.97469206154346,-8.9,138.166440010071));
#41766=CARTESIAN_POINT('Ctrl Pts',(-7.1838323622942,-8.9,138.493042945862));
#41767=CARTESIAN_POINT('Ctrl Pts',(-5.7914721518755,-9.,137.828377246857));
#41768=CARTESIAN_POINT('Ctrl Pts',(-5.7914721518755,-8.9,137.828377246857));
#41769=CARTESIAN_POINT('Ctrl Pts',(-6.32148618996143,-9.,137.828377246857));
#41770=CARTESIAN_POINT('Ctrl Pts',(-6.32148618996143,-8.9,137.828377246857));
#41771=CARTESIAN_POINT('Ctrl Pts',(-6.64808912575245,-9.,137.997408390045));
#41772=CARTESIAN_POINT('Ctrl Pts',(-6.64808912575245,-8.9,137.997408390045));
#41773=CARTESIAN_POINT('',(-5.7914721518755,-8.9,137.828377246857));
#41774=CARTESIAN_POINT('',(-5.7914721518755,-9.,137.828377246857));
#41775=CARTESIAN_POINT('Ctrl Pts',(-5.7914721518755,-8.9,137.828377246857));
#41776=CARTESIAN_POINT('Ctrl Pts',(-6.32148618996143,-8.9,137.828377246857));
#41777=CARTESIAN_POINT('Ctrl Pts',(-6.64808912575245,-8.9,137.997408390045));
#41778=CARTESIAN_POINT('Ctrl Pts',(-4.45927591621876,-9.,138.358390808105));
#41779=CARTESIAN_POINT('Ctrl Pts',(-4.45927591621876,-8.9,138.358390808105));
#41780=CARTESIAN_POINT('Ctrl Pts',(-4.84604234993458,-9.,137.828377246857));
#41781=CARTESIAN_POINT('Ctrl Pts',(-4.84604234993458,-8.9,137.828377246857));
#41782=CARTESIAN_POINT('Ctrl Pts',(-5.7914721518755,-9.,137.828377246857));
#41783=CARTESIAN_POINT('Ctrl Pts',(-5.7914721518755,-8.9,137.828377246857));
#41784=CARTESIAN_POINT('',(-4.45927591621876,-8.9,138.358390808105));
#41785=CARTESIAN_POINT('',(-4.45927591621876,-9.,138.358390808105));
#41786=CARTESIAN_POINT('Ctrl Pts',(-4.45927591621876,-8.9,138.358390808105));
#41787=CARTESIAN_POINT('Ctrl Pts',(-4.84604234993458,-8.9,137.828377246857));
#41788=CARTESIAN_POINT('Ctrl Pts',(-5.7914721518755,-8.9,137.828377246857));
#41789=CARTESIAN_POINT('Ctrl Pts',(-4.07250948250294,-9.,140.031514644623));
#41790=CARTESIAN_POINT('Ctrl Pts',(-4.07250948250294,-8.9,140.031514644623));
#41791=CARTESIAN_POINT('Ctrl Pts',(-4.07250948250294,-9.,138.888404369354));
#41792=CARTESIAN_POINT('Ctrl Pts',(-4.07250948250294,-8.9,138.888404369354));
#41793=CARTESIAN_POINT('Ctrl Pts',(-4.45927591621876,-9.,138.358390808105));
#41794=CARTESIAN_POINT('Ctrl Pts',(-4.45927591621876,-8.9,138.358390808105));
#41795=CARTESIAN_POINT('',(-4.07250948250294,-8.9,140.031514644623));
#41796=CARTESIAN_POINT('',(-4.07250948250294,-9.,140.031514644623));
#41797=CARTESIAN_POINT('Ctrl Pts',(-4.07250948250294,-8.9,140.031514644623));
#41798=CARTESIAN_POINT('Ctrl Pts',(-4.07250948250294,-8.9,138.888404369354));
#41799=CARTESIAN_POINT('Ctrl Pts',(-4.45927591621876,-8.9,138.358390808105));
#41800=CARTESIAN_POINT('Ctrl Pts',(-4.18997164070606,-9.,141.011323928833));
#41801=CARTESIAN_POINT('Ctrl Pts',(-4.18997164070606,-8.9,141.011323928833));
#41802=CARTESIAN_POINT('Ctrl Pts',(-4.07250948250294,-9.,140.541473865509));
#41803=CARTESIAN_POINT('Ctrl Pts',(-4.07250948250294,-8.9,140.541473865509));
#41804=CARTESIAN_POINT('Ctrl Pts',(-4.07250948250294,-9.,140.031514644623));
#41805=CARTESIAN_POINT('Ctrl Pts',(-4.07250948250294,-8.9,140.031514644623));
#41806=CARTESIAN_POINT('',(-4.18997164070606,-8.9,141.011323928833));
#41807=CARTESIAN_POINT('',(-4.18997164070606,-9.,141.011323928833));
#41808=CARTESIAN_POINT('Ctrl Pts',(-4.18997164070606,-8.9,141.011323928833));
#41809=CARTESIAN_POINT('Ctrl Pts',(-4.07250948250294,-8.9,140.541473865509));
#41810=CARTESIAN_POINT('Ctrl Pts',(-4.07250948250294,-8.9,140.031514644623));
#41811=CARTESIAN_POINT('Ctrl Pts',(-4.34897585213184,-9.,141.442497253418));
#41812=CARTESIAN_POINT('Ctrl Pts',(-4.34897585213184,-8.9,141.442497253418));
#41813=CARTESIAN_POINT('Ctrl Pts',(-4.25013513863087,-9.,141.2577085495));
#41814=CARTESIAN_POINT('Ctrl Pts',(-4.25013513863087,-8.9,141.2577085495));
#41815=CARTESIAN_POINT('Ctrl Pts',(-4.18997164070606,-9.,141.011323928833));
#41816=CARTESIAN_POINT('Ctrl Pts',(-4.18997164070606,-8.9,141.011323928833));
#41817=CARTESIAN_POINT('',(-4.34897585213184,-8.9,141.442497253418));
#41818=CARTESIAN_POINT('',(-4.34897585213184,-9.,141.442497253418));
#41819=CARTESIAN_POINT('Ctrl Pts',(-4.34897585213184,-8.9,141.442497253418));
#41820=CARTESIAN_POINT('Ctrl Pts',(-4.25013513863087,-8.9,141.2577085495));
#41821=CARTESIAN_POINT('Ctrl Pts',(-4.18997164070606,-8.9,141.011323928833));
#41822=CARTESIAN_POINT('Ctrl Pts',(-4.61971254646778,-9.,141.794884681702));
#41823=CARTESIAN_POINT('Ctrl Pts',(-4.61971254646778,-8.9,141.794884681702));
#41824=CARTESIAN_POINT('Ctrl Pts',(-4.44781656563282,-9.,141.627285718918));
#41825=CARTESIAN_POINT('Ctrl Pts',(-4.44781656563282,-8.9,141.627285718918));
#41826=CARTESIAN_POINT('Ctrl Pts',(-4.34897585213184,-9.,141.442497253418));
#41827=CARTESIAN_POINT('Ctrl Pts',(-4.34897585213184,-8.9,141.442497253418));
#41828=CARTESIAN_POINT('',(-4.61971254646778,-8.9,141.794884681702));
#41829=CARTESIAN_POINT('',(-4.61971254646778,-9.,141.794884681702));
#41830=CARTESIAN_POINT('Ctrl Pts',(-4.61971254646778,-8.9,141.794884681702));
#41831=CARTESIAN_POINT('Ctrl Pts',(-4.44781656563282,-8.9,141.627285718918));
#41832=CARTESIAN_POINT('Ctrl Pts',(-4.34897585213184,-8.9,141.442497253418));
#41833=CARTESIAN_POINT('Ctrl Pts',(-5.06377764046192,-9.,142.067054271698));
#41834=CARTESIAN_POINT('Ctrl Pts',(-5.06377764046192,-8.9,142.067054271698));
#41835=CARTESIAN_POINT('Ctrl Pts',(-4.79160852730274,-9.,141.962483882904));
#41836=CARTESIAN_POINT('Ctrl Pts',(-4.79160852730274,-8.9,141.962483882904));
#41837=CARTESIAN_POINT('Ctrl Pts',(-4.61971254646778,-9.,141.794884681702));
#41838=CARTESIAN_POINT('Ctrl Pts',(-4.61971254646778,-8.9,141.794884681702));
#41839=CARTESIAN_POINT('',(-5.06377764046192,-8.9,142.067054271698));
#41840=CARTESIAN_POINT('',(-5.06377764046192,-9.,142.067054271698));
#41841=CARTESIAN_POINT('Ctrl Pts',(-5.06377764046192,-8.9,142.067054271698));
#41842=CARTESIAN_POINT('Ctrl Pts',(-4.79160852730274,-8.9,141.962483882904));
#41843=CARTESIAN_POINT('Ctrl Pts',(-4.61971254646778,-8.9,141.794884681702));
#41844=CARTESIAN_POINT('Ctrl Pts',(-5.75995798408985,-9.,142.171624183655));
#41845=CARTESIAN_POINT('Ctrl Pts',(-5.75995798408985,-8.9,142.171624183655));
#41846=CARTESIAN_POINT('Ctrl Pts',(-5.3359467536211,-9.,142.171624183655));
#41847=CARTESIAN_POINT('Ctrl Pts',(-5.3359467536211,-8.9,142.171624183655));
#41848=CARTESIAN_POINT('Ctrl Pts',(-5.06377764046192,-9.,142.067054271698));
#41849=CARTESIAN_POINT('Ctrl Pts',(-5.06377764046192,-8.9,142.067054271698));
#41850=CARTESIAN_POINT('',(-5.75995798408985,-8.9,142.171624183655));
#41851=CARTESIAN_POINT('',(-5.75995798408985,-9.,142.171624183655));
#41852=CARTESIAN_POINT('Ctrl Pts',(-5.75995798408985,-8.9,142.171624183655));
#41853=CARTESIAN_POINT('Ctrl Pts',(-5.3359467536211,-8.9,142.171624183655));
#41854=CARTESIAN_POINT('Ctrl Pts',(-5.06377764046192,-8.9,142.067054271698));
#41855=CARTESIAN_POINT('Ctrl Pts',(-7.07353182137012,-9.,141.693179368973));
#41856=CARTESIAN_POINT('Ctrl Pts',(-7.07353182137012,-8.9,141.693179368973));
#41857=CARTESIAN_POINT('Ctrl Pts',(-6.64235849678516,-9.,142.171624183655));
#41858=CARTESIAN_POINT('Ctrl Pts',(-6.64235849678516,-8.9,142.171624183655));
#41859=CARTESIAN_POINT('Ctrl Pts',(-5.75995798408985,-9.,142.171624183655));
#41860=CARTESIAN_POINT('Ctrl Pts',(-5.75995798408985,-8.9,142.171624183655));
#41861=CARTESIAN_POINT('',(-7.07353182137012,-8.9,141.693179368973));
#41862=CARTESIAN_POINT('',(-7.07353182137012,-9.,141.693179368973));
#41863=CARTESIAN_POINT('Ctrl Pts',(-7.07353182137012,-8.9,141.693179368973));
#41864=CARTESIAN_POINT('Ctrl Pts',(-6.64235849678516,-8.9,142.171624183655));
#41865=CARTESIAN_POINT('Ctrl Pts',(-5.75995798408985,-8.9,142.171624183655));
#41866=CARTESIAN_POINT('Ctrl Pts',(-7.50470562279224,-9.,140.01719045639));
#41867=CARTESIAN_POINT('Ctrl Pts',(-7.50470562279224,-8.9,140.01719045639));
#41868=CARTESIAN_POINT('Ctrl Pts',(-7.50470562279224,-9.,141.214734554291));
#41869=CARTESIAN_POINT('Ctrl Pts',(-7.50470562279224,-8.9,141.214734554291));
#41870=CARTESIAN_POINT('Ctrl Pts',(-7.07353182137012,-9.,141.693179368973));
#41871=CARTESIAN_POINT('Ctrl Pts',(-7.07353182137012,-8.9,141.693179368973));
#41872=CARTESIAN_POINT('',(-7.50470562279224,-8.9,140.01719045639));
#41873=CARTESIAN_POINT('',(-7.50470562279224,-9.,140.01719045639));
#41874=CARTESIAN_POINT('Ctrl Pts',(-7.50470562279224,-8.9,140.01719045639));
#41875=CARTESIAN_POINT('Ctrl Pts',(-7.50470562279224,-8.9,141.214734554291));
#41876=CARTESIAN_POINT('Ctrl Pts',(-7.07353182137012,-8.9,141.693179368973));
#41877=CARTESIAN_POINT('Ctrl Pts',(-7.42019005119801,-9.,139.127626895905));
#41878=CARTESIAN_POINT('Ctrl Pts',(-7.42019005119801,-8.9,139.127626895905));
#41879=CARTESIAN_POINT('Ctrl Pts',(-7.50470562279224,-9.,139.53015089035));
#41880=CARTESIAN_POINT('Ctrl Pts',(-7.50470562279224,-8.9,139.53015089035));
#41881=CARTESIAN_POINT('Ctrl Pts',(-7.50470562279224,-9.,140.01719045639));
#41882=CARTESIAN_POINT('Ctrl Pts',(-7.50470562279224,-8.9,140.01719045639));
#41883=CARTESIAN_POINT('Ctrl Pts',(-7.42019005119801,-8.9,139.127626895905));
#41884=CARTESIAN_POINT('Ctrl Pts',(-7.50470562279224,-8.9,139.53015089035));
#41885=CARTESIAN_POINT('Ctrl Pts',(-7.50470562279224,-8.9,140.01719045639));
#41886=CARTESIAN_POINT('Origin',(-5.78860755264759,-8.9,140.000000715256));
#41887=CARTESIAN_POINT('Origin',(-9.82530565559864,-9.,138.851160049438));
#41888=CARTESIAN_POINT('',(-9.82530565559864,-8.9,138.851160049438));
#41889=CARTESIAN_POINT('',(-9.82530565559864,-9.,138.851160049438));
#41890=CARTESIAN_POINT('',(-8.00320501625538,-8.9,138.851160049438));
#41891=CARTESIAN_POINT('',(-9.82530565559864,-8.9,138.851160049438));
#41892=CARTESIAN_POINT('',(-8.00320501625538,-9.,138.851160049438));
#41893=CARTESIAN_POINT('Ctrl Pts',(-9.54597444832325,-9.,139.106139659882));
#41894=CARTESIAN_POINT('Ctrl Pts',(-9.54597444832325,-8.9,139.106139659882));
#41895=CARTESIAN_POINT('Ctrl Pts',(-9.66486950218678,-9.,139.008731842041));
#41896=CARTESIAN_POINT('Ctrl Pts',(-9.66486950218678,-8.9,139.008731842041));
#41897=CARTESIAN_POINT('Ctrl Pts',(-9.82530565559864,-9.,138.851160049438));
#41898=CARTESIAN_POINT('Ctrl Pts',(-9.82530565559864,-8.9,138.851160049438));
#41899=CARTESIAN_POINT('',(-9.54597444832325,-8.9,139.106139659882));
#41900=CARTESIAN_POINT('',(-9.54597444832325,-9.,139.106139659882));
#41901=CARTESIAN_POINT('Ctrl Pts',(-9.54597444832325,-8.9,139.106139659882));
#41902=CARTESIAN_POINT('Ctrl Pts',(-9.66486950218678,-8.9,139.008731842041));
#41903=CARTESIAN_POINT('Ctrl Pts',(-9.82530565559864,-8.9,138.851160049438));
#41904=CARTESIAN_POINT('Ctrl Pts',(-9.07469196617603,-9.,139.447067260742));
#41905=CARTESIAN_POINT('Ctrl Pts',(-9.07469196617603,-8.9,139.447067260742));
#41906=CARTESIAN_POINT('Ctrl Pts',(-9.42707939445972,-9.,139.203547477722));
#41907=CARTESIAN_POINT('Ctrl Pts',(-9.42707939445972,-8.9,139.203547477722));
#41908=CARTESIAN_POINT('Ctrl Pts',(-9.54597444832325,-9.,139.106139659882));
#41909=CARTESIAN_POINT('Ctrl Pts',(-9.54597444832325,-8.9,139.106139659882));
#41910=CARTESIAN_POINT('',(-9.07469196617603,-8.9,139.447067260742));
#41911=CARTESIAN_POINT('',(-9.07469196617603,-9.,139.447067260742));
#41912=CARTESIAN_POINT('Ctrl Pts',(-9.07469196617603,-8.9,139.447067260742));
#41913=CARTESIAN_POINT('Ctrl Pts',(-9.42707939445972,-8.9,139.203547477722));
#41914=CARTESIAN_POINT('Ctrl Pts',(-9.54597444832325,-8.9,139.106139659882));
#41915=CARTESIAN_POINT('Ctrl Pts',(-8.25675220787525,-9.,140.214870929718));
#41916=CARTESIAN_POINT('Ctrl Pts',(-8.25675220787525,-8.9,140.214870929718));
#41917=CARTESIAN_POINT('Ctrl Pts',(-8.48165006935596,-9.,139.865348339081));
#41918=CARTESIAN_POINT('Ctrl Pts',(-8.48165006935596,-8.9,139.865348339081));
#41919=CARTESIAN_POINT('Ctrl Pts',(-9.07469196617603,-9.,139.447067260742));
#41920=CARTESIAN_POINT('Ctrl Pts',(-9.07469196617603,-8.9,139.447067260742));
#41921=CARTESIAN_POINT('',(-8.25675220787525,-8.9,140.214870929718));
#41922=CARTESIAN_POINT('',(-8.25675220787525,-9.,140.214870929718));
#41923=CARTESIAN_POINT('Ctrl Pts',(-8.25675220787525,-8.9,140.214870929718));
#41924=CARTESIAN_POINT('Ctrl Pts',(-8.48165006935596,-8.9,139.865348339081));
#41925=CARTESIAN_POINT('Ctrl Pts',(-9.07469196617603,-8.9,139.447067260742));
#41926=CARTESIAN_POINT('Ctrl Pts',(-8.03185434639454,-9.,140.948295116425));
#41927=CARTESIAN_POINT('Ctrl Pts',(-8.03185434639454,-8.9,140.948295116425));
#41928=CARTESIAN_POINT('Ctrl Pts',(-8.03185434639454,-9.,140.564393520355));
#41929=CARTESIAN_POINT('Ctrl Pts',(-8.03185434639454,-8.9,140.564393520355));
#41930=CARTESIAN_POINT('Ctrl Pts',(-8.25675220787525,-9.,140.214870929718));
#41931=CARTESIAN_POINT('Ctrl Pts',(-8.25675220787525,-8.9,140.214870929718));
#41932=CARTESIAN_POINT('',(-8.03185434639454,-8.9,140.948295116425));
#41933=CARTESIAN_POINT('',(-8.03185434639454,-9.,140.948295116425));
#41934=CARTESIAN_POINT('Ctrl Pts',(-8.03185434639454,-8.9,140.948295116425));
#41935=CARTESIAN_POINT('Ctrl Pts',(-8.03185434639454,-8.9,140.564393520355));
#41936=CARTESIAN_POINT('Ctrl Pts',(-8.25675220787525,-8.9,140.214870929718));
#41937=CARTESIAN_POINT('Ctrl Pts',(-8.22810240089893,-9.,141.600068569183));
#41938=CARTESIAN_POINT('Ctrl Pts',(-8.22810240089893,-8.9,141.600068569183));
#41939=CARTESIAN_POINT('Ctrl Pts',(-8.03185434639454,-9.,141.309277296066));
#41940=CARTESIAN_POINT('Ctrl Pts',(-8.03185434639454,-8.9,141.309277296066));
#41941=CARTESIAN_POINT('Ctrl Pts',(-8.03185434639454,-9.,140.948295116425));
#41942=CARTESIAN_POINT('Ctrl Pts',(-8.03185434639454,-8.9,140.948295116425));
#41943=CARTESIAN_POINT('',(-8.22810240089893,-8.9,141.600068569183));
#41944=CARTESIAN_POINT('',(-8.22810240089893,-9.,141.600068569183));
#41945=CARTESIAN_POINT('Ctrl Pts',(-8.22810240089893,-8.9,141.600068569183));
#41946=CARTESIAN_POINT('Ctrl Pts',(-8.03185434639454,-8.9,141.309277296066));
#41947=CARTESIAN_POINT('Ctrl Pts',(-8.03185434639454,-8.9,140.948295116425));
#41948=CARTESIAN_POINT('Ctrl Pts',(-8.76671095192432,-9.,142.031241893768));
#41949=CARTESIAN_POINT('Ctrl Pts',(-8.76671095192432,-8.9,142.031241893768));
#41950=CARTESIAN_POINT('Ctrl Pts',(-8.42435093224049,-9.,141.8908598423));
#41951=CARTESIAN_POINT('Ctrl Pts',(-8.42435093224049,-8.9,141.8908598423));
#41952=CARTESIAN_POINT('Ctrl Pts',(-8.22810240089893,-9.,141.600068569183));
#41953=CARTESIAN_POINT('Ctrl Pts',(-8.22810240089893,-8.9,141.600068569183));
#41954=CARTESIAN_POINT('',(-8.76671095192432,-8.9,142.031241893768));
#41955=CARTESIAN_POINT('',(-8.76671095192432,-9.,142.031241893768));
#41956=CARTESIAN_POINT('Ctrl Pts',(-8.76671095192432,-8.9,142.031241893768));
#41957=CARTESIAN_POINT('Ctrl Pts',(-8.42435093224049,-8.9,141.8908598423));
#41958=CARTESIAN_POINT('Ctrl Pts',(-8.22810240089893,-8.9,141.600068569183));
#41959=CARTESIAN_POINT('Ctrl Pts',(-9.72503300011158,-9.,142.171623706818));
#41960=CARTESIAN_POINT('Ctrl Pts',(-9.72503300011158,-8.9,142.171623706818));
#41961=CARTESIAN_POINT('Ctrl Pts',(-9.10907144844532,-9.,142.171623706818));
#41962=CARTESIAN_POINT('Ctrl Pts',(-9.10907144844532,-8.9,142.171623706818));
#41963=CARTESIAN_POINT('Ctrl Pts',(-8.76671095192432,-9.,142.031241893768));
#41964=CARTESIAN_POINT('Ctrl Pts',(-8.76671095192432,-8.9,142.031241893768));
#41965=CARTESIAN_POINT('',(-9.72503300011158,-8.9,142.171623706818));
#41966=CARTESIAN_POINT('',(-9.72503300011158,-9.,142.171623706818));
#41967=CARTESIAN_POINT('Ctrl Pts',(-9.72503300011158,-8.9,142.171623706818));
#41968=CARTESIAN_POINT('Ctrl Pts',(-9.10907144844532,-8.9,142.171623706818));
#41969=CARTESIAN_POINT('Ctrl Pts',(-8.76671095192432,-8.9,142.031241893768));
#41970=CARTESIAN_POINT('Ctrl Pts',(-10.6489760428667,-9.,142.024079322815));
#41971=CARTESIAN_POINT('Ctrl Pts',(-10.6489760428667,-8.9,142.024079322815));
#41972=CARTESIAN_POINT('Ctrl Pts',(-10.3152105361223,-9.,142.171623706818));
#41973=CARTESIAN_POINT('Ctrl Pts',(-10.3152105361223,-8.9,142.171623706818));
#41974=CARTESIAN_POINT('Ctrl Pts',(-9.72503300011158,-9.,142.171623706818));
#41975=CARTESIAN_POINT('Ctrl Pts',(-9.72503300011158,-8.9,142.171623706818));
#41976=CARTESIAN_POINT('',(-10.6489760428667,-8.9,142.024079322815));
#41977=CARTESIAN_POINT('',(-10.6489760428667,-9.,142.024079322815));
#41978=CARTESIAN_POINT('Ctrl Pts',(-10.6489760428667,-8.9,142.024079322815));
#41979=CARTESIAN_POINT('Ctrl Pts',(-10.3152105361223,-8.9,142.171623706818));
#41980=CARTESIAN_POINT('Ctrl Pts',(-9.72503300011158,-8.9,142.171623706818));
#41981=CARTESIAN_POINT('Ctrl Pts',(-11.1660971194506,-9.,141.600068569183));
#41982=CARTESIAN_POINT('Ctrl Pts',(-11.1660971194506,-8.9,141.600068569183));
#41983=CARTESIAN_POINT('Ctrl Pts',(-10.9827410727739,-9.,141.876535177231));
#41984=CARTESIAN_POINT('Ctrl Pts',(-10.9827410727739,-8.9,141.876535177231));
#41985=CARTESIAN_POINT('Ctrl Pts',(-10.6489760428667,-9.,142.024079322815));
#41986=CARTESIAN_POINT('Ctrl Pts',(-10.6489760428667,-8.9,142.024079322815));
#41987=CARTESIAN_POINT('',(-11.1660971194506,-8.9,141.600068569183));
#41988=CARTESIAN_POINT('',(-11.1660971194506,-9.,141.600068569183));
#41989=CARTESIAN_POINT('Ctrl Pts',(-11.1660971194506,-8.9,141.600068569183));
#41990=CARTESIAN_POINT('Ctrl Pts',(-10.9827410727739,-8.9,141.876535177231));
#41991=CARTESIAN_POINT('Ctrl Pts',(-10.6489760428667,-8.9,142.024079322815));
#41992=CARTESIAN_POINT('Ctrl Pts',(-11.4182116538286,-9.,140.830832958221));
#41993=CARTESIAN_POINT('Ctrl Pts',(-11.4182116538286,-8.9,140.830832958221));
#41994=CARTESIAN_POINT('Ctrl Pts',(-11.3494531661272,-9.,141.323601961136));
#41995=CARTESIAN_POINT('Ctrl Pts',(-11.3494531661272,-8.9,141.323601961136));
#41996=CARTESIAN_POINT('Ctrl Pts',(-11.1660971194506,-9.,141.600068569183));
#41997=CARTESIAN_POINT('Ctrl Pts',(-11.1660971194506,-8.9,141.600068569183));
#41998=CARTESIAN_POINT('',(-11.4182116538286,-8.9,140.830832958221));
#41999=CARTESIAN_POINT('',(-11.4182116538286,-9.,140.830832958221));
#42000=CARTESIAN_POINT('Ctrl Pts',(-11.4182116538286,-8.9,140.830832958221));
#42001=CARTESIAN_POINT('Ctrl Pts',(-11.3494531661272,-8.9,141.323601961136));
#42002=CARTESIAN_POINT('Ctrl Pts',(-11.1660971194506,-8.9,141.600068569183));
#42003=CARTESIAN_POINT('Origin',(-10.2493168860674,-9.,140.73628950119));
#42004=CARTESIAN_POINT('',(-10.2493168860674,-8.9,140.73628950119));
#42005=CARTESIAN_POINT('',(-10.2493168860674,-9.,140.73628950119));
#42006=CARTESIAN_POINT('',(-10.2493168860674,-8.9,140.73628950119));
#42007=CARTESIAN_POINT('Ctrl Pts',(-10.058798506856,-9.,141.231924057007));
#42008=CARTESIAN_POINT('Ctrl Pts',(-10.058798506856,-8.9,141.231924057007));
#42009=CARTESIAN_POINT('Ctrl Pts',(-10.2006127387285,-9.,141.09154176712));
#42010=CARTESIAN_POINT('Ctrl Pts',(-10.2006127387285,-8.9,141.09154176712));
#42011=CARTESIAN_POINT('Ctrl Pts',(-10.2493168860674,-9.,140.73628950119));
#42012=CARTESIAN_POINT('Ctrl Pts',(-10.2493168860674,-8.9,140.73628950119));
#42013=CARTESIAN_POINT('',(-10.058798506856,-8.9,141.231924057007));
#42014=CARTESIAN_POINT('',(-10.058798506856,-9.,141.231924057007));
#42015=CARTESIAN_POINT('Ctrl Pts',(-10.058798506856,-8.9,141.231924057007));
#42016=CARTESIAN_POINT('Ctrl Pts',(-10.2006127387285,-8.9,141.09154176712));
#42017=CARTESIAN_POINT('Ctrl Pts',(-10.2493168860674,-8.9,140.73628950119));
#42018=CARTESIAN_POINT('Ctrl Pts',(-9.69351883232594,-9.,141.372305870056));
#42019=CARTESIAN_POINT('Ctrl Pts',(-9.69351883232594,-8.9,141.372305870056));
#42020=CARTESIAN_POINT('Ctrl Pts',(-9.91698379814625,-9.,141.372305870056));
#42021=CARTESIAN_POINT('Ctrl Pts',(-9.91698379814625,-8.9,141.372305870056));
#42022=CARTESIAN_POINT('Ctrl Pts',(-10.058798506856,-9.,141.231924057007));
#42023=CARTESIAN_POINT('Ctrl Pts',(-10.058798506856,-8.9,141.231924057007));
#42024=CARTESIAN_POINT('',(-9.69351883232594,-8.9,141.372305870056));
#42025=CARTESIAN_POINT('',(-9.69351883232594,-9.,141.372305870056));
#42026=CARTESIAN_POINT('Ctrl Pts',(-9.69351883232594,-8.9,141.372305870056));
#42027=CARTESIAN_POINT('Ctrl Pts',(-9.91698379814625,-8.9,141.372305870056));
#42028=CARTESIAN_POINT('Ctrl Pts',(-10.058798506856,-8.9,141.231924057007));
#42029=CARTESIAN_POINT('Ctrl Pts',(-9.33683367073536,-9.,141.236221313477));
#42030=CARTESIAN_POINT('Ctrl Pts',(-9.33683367073536,-8.9,141.236221313477));
#42031=CARTESIAN_POINT('Ctrl Pts',(-9.47864837944508,-9.,141.372305870056));
#42032=CARTESIAN_POINT('Ctrl Pts',(-9.47864837944508,-8.9,141.372305870056));
#42033=CARTESIAN_POINT('Ctrl Pts',(-9.69351883232594,-9.,141.372305870056));
#42034=CARTESIAN_POINT('Ctrl Pts',(-9.69351883232594,-8.9,141.372305870056));
#42035=CARTESIAN_POINT('',(-9.33683367073536,-8.9,141.236221313477));
#42036=CARTESIAN_POINT('',(-9.33683367073536,-9.,141.236221313477));
#42037=CARTESIAN_POINT('Ctrl Pts',(-9.33683367073536,-8.9,141.236221313477));
#42038=CARTESIAN_POINT('Ctrl Pts',(-9.47864837944508,-8.9,141.372305870056));
#42039=CARTESIAN_POINT('Ctrl Pts',(-9.69351883232594,-8.9,141.372305870056));
#42040=CARTESIAN_POINT('Ctrl Pts',(-9.1950194388628,-9.,140.908185958862));
#42041=CARTESIAN_POINT('Ctrl Pts',(-9.1950194388628,-8.9,140.908185958862));
#42042=CARTESIAN_POINT('Ctrl Pts',(-9.1950194388628,-9.,141.100136756897));
#42043=CARTESIAN_POINT('Ctrl Pts',(-9.1950194388628,-8.9,141.100136756897));
#42044=CARTESIAN_POINT('Ctrl Pts',(-9.33683367073536,-9.,141.236221313477));
#42045=CARTESIAN_POINT('Ctrl Pts',(-9.33683367073536,-8.9,141.236221313477));
#42046=CARTESIAN_POINT('',(-9.1950194388628,-8.9,140.908185958862));
#42047=CARTESIAN_POINT('',(-9.1950194388628,-9.,140.908185958862));
#42048=CARTESIAN_POINT('Ctrl Pts',(-9.1950194388628,-8.9,140.908185958862));
#42049=CARTESIAN_POINT('Ctrl Pts',(-9.1950194388628,-8.9,141.100136756897));
#42050=CARTESIAN_POINT('Ctrl Pts',(-9.33683367073536,-8.9,141.236221313477));
#42051=CARTESIAN_POINT('Ctrl Pts',(-9.3382660895586,-9.,140.53287935257));
#42052=CARTESIAN_POINT('Ctrl Pts',(-9.3382660895586,-8.9,140.53287935257));
#42053=CARTESIAN_POINT('Ctrl Pts',(-9.1950194388628,-9.,140.730559825897));
#42054=CARTESIAN_POINT('Ctrl Pts',(-9.1950194388628,-8.9,140.730559825897));
#42055=CARTESIAN_POINT('Ctrl Pts',(-9.1950194388628,-9.,140.908185958862));
#42056=CARTESIAN_POINT('Ctrl Pts',(-9.1950194388628,-8.9,140.908185958862));
#42057=CARTESIAN_POINT('',(-9.3382660895586,-8.9,140.53287935257));
#42058=CARTESIAN_POINT('',(-9.3382660895586,-9.,140.53287935257));
#42059=CARTESIAN_POINT('Ctrl Pts',(-9.3382660895586,-8.9,140.53287935257));
#42060=CARTESIAN_POINT('Ctrl Pts',(-9.1950194388628,-8.9,140.730559825897));
#42061=CARTESIAN_POINT('Ctrl Pts',(-9.1950194388628,-8.9,140.908185958862));
#42062=CARTESIAN_POINT('Ctrl Pts',(-9.99433727562428,-9.,139.954161167145));
#42063=CARTESIAN_POINT('Ctrl Pts',(-9.99433727562428,-8.9,139.954161167145));
#42064=CARTESIAN_POINT('Ctrl Pts',(-9.48151321709156,-9.,140.335197925568));
#42065=CARTESIAN_POINT('Ctrl Pts',(-9.48151321709156,-8.9,140.335197925568));
#42066=CARTESIAN_POINT('Ctrl Pts',(-9.3382660895586,-9.,140.53287935257));
#42067=CARTESIAN_POINT('Ctrl Pts',(-9.3382660895586,-8.9,140.53287935257));
#42068=CARTESIAN_POINT('',(-9.99433727562428,-8.9,139.954161167145));
#42069=CARTESIAN_POINT('',(-9.99433727562428,-9.,139.954161167145));
#42070=CARTESIAN_POINT('Ctrl Pts',(-9.99433727562428,-8.9,139.954161167145));
#42071=CARTESIAN_POINT('Ctrl Pts',(-9.48151321709156,-8.9,140.335197925568));
#42072=CARTESIAN_POINT('Ctrl Pts',(-9.3382660895586,-8.9,140.53287935257));
#42073=CARTESIAN_POINT('Ctrl Pts',(-11.1388804465532,-9.,138.875512123108));
#42074=CARTESIAN_POINT('Ctrl Pts',(-11.1388804465532,-8.9,138.875512123108));
#42075=CARTESIAN_POINT('Ctrl Pts',(-10.833764269948,-9.,139.332469940186));
#42076=CARTESIAN_POINT('Ctrl Pts',(-10.833764269948,-8.9,139.332469940186));
#42077=CARTESIAN_POINT('Ctrl Pts',(-9.99433727562428,-9.,139.954161167145));
#42078=CARTESIAN_POINT('Ctrl Pts',(-9.99433727562428,-8.9,139.954161167145));
#42079=CARTESIAN_POINT('',(-11.1388804465532,-8.9,138.875512123108));
#42080=CARTESIAN_POINT('',(-11.1388804465532,-9.,138.875512123108));
#42081=CARTESIAN_POINT('Ctrl Pts',(-11.1388804465532,-8.9,138.875512123108));
#42082=CARTESIAN_POINT('Ctrl Pts',(-10.833764269948,-8.9,139.332469940186));
#42083=CARTESIAN_POINT('Ctrl Pts',(-9.99433727562428,-8.9,139.954161167145));
#42084=CARTESIAN_POINT('Ctrl Pts',(-11.5041598826647,-9.,137.900000572205));
#42085=CARTESIAN_POINT('Ctrl Pts',(-11.5041598826647,-8.9,137.900000572205));
#42086=CARTESIAN_POINT('Ctrl Pts',(-11.4439961463213,-9.,138.41855430603));
#42087=CARTESIAN_POINT('Ctrl Pts',(-11.4439961463213,-8.9,138.41855430603));
#42088=CARTESIAN_POINT('Ctrl Pts',(-11.1388804465532,-9.,138.875512123108));
#42089=CARTESIAN_POINT('Ctrl Pts',(-11.1388804465532,-8.9,138.875512123108));
#42090=CARTESIAN_POINT('',(-11.5041598826647,-8.9,137.900000572205));
#42091=CARTESIAN_POINT('',(-11.5041598826647,-9.,137.900000572205));
#42092=CARTESIAN_POINT('Ctrl Pts',(-11.5041598826647,-8.9,137.900000572205));
#42093=CARTESIAN_POINT('Ctrl Pts',(-11.4439961463213,-8.9,138.41855430603));
#42094=CARTESIAN_POINT('Ctrl Pts',(-11.1388804465532,-8.9,138.875512123108));
#42095=CARTESIAN_POINT('Origin',(-8.00320501625538,-9.,137.900000572205));
#42096=CARTESIAN_POINT('',(-8.00320501625538,-8.9,137.900000572205));
#42097=CARTESIAN_POINT('',(-8.00320501625538,-9.,137.900000572205));
#42098=CARTESIAN_POINT('',(-8.00320501625538,-8.9,137.900000572205));
#42099=CARTESIAN_POINT('Origin',(-8.00320501625538,-9.,138.851160049438));
#42100=CARTESIAN_POINT('',(-8.00320501625538,-8.9,138.851160049438));
#42101=CARTESIAN_POINT('Origin',(-9.75368244946003,-8.9,140.035812139511));
#42102=CARTESIAN_POINT('Origin',(8.70797948539257,-9.,137.900000572205));
#42103=CARTESIAN_POINT('',(8.70797948539257,-8.9,137.900000572205));
#42104=CARTESIAN_POINT('',(8.70797948539257,-9.,137.900000572205));
#42105=CARTESIAN_POINT('',(7.4875166863203,-8.9,137.900000572205));
#42106=CARTESIAN_POINT('',(8.70797948539257,-8.9,137.900000572205));
#42107=CARTESIAN_POINT('',(7.4875166863203,-9.,137.900000572205));
#42108=CARTESIAN_POINT('Origin',(8.70797948539257,-9.,140.206097126007));
#42109=CARTESIAN_POINT('',(8.70797948539257,-8.9,140.206097126007));
#42110=CARTESIAN_POINT('',(8.70797948539257,-9.,140.206097126007));
#42111=CARTESIAN_POINT('',(8.70797948539257,-8.9,140.206097126007));
#42112=CARTESIAN_POINT('Origin',(10.2808306664228,-9.,137.900000572205));
#42113=CARTESIAN_POINT('',(10.2808306664228,-8.9,137.900000572205));
#42114=CARTESIAN_POINT('',(10.2808306664228,-9.,137.900000572205));
#42115=CARTESIAN_POINT('',(10.2808306664228,-8.9,137.900000572205));
#42116=CARTESIAN_POINT('Origin',(11.5041602104902,-9.,137.900000572205));
#42117=CARTESIAN_POINT('',(11.5041602104902,-8.9,137.900000572205));
#42118=CARTESIAN_POINT('',(11.5041602104902,-9.,137.900000572205));
#42119=CARTESIAN_POINT('',(11.5041602104902,-8.9,137.900000572205));
#42120=CARTESIAN_POINT('Origin',(11.5041602104902,-9.,142.10000038147));
#42121=CARTESIAN_POINT('',(11.5041602104902,-8.9,142.10000038147));
#42122=CARTESIAN_POINT('',(11.5041602104902,-9.,142.10000038147));
#42123=CARTESIAN_POINT('',(11.5041602104902,-8.9,142.10000038147));
#42124=CARTESIAN_POINT('Origin',(10.2808306664228,-9.,142.10000038147));
#42125=CARTESIAN_POINT('',(10.2808306664228,-8.9,142.10000038147));
#42126=CARTESIAN_POINT('',(10.2808306664228,-9.,142.10000038147));
#42127=CARTESIAN_POINT('',(10.2808306664228,-8.9,142.10000038147));
#42128=CARTESIAN_POINT('Origin',(10.2808306664228,-9.,139.776356220245));
#42129=CARTESIAN_POINT('',(10.2808306664228,-8.9,139.776356220245));
#42130=CARTESIAN_POINT('',(10.2808306664228,-9.,139.776356220245));
#42131=CARTESIAN_POINT('',(10.2808306664228,-8.9,139.776356220245));
#42132=CARTESIAN_POINT('Origin',(8.69938497245312,-9.,142.10000038147));
#42133=CARTESIAN_POINT('',(8.69938497245312,-8.9,142.10000038147));
#42134=CARTESIAN_POINT('',(8.69938497245312,-9.,142.10000038147));
#42135=CARTESIAN_POINT('',(8.69938497245312,-8.9,142.10000038147));
#42136=CARTESIAN_POINT('Origin',(7.4875166863203,-9.,142.10000038147));
#42137=CARTESIAN_POINT('',(7.4875166863203,-8.9,142.10000038147));
#42138=CARTESIAN_POINT('',(7.4875166863203,-9.,142.10000038147));
#42139=CARTESIAN_POINT('',(7.4875166863203,-8.9,142.10000038147));
#42140=CARTESIAN_POINT('Origin',(7.4875166863203,-9.,137.900000572205));
#42141=CARTESIAN_POINT('',(7.4875166863203,-8.9,137.900000572205));
#42142=CARTESIAN_POINT('Origin',(9.49583844840527,-8.9,140.000000476837));
#42143=CARTESIAN_POINT('Origin',(-38.,-9.,145.));
#42144=CARTESIAN_POINT('Origin',(-38.,-9.,145.));
#42145=CARTESIAN_POINT('Origin',(0.,0.,135.));
#42146=CARTESIAN_POINT('',(-25.8,9.,135.));
#42147=CARTESIAN_POINT('Origin',(-25.8,9.,134.));
#42148=CARTESIAN_POINT('',(-25.8,0.,135.));
#42149=CARTESIAN_POINT('Origin',(-38.,4.,135.));
#42150=CARTESIAN_POINT('Origin',(-38.,4.8,144.2));
#42151=CARTESIAN_POINT('Origin',(-38.,-9.,135.));
#42152=CARTESIAN_POINT('Origin',(-38.,-4.8,144.2));
#71452=UNCERTAINTY_MEASURE_WITH_UNIT(LENGTH_MEASURE(0.001),#71493,
'DISTANCE_ACCURACY_VALUE',
'Maximum model space distance between geometric entities at asserted c
onnectivities');
#71471=UNCERTAINTY_MEASURE_WITH_UNIT(LENGTH_MEASURE(0.001),#71493,
'DISTANCE_ACCURACY_VALUE',
'Maximum model space distance between geometric entities at asserted c
onnectivities');
#71473=(
GEOMETRIC_REPRESENTATION_CONTEXT(3)
GLOBAL_UNCERTAINTY_ASSIGNED_CONTEXT((#71452))
GLOBAL_UNIT_ASSIGNED_CONTEXT((#71493,#71495,#71496))
REPRESENTATION_CONTEXT('','3D')
);
#71492=(
GEOMETRIC_REPRESENTATION_CONTEXT(3)
GLOBAL_UNCERTAINTY_ASSIGNED_CONTEXT((#71471))
GLOBAL_UNIT_ASSIGNED_CONTEXT((#71493,#71495,#71496))
REPRESENTATION_CONTEXT('','3D')
);
#71493=(
LENGTH_UNIT()
NAMED_UNIT(*)
SI_UNIT(.CENTI.,.METRE.)
);
#71495=(
NAMED_UNIT(*)
PLANE_ANGLE_UNIT()
SI_UNIT($,.RADIAN.)
);
#71496=(
NAMED_UNIT(*)
SI_UNIT($,.STERADIAN.)
SOLID_ANGLE_UNIT()
);
#71498=SHAPE_DEFINITION_REPRESENTATION(#71518,#71603);
#71518=PRODUCT_DEFINITION_SHAPE('',$,#71624);
#71603=SHAPE_REPRESENTATION('',(#28689),#71473);
#71622=PRODUCT_DEFINITION_CONTEXT('part definition',#71684,'design');
#71624=PRODUCT_DEFINITION('2026-10-19-03-21-47-060',
'02_Top_Head_Beam_Twin_RHS100x50x6',#71644,#71622);
#71644=PRODUCT_DEFINITION_FORMATION('',$,#71687);
#71684=APPLICATION_CONTEXT(
'Core Data for Automotive Mechanical Design Process');
#71685=PRODUCT_CONTEXT('part definition',#71684,'mechanical');
#71687=PRODUCT('2026-10-19-03-21-47-060',
'02_Top_Head_Beam_Twin_RHS100x50x6',$,(#71685));
#71867=COLOUR_RGB('Light Blue',0.38,0.62,0.78);
#71868=FILL_AREA_STYLE_COLOUR('',#71867);
#71869=FILL_AREA_STYLE('',(#71868));
#71870=SURFACE_STYLE_FILL_AREA(#71869);
#71871=SURFACE_SIDE_STYLE('',(#71870));
#71872=SURFACE_STYLE_USAGE(.BOTH.,#71871);
#71873=PRESENTATION_STYLE_ASSIGNMENT((#71872));
ENDSEC;
END-ISO-10303-21;
